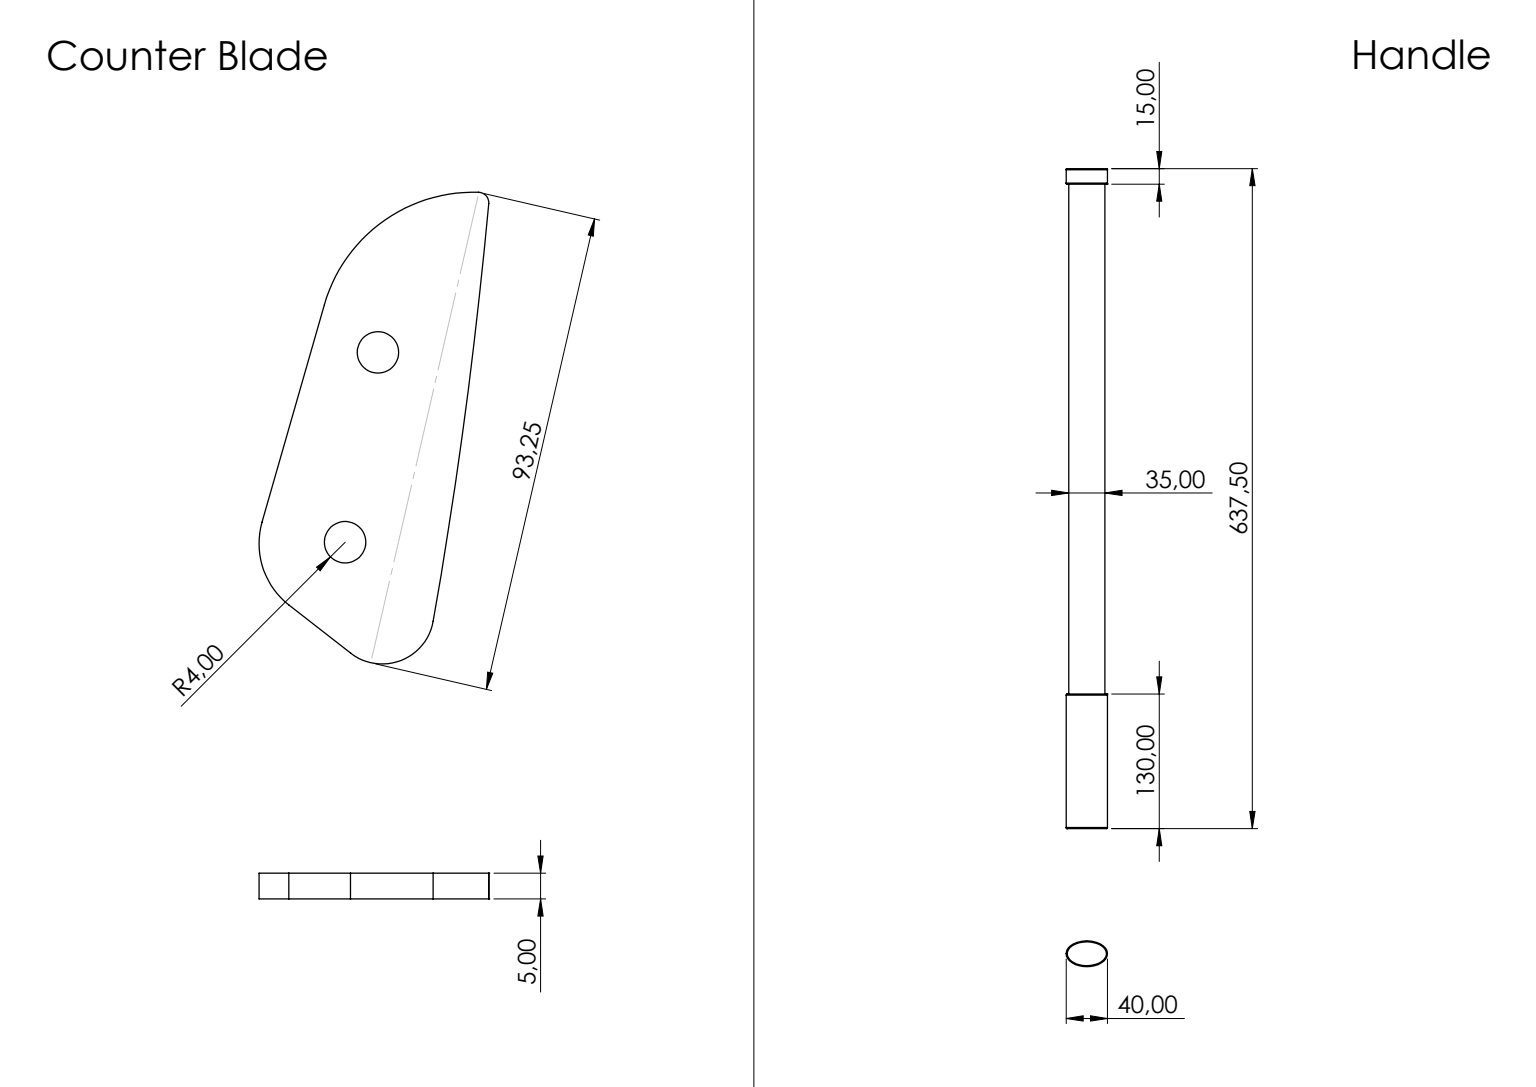
ISO-10303-21;
HEADER;
FILE_DESCRIPTION (('STEP AP214'),
    '1' );
FILE_NAME ('Handle.step',
    '2026-10-06T08:24:18',
    ( '' ),
    ( '' ),
    'SwSTEP 2.0',
    'SolidWorks 2020',
    '' );
FILE_SCHEMA (( 'AUTOMOTIVE_DESIGN' ));
ENDSEC;

DATA;
#4=CARTESIAN_POINT ( 'NONE',  ( 15.24035984457677628, 4.192874667847209302, 315.0000000000000000 ) ) ;
#5=CARTESIAN_POINT ( 'NONE',  ( 9.254661647337838914, -11.09380704494734360, -303.4999999999996589 ) ) ;
#6=CARTESIAN_POINT ( 'NONE',  ( 16.58659719219999928, 2.947707964209000053, -314.6383426456000052 ) ) ;
#11=CARTESIAN_POINT ( 'NONE',  ( 14.97796429264999141, 8.396158284077998246, -317.0792622552969533 ) ) ;
#15=CARTESIAN_POINT ( 'NONE',  ( 4.345375235838000449, -11.20786428128000090, 320.0000000000000000 ) ) ;
#19=CARTESIAN_POINT ( 'NONE',  ( 12.11078853722071180, -6.646648371397081867, -315.0000000000000000 ) ) ;
#22=VERTEX_POINT ( 'NONE', #5856 ) ;
#23=CARTESIAN_POINT ( 'NONE',  ( -16.90341843474000072, 5.241942252742000541, -317.4999999999989768 ) ) ;
#26=CARTESIAN_POINT ( 'NONE',  ( -6.686361683900003072, -11.78513185998999546, -303.6197174156509391 ) ) ;
#28=CARTESIAN_POINT ( 'NONE',  ( 9.022589772749004311, -9.990182113135000819, -317.4928077629770087 ) ) ;
#29=CARTESIAN_POINT ( 'NONE',  ( 10.00000000000000000, 2.500000000000000000, -317.5000000000000000 ) ) ;
#30=EDGE_CURVE ( 'NONE', #1105, #135, #3775, .T. ) ;
#31=CARTESIAN_POINT ( 'NONE',  ( -18.56223039349998771, 4.700611568415998143, -303.6197174156520759 ) ) ;
#32=CARTESIAN_POINT ( 'NONE',  ( -17.50000003227012613, 5.857864393370423528, 314.9999999999999432 ) ) ;
#40=CARTESIAN_POINT ( 'NONE',  ( 16.39637408479998726, -7.274214857915000998, 190.4207385301700128 ) ) ;
#42=CARTESIAN_POINT ( 'NONE',  ( 16.31080841943641602, 2.657385524587721370, -314.9999999999999432 ) ) ;
#45=CARTESIAN_POINT ( 'NONE',  ( 17.36938240862999905, -0.02134527931159000205, 314.6383426456000052 ) ) ;
#50=CARTESIAN_POINT ( 'NONE',  ( 15.30440697208000600, -7.531500302410004011, 320.0770942683900557 ) ) ;
#52=CARTESIAN_POINT ( 'NONE',  ( -19.86889125890001395, 1.746333262808030584, -303.4999999999990905 ) ) ;
#53=CARTESIAN_POINT ( 'NONE',  ( 15.71297435277999810, 3.490404421959999670, 315.0848619657999734 ) ) ;
#55=CARTESIAN_POINT ( 'NONE',  ( 12.16184652991773163, -9.933083713569276441, 190.9999999999995737 ) ) ;
#61=CARTESIAN_POINT ( 'NONE',  ( 15.00000000000000000, 0.000000000000000000, -285.0000000000000000 ) ) ;
#67=ORIENTED_EDGE ( 'NONE', *, *, #7702, .T. ) ;
#68=CARTESIAN_POINT ( 'NONE',  ( -16.87780931964001141, 6.722286650069999148, -316.3802825947000201 ) ) ;
#70=CARTESIAN_POINT ( 'NONE',  ( -13.47907531561000027, -8.083075672345000129, 320.0000000000000000 ) ) ;
#72=DIRECTION ( 'NONE',  ( 2.134661487851416834E-05, 5.799867324353239268E-11, -0.9999999997721611411 ) ) ;
#73=CARTESIAN_POINT ( 'NONE',  ( 2.450863364448387038, -9.399909383054028567, -315.0000000000000000 ) ) ;
#76=CARTESIAN_POINT ( 'NONE',  ( 4.551150791544315233, -9.653623619670588241, -314.5171481538503144 ) ) ;
#79=CARTESIAN_POINT ( 'NONE',  ( 14.32993508528999982, 7.533629911342000440, -317.5000000000000000 ) ) ;
#80=EDGE_LOOP ( 'NONE', ( #2760, #368 ) ) ;
#82=CARTESIAN_POINT ( 'NONE',  ( -17.70828763765000247, -5.833668797872996414, -303.6197174156520759 ) ) ;
#83=CLOSED_SHELL ( 'NONE', ( #10215, #9940, #6869, #5277, #4807 ) ) ;
#84=CARTESIAN_POINT ( 'NONE',  ( 3.630810623869999976, -11.17897874952999793, -317.4928077629770087 ) ) ;
#92=CARTESIAN_POINT ( 'NONE',  ( -10.00000000000000000, 2.500000000000000000, -315.0000000000000000 ) ) ;
#95=CARTESIAN_POINT ( 'NONE',  ( 18.68134283559999531, -4.475435185431997809, 191.1197171614399792 ) ) ;
#99=CARTESIAN_POINT ( 'NONE',  ( -7.781240562249999826, 11.51887802030999985, 191.1197171614399792 ) ) ;
#100=ORIENTED_CLOSED_SHELL ( 'NONE', *, #3850, .F. );
#105=CARTESIAN_POINT ( 'NONE',  ( 18.85102544288001170, -0.8044398135754999846, 319.9928079742500131 ) ) ;
#106=CARTESIAN_POINT ( 'NONE',  ( -9.994972990543319113, 8.217268623422803842, 314.4999428952269227 ) ) ;
#107=CARTESIAN_POINT ( 'NONE',  ( 8.519003879469000395, 8.390442916014999142, 314.8616023057000461 ) ) ;
#109=CARTESIAN_POINT ( 'NONE',  ( 7.783073706837757122, -11.52583533951409756, 190.9999999999995737 ) ) ;
#116=CARTESIAN_POINT ( 'NONE',  ( -3.309867371927075919, 9.320876041153052682, 315.0000000000000568 ) ) ;
#118=EDGE_LOOP ( 'NONE', ( #3514, #10461 ) ) ;
#123=CARTESIAN_POINT ( 'NONE',  ( 0.000000000000000000, 7.937240849781000307, 315.0000000000001705 ) ) ;
#125=CARTESIAN_POINT ( 'NONE',  ( 1.606003227921999343, 12.55439432250999587, -317.0792622552969533 ) ) ;
#130=CARTESIAN_POINT ( 'NONE',  ( 16.45380452100018331, -2.370995337294541372, -315.0000000000000000 ) ) ;
#133=ORIENTED_EDGE ( 'NONE', *, *, #10090, .F. ) ;
#135=VERTEX_POINT ( 'NONE', #4262 ) ;
#136=CARTESIAN_POINT ( 'NONE',  ( 3.426853146664001759, -12.32346385046998627, -303.6197174156509391 ) ) ;
#137=CARTESIAN_POINT ( 'NONE',  ( -10.06352840551000050, -9.619263554820991047, -317.4928077629770087 ) ) ;
#139=CARTESIAN_POINT ( 'NONE',  ( -16.90798586812000082, -0.2930809059028999797, -315.0848619657999734 ) ) ;
#141=CARTESIAN_POINT ( 'NONE',  ( -5.044863629634003921, 12.10215170741999557, -303.6197174156520759 ) ) ;
#142=CARTESIAN_POINT ( 'NONE',  ( -15.42236150774597903, -4.758481132285194981, 314.4999482133869719 ) ) ;
#143=EDGE_LOOP ( 'NONE', ( #5687, #4056 ) ) ;
#145=CARTESIAN_POINT ( 'NONE',  ( -12.36246450207000080, 8.718211867489999989, -302.5000000000000000 ) ) ;
#147=CARTESIAN_POINT ( 'NONE',  ( 17.61637523988000353, -5.923742513492005202, 191.1197171614399792 ) ) ;
#148=CARTESIAN_POINT ( 'NONE',  ( -12.98706127646999953, -6.788989183774999603, -315.0000000000001137 ) ) ;
#149=CARTESIAN_POINT ( 'NONE',  ( 15.88699210612483803, 3.373196549223925533, -315.0000000000000000 ) ) ;
#151=CARTESIAN_POINT ( 'NONE',  ( 13.05089818882000507, 9.570190452814999915, 190.4207385301700128 ) ) ;
#153=CARTESIAN_POINT ( 'NONE',  ( 17.12432750374000179, 0.4000877216259000058, 314.8616023057000461 ) ) ;
#155=CARTESIAN_POINT ( 'NONE',  ( -18.77022956583000735, -3.456581952569002247, 320.0770942683900557 ) ) ;
#156=CARTESIAN_POINT ( 'NONE',  ( -17.50000000000000000, 1.896400240175167841E-08, 314.4999014931028682 ) ) ;
#157=CARTESIAN_POINT ( 'NONE',  ( -19.99979308783253273, 0.5741528085765136291, -303.4999999999998863 ) ) ;
#159=CARTESIAN_POINT ( 'NONE',  ( 14.38384290288000145, 5.252906928686999599, 314.8616023057000461 ) ) ;
#161=CARTESIAN_POINT ( 'NONE',  ( 10.13048420337591615, -10.78707197045944355, 190.9999999999995737 ) ) ;
#163=CARTESIAN_POINT ( 'NONE',  ( -0.6354225718825003977, 12.59144946217000260, 319.5792614743400009 ) ) ;
#166=CARTESIAN_POINT ( 'NONE',  ( -12.75139817577315604, 6.274227700150676768, 315.0000000000000568 ) ) ;
#175=CARTESIAN_POINT ( 'NONE',  ( 11.05300996161902560, -7.762248705067454679, 314.4999426419801694 ) ) ;
#183=CARTESIAN_POINT ( 'NONE',  ( 17.50000000000000000, 0.000000000000000000, -315.0000000000000000 ) ) ;
#185=CARTESIAN_POINT ( 'NONE',  ( 4.714169693051698751, -9.123832451407690058, -315.0000000000000000 ) ) ;
#188=CARTESIAN_POINT ( 'NONE',  ( 13.93637444108895096, -8.981144148067276234, -316.5000000000004547 ) ) ;
#189=VERTEX_POINT ( 'NONE', #1946 ) ;
#190=CARTESIAN_POINT ( 'NONE',  ( -5.180828043054999554, 11.07085478567999992, -317.5000000000000000 ) ) ;
#192=CARTESIAN_POINT ( 'NONE',  ( -5.254364691879999327, -12.06635523715000424, -303.6197174156520759 ) ) ;
#193=CARTESIAN_POINT ( 'NONE',  ( 10.19016500772999656, -9.569509725303996461, -317.4928077629770087 ) ) ;
#196=CARTESIAN_POINT ( 'NONE',  ( -3.426853146664001759, 12.32346385046998627, -303.6197174156509391 ) ) ;
#197=ADVANCED_FACE ( 'NONE', ( #5213 ), #3671, .T. ) ;
#200=CARTESIAN_POINT ( 'NONE',  ( -17.12450099635000100, 0.4005340032738999856, -314.8616023057000461 ) ) ;
#201=CARTESIAN_POINT ( 'NONE',  ( -19.00000000000000000, 0.000000000000000000, -302.5000000001010108 ) ) ;
#203=CARTESIAN_POINT ( 'NONE',  ( -20.05695074155000768, 0.5616361869863997214, 190.4207385301700128 ) ) ;
#205=CARTESIAN_POINT ( 'NONE',  ( 13.92525118639320425, 5.424153755683056133, -315.0000000000000000 ) ) ;
#206=CARTESIAN_POINT ( 'NONE',  ( 18.77789454208001985, 4.479159834667000517, 190.4207385301700128 ) ) ;
#207=CARTESIAN_POINT ( 'NONE',  ( 15.60185585328000002, -4.689707898928999974, 314.4150829855000211 ) ) ;
#210=CARTESIAN_POINT ( 'NONE',  ( 4.335116381453002710, -11.79481621787999757, 320.0770942683900557 ) ) ;
#212=CARTESIAN_POINT ( 'NONE',  ( -5.453155018295565704, 9.512440914238338152, 314.4999437815906731 ) ) ;
#213=CARTESIAN_POINT ( 'NONE',  ( -19.32402384659099326, 3.348155292981251030, -303.4999999999990905 ) ) ;
#214=CARTESIAN_POINT ( 'NONE',  ( 12.10743226551000085, 7.094093637544000686, 314.6383426456000052 ) ) ;
#217=CARTESIAN_POINT ( 'NONE',  ( 4.941041030666997180, 12.20591504665998350, 319.5792614743400009 ) ) ;
#220=CARTESIAN_POINT ( 'NONE',  ( -7.529172669043764365, 8.513076715957524243, 315.0000000000000000 ) ) ;
#227=CARTESIAN_POINT ( 'NONE',  ( -6.280550016735999996, 10.85821747223999978, 190.0000000000000000 ) ) ;
#228=CARTESIAN_POINT ( 'NONE',  ( 17.49966312145292591, -0.4461383165315541688, 314.4999388432775049 ) ) ;
#231=CARTESIAN_POINT ( 'NONE',  ( 10.60393767981000757, 9.400660304482000740, 190.0071920248299477 ) ) ;
#239=CARTESIAN_POINT ( 'NONE',  ( -8.616488358140818704, -8.177789738293625987, -315.0000000000000000 ) ) ;
#242=CARTESIAN_POINT ( 'NONE',  ( -13.89291764776418603, -9.007512922136868383, -316.5000000000004547 ) ) ;
#245=VERTEX_POINT ( 'NONE', #4539 ) ;
#246=CARTESIAN_POINT ( 'NONE',  ( -17.62591998684001027, 4.093640041088997705, -317.4928077629770087 ) ) ;
#247=CARTESIAN_POINT ( 'NONE',  ( 19.46922894822000316, -1.611824300579999925, -317.5770954168139610 ) ) ;
#249=CARTESIAN_POINT ( 'NONE',  ( -16.41165915566000066, 2.800979832323999830, -314.8616023057000461 ) ) ;
#258=CARTESIAN_POINT ( 'NONE',  ( -7.580171359958006505, -11.65906041016999062, 190.4207385301700128 ) ) ;
#260=CARTESIAN_POINT ( 'NONE',  ( 16.10169247195999631, -5.923112460043001626, -302.5071922382879279 ) ) ;
#261=CARTESIAN_POINT ( 'NONE',  ( -15.61478958302000208, 7.813810907915007320, 191.1197171614399792 ) ) ;
#263=CARTESIAN_POINT ( 'NONE',  ( 13.50042001888999899, -6.225262767767000049, 314.6383426456000052 ) ) ;
#264=DIRECTION ( 'NONE',  ( -1.023612789531999991E-09, -6.047396539087999167E-11, 1.000000000000000000 ) ) ;
#265=CARTESIAN_POINT ( 'NONE',  ( 2.578726422179000721, -12.49238522902999726, 319.5792614743400009 ) ) ;
#267=CARTESIAN_POINT ( 'NONE',  ( -16.88587703871184686, 6.724495681871323960, -303.4999999999990905 ) ) ;
#268=CARTESIAN_POINT ( 'NONE',  ( 16.95904175860000151, 2.156867278632000229, 314.6383426456000052 ) ) ;
#270=CARTESIAN_POINT ( 'NONE',  ( 13.10504385913262482, -9.452822371482909602, 190.9999999999995737 ) ) ;
#271=CARTESIAN_POINT ( 'NONE',  ( 6.490016473005998598, 11.91548699335000272, 319.5792614743400009 ) ) ;
#272=DIRECTION ( 'NONE',  ( 5.580921735165581358E-06, -2.007400791704409772E-12, 0.9999999999844266796 ) ) ;
#273=CARTESIAN_POINT ( 'NONE',  ( 4.934712326437797003, 9.087261561615623151, 315.0000000000000000 ) ) ;
#277=CARTESIAN_POINT ( 'NONE',  ( 2.585384220735000405, 11.41066401029999966, 190.0000000000000000 ) ) ;
#278=CARTESIAN_POINT ( 'NONE',  ( -14.02804746531204749, 5.341076607092833051, -315.0000000000000000 ) ) ;
#284=LINE ( 'NONE', #8342, #7202 ) ;
#288=CARTESIAN_POINT ( 'NONE',  ( 5.323201728285183343, -12.06184864676790447, -316.5000000000004547 ) ) ;
#291=ORIENTED_EDGE ( 'NONE', *, *, #4224, .T. ) ;
#292=DIRECTION ( 'NONE',  ( -2.558226603731915840E-07, 0.9999999999999674705, 3.930810334569221757E-22 ) ) ;
#294=CARTESIAN_POINT ( 'NONE',  ( -19.60172830838999047, -0.3498260303709999630, -317.5770954168139610 ) ) ;
#296=CARTESIAN_POINT ( 'NONE',  ( -17.56758064089999749, 0.6313722887073000001, -314.4150829855000211 ) ) ;
#297=( BOUNDED_CURVE ( )  B_SPLINE_CURVE ( 3, ( #701, #648, #8167, #4939 ),
 .UNSPECIFIED., .F., .F. ) 
 B_SPLINE_CURVE_WITH_KNOTS ( ( 4, 4 ),
 ( 0.000000000000000000, 0.9999999989866708017 ),
 .UNSPECIFIED. ) 
 CURVE ( )  GEOMETRIC_REPRESENTATION_ITEM ( )  RATIONAL_B_SPLINE_CURVE ( ( 1.000000000000000000, 0.8029010327867776020, 0.8003084355100938962, 0.9922222081699485496 ) ) 
 REPRESENTATION_ITEM ( '' )  );
#299=CARTESIAN_POINT ( 'NONE',  ( 17.59656075795390606, 5.807225057570236437, 315.0000000000000000 ) ) ;
#300=ORIENTED_EDGE ( 'NONE', *, *, #1909, .T. ) ;
#301=CARTESIAN_POINT ( 'NONE',  ( -17.35547125580999861, -4.661453509011000307, 190.0000000000000000 ) ) ;
#307=CARTESIAN_POINT ( 'NONE',  ( -10.00000000000000000, 2.500000000000000000, -285.0000000000000000 ) ) ;
#310=CARTESIAN_POINT ( 'NONE',  ( 7.580171359958006505, 11.65906041016999062, 190.4207385301700128 ) ) ;
#314=CARTESIAN_POINT ( 'NONE',  ( -18.87180507196998747, -0.3567823988189002815, -302.5071922382879279 ) ) ;
#315=CARTESIAN_POINT ( 'NONE',  ( -19.98292278601002181, 0.4165571180016003350, 318.8802828394900644 ) ) ;
#317=CARTESIAN_POINT ( 'NONE',  ( 17.13090252310000139, 0.3058267005333999977, -314.8616023057000461 ) ) ;
#319=CARTESIAN_POINT ( 'NONE',  ( -14.57772014836000096, 5.380605385836000565, 314.6383426456000052 ) ) ;
#321=CARTESIAN_POINT ( 'NONE',  ( 14.19899178590998190, -7.472503199908998361, 190.0071920248299477 ) ) ;
#323=CARTESIAN_POINT ( 'NONE',  ( 1.330908921489000418, 12.56946842516999041, 319.5792614743400009 ) ) ;
#325=CARTESIAN_POINT ( 'NONE',  ( 9.142607798242581296, 7.997258514545670494, 315.0000000000000000 ) ) ;
#330=CARTESIAN_POINT ( 'NONE',  ( 13.37693598625000213, 8.145668871592000926, 190.0000000000000000 ) ) ;
#331=CARTESIAN_POINT ( 'NONE',  ( 13.64750606492133045, -6.290789845814279246, 314.4999418822395114 ) ) ;
#332=CARTESIAN_POINT ( 'NONE',  ( -15.60334176867001688, 6.376785739494004623, 190.0071920248299477 ) ) ;
#337=CARTESIAN_POINT ( 'NONE',  ( 14.25090727152774228, -5.161646102170217354, 315.0000000000000568 ) ) ;
#340=CARTESIAN_POINT ( 'NONE',  ( 3.092734256763002065, 11.24153629139000188, 319.9928079742500131 ) ) ;
#341=CARTESIAN_POINT ( 'NONE',  ( -16.85039254115126539, -6.759165854037040511, -316.5000000000004547 ) ) ;
#347=CARTESIAN_POINT ( 'NONE',  ( -14.69255688194000520, -7.987735679832996816, -317.5770954168139610 ) ) ;
#348=CARTESIAN_POINT ( 'NONE',  ( -15.92197846796999983, 3.582977715798000062, -314.8616023057000461 ) ) ;
#349=CARTESIAN_POINT ( 'NONE',  ( 17.27223423031419358, 1.573973318776797026, -314.5135302205612220 ) ) ;
#350=ORIENTED_EDGE ( 'NONE', *, *, #8269, .F. ) ;
#361=ADVANCED_FACE ( 'NONE', ( #10562 ), #4708, .F. ) ;
#364=FACE_OUTER_BOUND ( 'NONE', #2969, .T. ) ;
#365=CARTESIAN_POINT ( 'NONE',  ( 19.56939737065003015, -2.860667089442002986, 319.5792614743400009 ) ) ;
#367=CARTESIAN_POINT ( 'NONE',  ( -14.43094748301999886, 5.211771040651000497, 314.8616023057000461 ) ) ;
#368=ORIENTED_EDGE ( 'NONE', *, *, #5471, .T. ) ;
#370=ORIENTED_EDGE ( 'NONE', *, *, #7787, .T. ) ;
#371=CARTESIAN_POINT ( 'NONE',  ( -17.61140045117998554, 5.929979699424000827, 318.8802828394900644 ) ) ;
#374=CARTESIAN_POINT ( 'NONE',  ( -17.13182678275000370, 0.2945984483948000388, 314.8616023057000461 ) ) ;
#375=CARTESIAN_POINT ( 'NONE',  ( -15.88661950543927404, 3.373766516133892335, 315.0000000000000000 ) ) ;
#383=CARTESIAN_POINT ( 'NONE',  ( -8.676965067697993916, 10.10010313590999509, 190.0071920248299477 ) ) ;
#387=CARTESIAN_POINT ( 'NONE',  ( 8.517242506840645433, -8.210459489885888473, 315.0000000000000568 ) ) ;
#388=CARTESIAN_POINT ( 'NONE',  ( 11.99990625867999938, 6.898016740823000426, -314.8616023057000461 ) ) ;
#391=CARTESIAN_POINT ( 'NONE',  ( 10.79243608611000305, 9.321647281761997306, 319.9928079742500131 ) ) ;
#395=CARTESIAN_POINT ( 'NONE',  ( -15.97383562432999149, -7.643564190274003245, -317.0792622552969533 ) ) ;
#399=CARTESIAN_POINT ( 'NONE',  ( 12.62255196312000116, -8.576358104672999971, 190.0000000000000000 ) ) ;
#402=CARTESIAN_POINT ( 'NONE',  ( -15.59929043073998578, -7.826471063572999931, 191.1197171614399792 ) ) ;
#405=CARTESIAN_POINT ( 'NONE',  ( -1.914578617915998704, -11.33709939001001032, -302.5071922382879279 ) ) ;
#411=CARTESIAN_POINT ( 'NONE',  ( -13.35956122709998795, 8.020600178289003068, -302.5071922382879279 ) ) ;
#412=CARTESIAN_POINT ( 'NONE',  ( -19.58476356052999279, -2.818858455686998887, 319.5792614743400009 ) ) ;
#413=CARTESIAN_POINT ( 'NONE',  ( 16.99702983282000091, -1.298346578676000007, -314.8616023057000461 ) ) ;
#414=AXIS2_PLACEMENT_3D ( 'NONE', #9424, #292, #2763 ) ;
#415=CARTESIAN_POINT ( 'NONE',  ( -12.17979804859000126, 7.053762231097000068, 314.6383426456000052 ) ) ;
#417=CARTESIAN_POINT ( 'NONE',  ( -9.595833218033995138, -9.789665514059997520, 190.0071920248299477 ) ) ;
#423=CARTESIAN_POINT ( 'NONE',  ( -17.35477687787999912, 0.3068793820639000303, 314.6383426456000052 ) ) ;
#424=CARTESIAN_POINT ( 'NONE',  ( -16.34899991413091414, 2.583752171356570759, 315.0000000000000000 ) ) ;
#427=AXIS2_PLACEMENT_3D ( 'NONE', #92, #1648, #838 ) ;
#428=CARTESIAN_POINT ( 'NONE',  ( -16.31080841943642312, -2.657385524587722703, -315.0000000000001137 ) ) ;
#431=CARTESIAN_POINT ( 'NONE',  ( 11.71572875054933327, 12.50000000135959688, -303.5000000000000000 ) ) ;
#433=CARTESIAN_POINT ( 'NONE',  ( 8.586696445213114259, 8.187646113561793726, -314.9999999999999432 ) ) ;
#434=CARTESIAN_POINT ( 'NONE',  ( 17.75414941409001557, 3.856242593410000197, 190.0071920248299477 ) ) ;
#436=CARTESIAN_POINT ( 'NONE',  ( 17.50000000000000711, -8.653864165198663120E-10, -302.4999999999999432 ) ) ;
#439=CARTESIAN_POINT ( 'NONE',  ( -11.26076953950000004, -9.251451169536998975, -317.5000000000000000 ) ) ;
#442=CARTESIAN_POINT ( 'NONE',  ( 2.737672117484407863, -9.377292971636139285, 315.0000000000000568 ) ) ;
#443=CARTESIAN_POINT ( 'NONE',  ( 13.18712987686000027, 5.898505050745000311, -315.0848619657999734 ) ) ;
#445=CARTESIAN_POINT ( 'NONE',  ( 18.45919443845001950, 2.405475664342000996, 319.9928079742500131 ) ) ;
#448=ORIENTED_EDGE ( 'NONE', *, *, #9438, .T. ) ;
#450=CARTESIAN_POINT ( 'NONE',  ( 19.39427072114999717, -3.381181012882998882, -317.0792622552969533 ) ) ;
#452=B_SPLINE_CURVE_WITH_KNOTS ( 'NONE', 3,
 ( #9871, #3367, #5940, #9919, #5772, #2557, #9228, #142, #5825, #942, #10323, #1912, #8408, #5184, #1349, #10377, #4385, #5129, #7659, #8654, #4578, #3528 ),
 .UNSPECIFIED., .F., .F.,
 ( 4, 2, 2, 2, 2, 2, 2, 2, 2, 2, 4 ),
 ( 0.000000000000000000, 0.06249979490446620767, 0.1249995898089324153, 0.1874993847133986091, 0.2499991796178648307, 0.3124989745223310522, 0.3437488719745641630, 0.3749987694267972183, 0.4062486668790303290, 0.4374985643312634398, 0.4999983592357296613 ),
 .UNSPECIFIED. ) ;
#453=ADVANCED_BREP_SHAPE_REPRESENTATION ( '', ( #5170, #2817 ), #8168 ) ;
#455=ORIENTED_EDGE ( 'NONE', *, *, #1550, .F. ) ;
#456=CARTESIAN_POINT ( 'NONE',  ( -14.18540515794000001, -7.627402598852000004, 190.0000000000000000 ) ) ;
#458=ORIENTED_EDGE ( 'NONE', *, *, #4238, .T. ) ;
#459=CARTESIAN_POINT ( 'NONE',  ( 10.12800840543000724, -10.78031690431999756, 191.1197171614399792 ) ) ;
#461=CARTESIAN_POINT ( 'NONE',  ( -16.68818136459866253, -1.819152193222137281, 315.0000000000000000 ) ) ;
#462=CARTESIAN_POINT ( 'NONE',  ( 13.35956122709998795, -8.020600178289003068, -302.5071922382879279 ) ) ;
#466=CARTESIAN_POINT ( 'NONE',  ( 6.445894847559003438, 10.69844988487999693, -302.5071922382879279 ) ) ;
#468=CARTESIAN_POINT ( 'NONE',  ( -16.43550475785002263, -7.239471399781003846, 319.5792614743400009 ) ) ;
#469=CARTESIAN_POINT ( 'NONE',  ( 15.92197846796999983, -3.582977715798000062, -314.8616023057000461 ) ) ;
#470=CARTESIAN_POINT ( 'NONE',  ( -13.62823431091000081, 6.408810695481999886, 314.4150829855000211 ) ) ;
#472=CARTESIAN_POINT ( 'NONE',  ( 17.73236801841998300, -3.892024484092002634, 190.0071920248299477 ) ) ;
#482=CARTESIAN_POINT ( 'NONE',  ( -16.61594764501906596, 2.013242305049250280, 315.0000000000001137 ) ) ;
#484=CARTESIAN_POINT ( 'NONE',  ( -10.90988923471838667, -7.272053090123304031, -315.0000000000000568 ) ) ;
#487=CARTESIAN_POINT ( 'NONE',  ( 17.50000000088855501, 5.867334121986936601, -302.4999999999996589 ) ) ;
#488=CARTESIAN_POINT ( 'NONE',  ( 0.9838506439437809670, 9.488399989288442526, -314.9999999999998863 ) ) ;
#489=CARTESIAN_POINT ( 'NONE',  ( -19.54676335584001023, 0.8901129224502002391, 189.9229057364800042 ) ) ;
#490=CARTESIAN_POINT ( 'NONE',  ( 11.54127216423516877, 7.525448809341461320, 314.4999468205385824 ) ) ;
#496=CARTESIAN_POINT ( 'NONE',  ( 9.217211940708146756, -7.977736869146946574, 315.0000000000000000 ) ) ;
#497=CARTESIAN_POINT ( 'NONE',  ( -8.551447359560999217, 8.144527334518999240, -315.0848619657999734 ) ) ;
#499=CARTESIAN_POINT ( 'NONE',  ( -18.12318599310000167, 3.186119256560000945, 319.9928079742500131 ) ) ;
#503=CARTESIAN_POINT ( 'NONE',  ( -18.21319838702001448, 4.476589323548002319, -317.5770954168139610 ) ) ;
#504=CARTESIAN_POINT ( 'NONE',  ( -11.69962851017000283, -10.23591410519999201, -317.0792622552969533 ) ) ;
#508=CARTESIAN_POINT ( 'NONE',  ( -17.50000000000000000, 0.000000000000000000, -315.0000000000000000 ) ) ;
#510=CARTESIAN_POINT ( 'NONE',  ( -12.62255196312000116, 8.576358104672999971, 190.0000000000000000 ) ) ;
#513=DIRECTION ( 'NONE',  ( 0.000000000000000000, 0.000000000000000000, 1.000000000000000000 ) ) ;
#515=CARTESIAN_POINT ( 'NONE',  ( -19.78498824058000594, -1.878712957033002340, 191.1197171614399792 ) ) ;
#518=CARTESIAN_POINT ( 'NONE',  ( 10.36918760129999484, -10.25095399663999451, -302.4229045757450081 ) ) ;
#523=CARTESIAN_POINT ( 'NONE',  ( -6.297776810737998332, 10.73166643879000404, -302.5071922382879279 ) ) ;
#525=CARTESIAN_POINT ( 'NONE',  ( -17.14577796628000073, 0.02050488658304999712, 314.8616023057000461 ) ) ;
#528=CARTESIAN_POINT ( 'NONE',  ( -16.98888588455999127, 6.600739700975996271, 318.8802828394900644 ) ) ;
#530=DIRECTION ( 'NONE',  ( 0.000000000000000000, 0.000000000000000000, 1.000000000000000000 ) ) ;
#534=CARTESIAN_POINT ( 'NONE',  ( 11.28781796570999951, -4.951468039558000633, 315.0000000000001705 ) ) ;
#535=CARTESIAN_POINT ( 'NONE',  ( -13.94567317170587017, -5.407789506212602682, -314.9999999999999432 ) ) ;
#538=CARTESIAN_POINT ( 'NONE',  ( -10.23467949692583190, 10.00000000050611959, -302.5000000000002842 ) ) ;
#539=CARTESIAN_POINT ( 'NONE',  ( 8.377487131979357571, 8.255758461348163380, -315.0000000000000000 ) ) ;
#540=CARTESIAN_POINT ( 'NONE',  ( -20.05687582562997662, -0.5621360437329007143, 190.4207385301700128 ) ) ;
#542=CARTESIAN_POINT ( 'NONE',  ( 9.038557733644999814, -10.11114377999000169, -317.5000000000000000 ) ) ;
#545=CARTESIAN_POINT ( 'NONE',  ( 13.92506561308973545, -5.424300063451886089, 315.0000000000000568 ) ) ;
#546=CARTESIAN_POINT ( 'NONE',  ( -6.488017178959999853, 9.182784307579000327, -314.6383426456000052 ) ) ;
#547=FACE_OUTER_BOUND ( 'NONE', #6635, .T. ) ;
#548=CARTESIAN_POINT ( 'NONE',  ( 17.87038977196999312, 4.940238929760003117, 320.0770942683900557 ) ) ;
#552=CARTESIAN_POINT ( 'NONE',  ( -20.10152810630999554, 0.3450717431897997733, -317.0792622552969533 ) ) ;
#553=CARTESIAN_POINT ( 'NONE',  ( -7.863726017345004315, -11.49810175465000661, -316.3802825947000201 ) ) ;
#558=CARTESIAN_POINT ( 'NONE',  ( -4.551150791544325003, 9.653623619670586464, -314.5171481538502576 ) ) ;
#561=CARTESIAN_POINT ( 'NONE',  ( -17.80781204382000027, 3.997739559166000323, 190.0000000000000000 ) ) ;
#562=CARTESIAN_POINT ( 'NONE',  ( 15.56166711177641204, -7.864757419948091410, 319.0000000000003979 ) ) ;
#563=VERTEX_POINT ( 'NONE', #7338 ) ;
#566=CARTESIAN_POINT ( 'NONE',  ( -4.780298404687055580, -9.113031460416761931, 315.0000000000000000 ) ) ;
#567=CARTESIAN_POINT ( 'NONE',  ( -16.90094380520001849, -6.817658119454999444, -302.9207377450070453 ) ) ;
#572=CARTESIAN_POINT ( 'NONE',  ( -9.124390749379998056, 10.69353917616999539, -302.4229045757450081 ) ) ;
#573=CARTESIAN_POINT ( 'NONE',  ( 17.61140045117998554, -5.929979699424000827, 318.8802828394900644 ) ) ;
#575=CARTESIAN_POINT ( 'NONE',  ( -13.56771446467999986, -6.451120369226999607, -314.4150829855000211 ) ) ;
#576=LINE ( 'NONE', #10569, #3520 ) ;
#577=ORIENTED_EDGE ( 'NONE', *, *, #8567, .T. ) ;
#578=CARTESIAN_POINT ( 'NONE',  ( -0.7033324871772000941, -12.09174782753000166, 189.9229057364800042 ) ) ;
#579=CARTESIAN_POINT ( 'NONE',  ( -19.77468550638000266, 1.920668048511998904, 318.8802828394900644 ) ) ;
#584=CARTESIAN_POINT ( 'NONE',  ( -13.31399140613000043, -6.082710156904999721, 314.8616023057000461 ) ) ;
#586=CARTESIAN_POINT ( 'NONE',  ( -13.82226565756009684, 5.505830577453552088, 315.0000000000000568 ) ) ;
#587=FACE_OUTER_BOUND ( 'NONE', #4840, .T. ) ;
#589=CARTESIAN_POINT ( 'NONE',  ( -3.970004819630974957, -9.235895690467337715, -315.0000000000000568 ) ) ;
#590=CARTESIAN_POINT ( 'NONE',  ( 19.99999035944999903, -7.277437094418000096E-10, -303.5000000000000000 ) ) ;
#591=CARTESIAN_POINT ( 'NONE',  ( -11.28781796570999951, 4.951468039558000633, 315.0000000000000000 ) ) ;
#596=CARTESIAN_POINT ( 'NONE',  ( -4.780493465650554441, 9.113006550021843566, -314.9999999999999432 ) ) ;
#598=CARTESIAN_POINT ( 'NONE',  ( 16.06942734036999454, 6.898991720969999797, 189.9229057364800042 ) ) ;
#599=CARTESIAN_POINT ( 'NONE',  ( 17.50000000088856567, 5.867334121986925055, 190.0000000000002558 ) ) ;
#600=CARTESIAN_POINT ( 'NONE',  ( -17.62191473184000046, -4.312542294520999242, -317.5000000000030127 ) ) ;
#604=FACE_BOUND ( 'NONE', #4756, .T. ) ;
#607=CARTESIAN_POINT ( 'NONE',  ( 17.57772697299999720, -0.3191603157329999663, -314.4150829855000211 ) ) ;
#609=CARTESIAN_POINT ( 'NONE',  ( -11.81011838702999484, 9.634252844421009598, 320.0770942683900557 ) ) ;
#613=CARTESIAN_POINT ( 'NONE',  ( -19.56985579239002959, -0.3946094453810997660, -317.5770954168139610 ) ) ;
#614=CARTESIAN_POINT ( 'NONE',  ( 11.75551710966999153, -10.11738730586000123, -316.3802825947000201 ) ) ;
#619=CARTESIAN_POINT ( 'NONE',  ( 19.99999721132999753, -3.518697978483000342E-10, 319.0000000000000000 ) ) ;
#623=CARTESIAN_POINT ( 'NONE',  ( -15.47214269673303200, -3.911151857093433382, 315.0000000000000568 ) ) ;
#624=CARTESIAN_POINT ( 'NONE',  ( -19.95002954278003315, -1.762942793154997911, -302.9207377450070453 ) ) ;
#625=CARTESIAN_POINT ( 'NONE',  ( 10.00000000000000000, 2.500000000000000000, -315.0000000000000000 ) ) ;
#627=ADVANCED_FACE ( 'NONE', ( #9915 ), #6187, .T. ) ;
#628=CARTESIAN_POINT ( 'NONE',  ( 5.268482393219001025, 12.14948647186998976, -302.9207377450070453 ) ) ;
#631=CARTESIAN_POINT ( 'NONE',  ( 10.58688533405000065, -7.844683714540999553, -314.6383426456000052 ) ) ;
#632=CARTESIAN_POINT ( 'NONE',  ( -17.13090252310000139, -0.3058267005333999977, 314.8616023057000461 ) ) ;
#633=ORIENTED_EDGE ( 'NONE', *, *, #4237, .T. ) ;
#634=CARTESIAN_POINT ( 'NONE',  ( 1.232798796115999851, -12.07489154382001040, 189.9229057364800042 ) ) ;
#635=CARTESIAN_POINT ( 'NONE',  ( 9.974269275089660880, 10.84391064191637000, 190.9999999999996589 ) ) ;
#639=CARTESIAN_POINT ( 'NONE',  ( -12.21495827233999876, -7.290170534263999969, 314.4150829855000211 ) ) ;
#642=CARTESIAN_POINT ( 'NONE',  ( 11.73784133842000088, 9.026952533543999735, 320.0000000000000000 ) ) ;
#643=CARTESIAN_POINT ( 'NONE',  ( -1.281333103385001726, -11.37293729856000368, 319.9928079742500131 ) ) ;
#644=CARTESIAN_POINT ( 'NONE',  ( 12.21612826667444729, 9.907025583609536667, 319.0000000000005116 ) ) ;
#645=CARTESIAN_POINT ( 'NONE',  ( -17.50000000000000711, 8.653861160270983887E-10, 190.0000000000000568 ) ) ;
#648=CARTESIAN_POINT ( 'NONE',  ( 10.23467948564923091, 9.999999999493891067, 190.0000000000002558 ) ) ;
#649=CARTESIAN_POINT ( 'NONE',  ( -17.84297720825001221, 4.977647671642006166, 189.9229057364800042 ) ) ;
#651=B_SPLINE_CURVE_WITH_KNOTS ( 'NONE', 3,
 ( #7741, #9568, #4623, #10319, #2960, #6230, #7896, #8699, #10222, #6077, #2857, #6178, #9366, #542, #3819, #7103, #2907, #8589, #9413, #4463, #5316, #9516, #1237, #2157, #10370, #2207, #9462, #439, #8754, #1397, #2102, #1293, #4680, #4513, #600, #6895, #2001, #7793, #5265 ),
 .UNSPECIFIED., .F., .F.,
 ( 4, 1, 1, 1, 1, 1, 1, 1, 1, 1, 1, 1, 1, 1, 1, 1, 1, 1, 1, 1, 1, 1, 1, 1, 1, 1, 1, 1, 1, 1, 1, 1, 1, 1, 1, 1, 4 ),
 ( 0.000000000000000000, 0.02777777777778000015, 0.05555555555556000030, 0.08333333333333001192, 0.1111111111111000027, 0.1388888888888999973, 0.1666666666667000196, 0.1944444444444000109, 0.2222222222222000054, 0.2500000000000000000, 0.2777777777777999946, 0.3055555555555999891, 0.3333333333333000081, 0.3611111111111000027, 0.3888888888888999973, 0.4166666666666999919, 0.4444444444444000109, 0.4722222222222000054, 0.5000000000000000000, 0.5277777777777999946, 0.5555555555555999891, 0.5833333333333000637, 0.6111111111111000582, 0.6388888888888999418, 0.6666666666667000474, 0.6944444444444000109, 0.7222222222222000054, 0.7500000000000000000, 0.7777777777777999946, 0.8055555555555999891, 0.8333333333333000637, 0.8611111111111000582, 0.8888888888888999418, 0.9166666666667000474, 0.9444444444444000109, 0.9722222222222000054, 1.000000000000000000 ),
 .UNSPECIFIED. ) ;
#653=FACE_OUTER_BOUND ( 'NONE', #7217, .T. ) ;
#654=CARTESIAN_POINT ( 'NONE',  ( 11.77008734995756178, 6.834641529527616832, 315.0000000000000568 ) ) ;
#659=CARTESIAN_POINT ( 'NONE',  ( -18.86319819242002183, -0.4765179085981003926, 319.9928079742500131 ) ) ;
#662=CARTESIAN_POINT ( 'NONE',  ( -6.769722431736004076, 11.85293133419998846, -317.0792622552969533 ) ) ;
#663=CARTESIAN_POINT ( 'NONE',  ( 3.762811461229003562, -12.28417267642999278, -316.3802825947000201 ) ) ;
#666=B_SPLINE_CURVE_WITH_KNOTS ( 'NONE', 3,
 ( #4430, #5384, #5329, #349, #4384, #10335, #8456, #2766, #4475, #7755, #9429, #3676, #8664, #1097, #6963, #10237, #6038, #9328, #1964, #6909, #2873, #8605, #1251, #3728, #10285, #2924, #558, #4860, #7225, #8886, #8939, #7169, #3079, #8832, #8715, #9530, #2388, #2224, #7331, #10439, #4055, #7912, #5493, #3890, #2170, #9748 ),
 .UNSPECIFIED., .F., .F.,
 ( 4, 2, 2, 2, 2, 2, 2, 2, 2, 2, 2, 2, 2, 2, 2, 2, 2, 2, 2, 2, 2, 2, 4 ),
 ( 0.000000000000000000, 0.001362852592701295929, 0.002044278889051944111, 0.002725705185402593159, 0.004088557778103887354, 0.005451410370805182849, 0.006814262963506478345, 0.008177115556207774708, 0.01090282074161036743, 0.01635423111241555982, 0.01907993629781816122, 0.02180564148322075915, 0.02453134666862336055, 0.02725705185402596195, 0.02998275703942856335, 0.03270846222483116128, 0.03543416741023376615, 0.03815987259563636408, 0.03952272518833765264, 0.04088557778103895507, 0.04224843037374024363, 0.04292985667009089484, 0.04361128296644153912 ),
 .UNSPECIFIED. ) ;
#669=CARTESIAN_POINT ( 'NONE',  ( 16.99996037728000076, -1.352915083302999933E-09, -314.9999801883000146 ) ) ;
#672=CARTESIAN_POINT ( 'NONE',  ( 10.97430844189483423, -10.45950866754415820, 319.0000000000003979 ) ) ;
#674=CARTESIAN_POINT ( 'NONE',  ( 13.89291764776418603, 9.007512922137015821, -316.5000000000004547 ) ) ;
#675=ORIENTED_EDGE ( 'NONE', *, *, #9162, .F. ) ;
#676=CARTESIAN_POINT ( 'NONE',  ( -5.241997271368903810, -9.033710068163633977, 315.0000000000000000 ) ) ;
#677=CARTESIAN_POINT ( 'NONE',  ( -20.06799914428001941, 0.4075895895062001673, -302.9207377450070453 ) ) ;
#683=CARTESIAN_POINT ( 'NONE',  ( -5.058393412147005108, 12.18538300202998315, -302.9207377450070453 ) ) ;
#684=CARTESIAN_POINT ( 'NONE',  ( -12.21300849950000433, -9.900542285453001412, 318.8802828394900644 ) ) ;
#686=CARTESIAN_POINT ( 'NONE',  ( 13.62823431091000081, -6.408810695481999886, -314.4150829855000211 ) ) ;
#689=CARTESIAN_POINT ( 'NONE',  ( 16.06649953495000105, -6.900914778667005756, 189.9229057364800042 ) ) ;
#690=CARTESIAN_POINT ( 'NONE',  ( -13.10504385913262837, 9.452822371482907826, 190.9999999999996589 ) ) ;
#695=CARTESIAN_POINT ( 'NONE',  ( 1.388768300183999882, -9.421618921053999784, 315.0848619657999734 ) ) ;
#701=CARTESIAN_POINT ( 'NONE',  ( 1.279515965483999906E-07, 10.00000000755999885, 190.0000000000000000 ) ) ;
#702=CARTESIAN_POINT ( 'NONE',  ( -4.791123986588002204, 11.72534684832999119, 189.9229057364800042 ) ) ;
#706=( BOUNDED_SURFACE ( )  B_SPLINE_SURFACE ( 3, 1, ( 
 ( #9973, #6695 ),
 ( #7344, #9011 ),
 ( #5876, #1646 ),
 ( #9168, #7446 ),
 ( #32, #10026 ),
 ( #2508, #6588 ),
 ( #4922, #8198 ) ),
 .UNSPECIFIED., .F., .F., .F. ) 
 B_SPLINE_SURFACE_WITH_KNOTS ( ( 4, 3, 4 ),
 ( 2, 2 ),
 ( 0.000000000000000000, 0.5000000000000000000, 1.000000000000000000 ),
 ( 0.000000000000000000, 1.000000000000000000 ),
 .UNSPECIFIED. ) 
 GEOMETRIC_REPRESENTATION_ITEM ( )  RATIONAL_B_SPLINE_SURFACE ( (
 ( 1.000000000000000000, 1.000000000000000000),
 ( 0.8047378516590519837, 0.8047378516590519837),
 ( 0.8047378516590519837, 0.8047378516590519837),
 ( 1.000000000000000000, 1.000000000000000000),
 ( 0.8047378516590519837, 0.8047378516590519837),
 ( 0.8047378516590519837, 0.8047378516590519837),
 ( 1.000000000000000000, 1.000000000000000000) ) ) 
 REPRESENTATION_ITEM ( '' )  SURFACE ( )  );
#707=CARTESIAN_POINT ( 'NONE',  ( 17.49999999954662044, -9.625715914672042649E-06, 190.0000000000000000 ) ) ;
#710=CARTESIAN_POINT ( 'NONE',  ( 16.98808798087999961, 1.334629195702000004, -314.8616023057000461 ) ) ;
#712=CARTESIAN_POINT ( 'NONE',  ( -19.37251270682998694, 1.820313540576997680, 320.0770942683900557 ) ) ;
#716=CARTESIAN_POINT ( 'NONE',  ( 18.19038122738000141, 4.511441183124001775, -317.5770954168139610 ) ) ;
#717=CARTESIAN_POINT ( 'NONE',  ( 18.56065892533998962, -4.703159488203003669, -316.3802825947000201 ) ) ;
#718=CARTESIAN_POINT ( 'NONE',  ( -18.53598399141000286, -2.541378258162000137, 320.0000000000000000 ) ) ;
#719=AXIS2_PLACEMENT_3D ( 'NONE', #5470, #4675, #10264 ) ;
#721=CARTESIAN_POINT ( 'NONE',  ( 16.53772850381890791, -2.187491735906823997, -314.9999999999998863 ) ) ;
#725=CARTESIAN_POINT ( 'NONE',  ( 15.92495094281444601, 7.583842622554345603, -316.5000000000004547 ) ) ;
#727=( BOUNDED_CURVE ( )  B_SPLINE_CURVE ( 3, ( #4537, #2178, #9337, #3788, #7716, #7022, #2073 ),
 .UNSPECIFIED., .F., .T. ) 
 B_SPLINE_CURVE_WITH_KNOTS ( ( 4, 3, 4 ),
 ( 0.006576891565977574343, 0.5000000000000000000, 0.9934231084340225948 ),
 .UNSPECIFIED. ) 
 CURVE ( )  GEOMETRIC_REPRESENTATION_ITEM ( )  RATIONAL_B_SPLINE_CURVE ( ( 0.9922222087809801083, 0.8003084355045907428, 0.8029010325775972623, 1.000000000000000000, 0.8029010325775971513, 0.8003084355045906317, 0.9922222087809804414 ) ) 
 REPRESENTATION_ITEM ( '' )  );
#728=CARTESIAN_POINT ( 'NONE',  ( -14.89844356947526727, -4.564575774521109963, 315.0000000000000000 ) ) ;
#729=CARTESIAN_POINT ( 'NONE',  ( 4.978480136836995307, -11.69377972944999478, -302.4229045757450081 ) ) ;
#734=CARTESIAN_POINT ( 'NONE',  ( -1.652129430310999236, 12.05325387113999014, -302.4229045757450081 ) ) ;
#735=CARTESIAN_POINT ( 'NONE',  ( 19.98389199037000452, 0.4027620370101000491, 318.8802828394900644 ) ) ;
#736=ORIENTED_EDGE ( 'NONE', *, *, #7510, .T. ) ;
#737=CARTESIAN_POINT ( 'NONE',  ( 10.49789511286000021, -7.639556387670999982, -314.8616023057000461 ) ) ;
#738=CARTESIAN_POINT ( 'NONE',  ( -17.57673583306999632, -0.3313182897943000582, 314.4150829855000211 ) ) ;
#740=CARTESIAN_POINT ( 'NONE',  ( 4.791123986588002204, -11.72534684832999119, 189.9229057364800042 ) ) ;
#741=CARTESIAN_POINT ( 'NONE',  ( -19.78120799650142558, 1.924098540961039605, 190.9999999999996589 ) ) ;
#743=CARTESIAN_POINT ( 'NONE',  ( 1.399029207469000058, -9.644928263551999947, 314.8616023057000461 ) ) ;
#744=CARTESIAN_POINT ( 'NONE',  ( -18.95675155274000190, 0.9190877154199000865, 320.0000000000000000 ) ) ;
#746=CARTESIAN_POINT ( 'NONE',  ( 18.71196753105320099, 4.439097376277246099, 319.0000000000005116 ) ) ;
#747=DIRECTION ( 'NONE',  ( 0.000000000000000000, 0.000000000000000000, 1.000000000000000000 ) ) ;
#749=CARTESIAN_POINT ( 'NONE',  ( -11.71572875797656188, 12.49999999864037825, -303.5000000000000000 ) ) ;
#753=CARTESIAN_POINT ( 'NONE',  ( 14.08994485310920730, 5.290256584484003710, 314.9999999999999432 ) ) ;
#755=CARTESIAN_POINT ( 'NONE',  ( -11.70471109486296690, -10.14826236475114740, -303.4999999999996589 ) ) ;
#756=CARTESIAN_POINT ( 'NONE',  ( 16.19514236092000203, 2.730451569713999938, -315.0848619657999734 ) ) ;
#760=CARTESIAN_POINT ( 'NONE',  ( 17.64852322130001738, 5.886271888320000478, 318.8802828394900644 ) ) ;
#761=CARTESIAN_POINT ( 'NONE',  ( 10.00000000000000000, 2.500000000000000000, -285.0000000000000000 ) ) ;
#763=CARTESIAN_POINT ( 'NONE',  ( 7.006889269069000115, 6.844138725329000472, -284.9999999999999432 ) ) ;
#765=CARTESIAN_POINT ( 'NONE',  ( 19.86719273998999213, 1.743644188460999667, -316.3802825947000201 ) ) ;
#766=CARTESIAN_POINT ( 'NONE',  ( -19.98383894087000812, 0.4026063077914996402, -316.3802825947000201 ) ) ;
#769=CARTESIAN_POINT ( 'NONE',  ( -18.78897325516000194, -1.756194273835000041, 320.0000000000000000 ) ) ;
#777=FACE_OUTER_BOUND ( 'NONE', #6314, .T. ) ;
#779=CARTESIAN_POINT ( 'NONE',  ( -5.323201728285183343, 12.06184864676790269, -316.5000000000004547 ) ) ;
#781=CARTESIAN_POINT ( 'NONE',  ( 19.97270637197000909, 0.5553832019671997022, -303.6197174156509391 ) ) ;
#785=CARTESIAN_POINT ( 'NONE',  ( 5.185096592093999313, 11.65847420015999170, -302.4229045757450081 ) ) ;
#792=CARTESIAN_POINT ( 'NONE',  ( -16.79769345205001585, -5.168336178625003718, 190.0071920248299477 ) ) ;
#793=CARTESIAN_POINT ( 'NONE',  ( 11.03108320835583633, 10.43614982842405858, 190.9999999999996589 ) ) ;
#794=CARTESIAN_POINT ( 'NONE',  ( 8.096765587028130540, 8.344222180821057933, -315.0000000000000000 ) ) ;
#796=VECTOR ( 'NONE', #10114, 1000.000000000000000 ) ;
#797=CARTESIAN_POINT ( 'NONE',  ( -16.89608781496000134, -0.5923740909019999945, 315.0848619657999734 ) ) ;
#798=CARTESIAN_POINT ( 'NONE',  ( 17.81405818021000087, 3.987619665940000502, 320.0000000000000000 ) ) ;
#799=CARTESIAN_POINT ( 'NONE',  ( -18.89057790499001754, -0.06397434778252995835, 319.9928079742500131 ) ) ;
#800=CARTESIAN_POINT ( 'NONE',  ( 14.88027513490714249, 8.363422937417032799, 319.0000000000005116 ) ) ;
#802=CARTESIAN_POINT ( 'NONE',  ( -14.79012398733999945, 1.483731117707000058, 315.0000000000000000 ) ) ;
#806=CARTESIAN_POINT ( 'NONE',  ( 14.89844356947526727, 4.564575774521109963, 315.0000000000000000 ) ) ;
#808=CARTESIAN_POINT ( 'NONE',  ( 17.34710322845000263, -0.4172063223308000168, -314.6383426456000052 ) ) ;
#810=EDGE_CURVE ( 'NONE', #8301, #3853, #10500, .T. ) ;
#811=B_SPLINE_CURVE_WITH_KNOTS ( 'NONE', 3,
 ( #7075, #6916, #7815, #461, #3585, #10343, #6865, #2832, #1158, #6101, #10294, #2931, #6199, #4704, #6306, #8085, #623, #9590, #9644, #6363, #728, #2286, #4004, #3144, #2394, #8723, #5551, #6417, #5610, #4649, #8778, #2232, #5660, #7231, #7983, #8839, #7126, #10445, #1483, #3842, #7919, #4761, #7284, #8031, #3897, #1421, #8945, #9701, #3086, #7176, #676, #5499, #566, #3951, #2341, #4814, #10498, #10393, #8892, #1531, #10560, #3033, #3200, #6472, #9754, #1589, #1366, #6130, #7796, #2105, #442, #7003, #8702, #6951, #1241, #1186, #1346, #5480, #6080, #7744, #8759, #7057, #7694, #387, #10321, #2963, #9571, #10275, #496, #1400, #2004, #4628, #3661, #6234, #5371, #3615, #2860, #2807, #9370, #10225, #5318, #9417, #7900, #545, #5268, #6897, #337, #2053, #3821, #9464, #7106, #9521, #8543, #8592, #4465, #10375, #4517, #3717, #10164, #2912, #3015, #6180, #8652, #6289, #1295, #2211, #4575, #7849, #3764, #2160, #5426, #4558, #6437 ),
 .UNSPECIFIED., .F., .F.,
 ( 4, 1, 1, 1, 1, 1, 2, 2, 1, 1, 1, 1, 1, 2, 2, 1, 1, 1, 1, 1, 2, 2, 1, 1, 1, 1, 1, 2, 2, 1, 1, 1, 1, 1, 1, 2, 2, 1, 1, 1, 1, 1, 2, 2, 1, 1, 2, 2, 2, 1, 1, 2, 2, 1, 1, 1, 1, 2, 2, 1, 1, 1, 1, 1, 1, 2, 2, 1, 1, 1, 1, 1, 2, 2, 1, 1, 1, 1, 1, 2, 2, 1, 1, 1, 1, 1, 2, 2, 1, 1, 1, 1, 2, 2, 1, 1, 1, 2, 2, 4 ),
 ( 0.000000000000000000, 0.06250000000000791034, 0.09375000000001181000, 0.1093750000000137529, 0.1171875000000147105, 0.1210937500000152794, 0.1230468750000155709, 0.1250000000000158484, 0.1562500000000223432, 0.1718750000000255906, 0.1796875000000270617, 0.1835937500000277833, 0.1855468750000281719, 0.1865234375000283107, 0.1875000000000284217, 0.2187500000000311418, 0.2343750000000323908, 0.2421875000000330014, 0.2460937500000334177, 0.2480468750000336398, 0.2490234375000336953, 0.2500000000000337508, 0.2812500000000370259, 0.2968750000000386358, 0.3046875000000394684, 0.3085937500000398570, 0.3105468750000400235, 0.3115234375000401346, 0.3125000000000403011, 0.3437500000000445199, 0.3593750000000465739, 0.3671875000000476286, 0.3710937500000481282, 0.3730468750000484057, 0.3740234375000484612, 0.3745117187500484612, 0.3750000000000484612, 0.4062500000000490163, 0.4218750000000493494, 0.4296875000000495159, 0.4335937500000495715, 0.4355468750000495715, 0.4365234375000495715, 0.4375000000000495715, 0.4531250000000494604, 0.4609375000000494049, 0.4648437500000494049, 0.4687500000000494049, 0.5000000000000491829, 0.5156250000000491829, 0.5234375000000491829, 0.5273437500000490719, 0.5312500000000490719, 0.5468750000000488498, 0.5546875000000488498, 0.5585937500000488498, 0.5605468750000488498, 0.5615234375000488498, 0.5625000000000488498, 0.5937500000000481837, 0.6093750000000478506, 0.6171875000000476286, 0.6210937500000475175, 0.6230468750000474065, 0.6240234375000474065, 0.6245117187500474065, 0.6250000000000472955, 0.6562500000000430767, 0.6718750000000409672, 0.6796875000000398570, 0.6835937500000393019, 0.6855468750000390799, 0.6865234375000389688, 0.6875000000000388578, 0.7187500000000363043, 0.7343750000000350830, 0.7421875000000345279, 0.7460937500000343059, 0.7480468750000340838, 0.7490234375000340838, 0.7500000000000340838, 0.7812500000000317524, 0.7968750000000304201, 0.8046875000000298650, 0.8085937500000295319, 0.8105468750000293099, 0.8115234375000293099, 0.8125000000000293099, 0.8437500000000242029, 0.8593750000000216493, 0.8671875000000203171, 0.8710937500000196509, 0.8730468750000193179, 0.8750000000000189848, 0.9062500000000143219, 0.9218750000000121014, 0.9296875000000109912, 0.9335937500000103251, 0.9375000000000097700, 1.000000000000000000 ),
 .UNSPECIFIED. ) ;
#817=CARTESIAN_POINT ( 'NONE',  ( 13.93268562690000678, 9.073621533052996568, -317.0792622552969533 ) ) ;
#820=CARTESIAN_POINT ( 'NONE',  ( -14.99960151356000004, -7.033824075090999273, 320.0000000000000000 ) ) ;
#825=CARTESIAN_POINT ( 'NONE',  ( 8.900723324022980165, -8.081813809772741664, -315.0000000000000000 ) ) ;
#827=CARTESIAN_POINT ( 'NONE',  ( 12.98706127646999953, 6.788989183774999603, -314.4963898845653603 ) ) ;
#829=CARTESIAN_POINT ( 'NONE',  ( -13.36995595564000006, 8.154012700520999246, -317.5000000000000000 ) ) ;
#833=EDGE_CURVE ( 'NONE', #245, #7676, #3711, .T. ) ;
#834=CARTESIAN_POINT ( 'NONE',  ( -15.00000000000000000, -0.4945770392355999800, 315.0000000000000000 ) ) ;
#835=CARTESIAN_POINT ( 'NONE',  ( -16.93986923087000562, 6.779672025222003739, -302.9207377450070453 ) ) ;
#836=DIRECTION ( 'NONE',  ( 0.000000000000000000, 1.000000000000000000, 0.000000000000000000 ) ) ;
#838=DIRECTION ( 'NONE',  ( 1.000000000000000000, 0.000000000000000000, 0.000000000000000000 ) ) ;
#841=CARTESIAN_POINT ( 'NONE',  ( -19.56991616969001058, 0.3941640562313002416, 189.9229057364800042 ) ) ;
#842=CARTESIAN_POINT ( 'NONE',  ( -13.99679147458261319, 8.939383429014137405, 190.9999999999996589 ) ) ;
#843=CARTESIAN_POINT ( 'NONE',  ( 11.72583169940718584, 6.858410958448125427, -315.0000000000000000 ) ) ;
#845=AXIS2_PLACEMENT_3D ( 'NONE', #2139, #530, #7882 ) ;
#846=CARTESIAN_POINT ( 'NONE',  ( 13.37260572687999982, -6.041714840053000302, 314.8616023057000461 ) ) ;
#847=CARTESIAN_POINT ( 'NONE',  ( 6.294482982547999761, 10.85527983184999989, 320.0000000000000000 ) ) ;
#848=CARTESIAN_POINT ( 'NONE',  ( 16.03176714517000079, -6.932210726315004123, 320.0770942683900557 ) ) ;
#849=CARTESIAN_POINT ( 'NONE',  ( -19.95988936745280995, 0.9706423173584770581, 319.0000000000005116 ) ) ;
#850=CARTESIAN_POINT ( 'NONE',  ( 16.84717009645851604, 6.762270094121639374, -303.4999999999990905 ) ) ;
#851=CARTESIAN_POINT ( 'NONE',  ( 11.99990625867999938, 6.898016740823000426, 314.8616023057000461 ) ) ;
#852=ORIENTED_EDGE ( 'NONE', *, *, #3700, .T. ) ;
#858=CARTESIAN_POINT ( 'NONE',  ( 13.64105609808563457, 5.653588212731087026, 315.0000000000000000 ) ) ;
#864=CARTESIAN_POINT ( 'NONE',  ( 10.49155472272000011, 10.73755170802999714, -317.0792622552969533 ) ) ;
#868=CARTESIAN_POINT ( 'NONE',  ( 16.83239583074999857, -5.311267823799999732, 320.0000000000000000 ) ) ;
#870=PRODUCT_DEFINITION_CONTEXT ( 'detailed design', #5238, 'design' ) ;
#871=DIRECTION ( 'NONE',  ( 0.000000000000000000, 0.000000000000000000, -1.000000000000000000 ) ) ;
#872=CARTESIAN_POINT ( 'NONE',  ( 14.00145308865741711, -5.362717611231083481, -315.0000000000000000 ) ) ;
#874=CARTESIAN_POINT ( 'NONE',  ( -8.037373804805000077, 9.179324345868998591, -314.4963898845653603 ) ) ;
#876=CARTESIAN_POINT ( 'NONE',  ( 18.99987372849000167, 0.5562009942294000586, -317.4999999998989892 ) ) ;
#879=CARTESIAN_POINT ( 'NONE',  ( -20.01660392705000646, -0.3690847706228002623, -303.6197174156509391 ) ) ;
#884=CARTESIAN_POINT ( 'NONE',  ( 5.254364691879999327, 12.06635523715000424, -303.6197174156520759 ) ) ;
#892=CARTESIAN_POINT ( 'NONE',  ( 6.420662313211997763, -11.93024803506000531, 190.4207385301700128 ) ) ;
#894=CARTESIAN_POINT ( 'NONE',  ( 15.06645494800450891, 4.378519400638148262, -315.0000000000000568 ) ) ;
#896=CARTESIAN_POINT ( 'NONE',  ( -11.20196042648000123, 10.44833032063000111, 190.4207385301700128 ) ) ;
#897=CARTESIAN_POINT ( 'NONE',  ( 13.24479143485999977, -5.858166912337999577, 315.0848619657999734 ) ) ;
#900=LINE ( 'NONE', #1923, #3134 ) ;
#901=CARTESIAN_POINT ( 'NONE',  ( 19.57081977481000834, 0.3814303831828999014, 320.0770942683900557 ) ) ;
#903=( NAMED_UNIT ( * ) SI_UNIT ( $, .STERADIAN. ) SOLID_ANGLE_UNIT ( ) );
#904=CARTESIAN_POINT ( 'NONE',  ( 6.273744347102000241, 8.772995918477999311, 315.0848619657999734 ) ) ;
#909=CARTESIAN_POINT ( 'NONE',  ( -11.54746845216141082, 6.952771041492575854, 315.0000000000000000 ) ) ;
#915=CARTESIAN_POINT ( 'NONE',  ( 14.18540515794000001, 7.627402598852000004, 190.0000000000000000 ) ) ;
#917=CARTESIAN_POINT ( 'NONE',  ( 0.000000000000000000, 7.937240849781000307, -284.9999999999999432 ) ) ;
#919=CARTESIAN_POINT ( 'NONE',  ( 7.863726017345004315, 11.49810175465000661, -316.3802825947000201 ) ) ;
#923=DIRECTION ( 'NONE',  ( 0.000000000000000000, 0.000000000000000000, 1.000000000000000000 ) ) ;
#925=CARTESIAN_POINT ( 'NONE',  ( 13.64075175739776924, -5.653800323622448332, -315.0000000000000000 ) ) ;
#928=CARTESIAN_POINT ( 'NONE',  ( 0.000000000000000000, 10.54711710274999881, -314.4963898845653603 ) ) ;
#929=AXIS2_PLACEMENT_3D ( 'NONE', #6785, #1073, #8433 ) ;
#934=CARTESIAN_POINT ( 'NONE',  ( 6.550050338814993545, -11.90210887660999184, -302.9207377450070453 ) ) ;
#935=CARTESIAN_POINT ( 'NONE',  ( -3.239095488904002007, -11.22417384501999038, -317.4928077629770087 ) ) ;
#936=FACE_OUTER_BOUND ( 'NONE', #3393, .T. ) ;
#938=VECTOR ( 'NONE', #1431, 1000.000000000000000 ) ;
#941=CARTESIAN_POINT ( 'NONE',  ( 11.70175841024000185, 10.14170047206000014, -303.6197174156520759 ) ) ;
#942=CARTESIAN_POINT ( 'NONE',  ( -13.64771691246352781, -6.290639962997291335, 314.4999474536514299 ) ) ;
#944=PLANE ( 'NONE',  #427 ) ;
#947=CARTESIAN_POINT ( 'NONE',  ( 19.77421425755001039, -1.922351829117000976, 191.1197171614399792 ) ) ;
#949=CARTESIAN_POINT ( 'NONE',  ( 11.65180110541762737, 6.897852064324585974, -315.0000000000000000 ) ) ;
#951=CARTESIAN_POINT ( 'NONE',  ( 2.648868200019002472, 12.40196232477001459, 191.1197171614399792 ) ) ;
#952=CARTESIAN_POINT ( 'NONE',  ( 16.92217352393999974, -0.01966449385450000364, 315.0848619657999734 ) ) ;
#954=CARTESIAN_POINT ( 'NONE',  ( -7.740399053647997185, -11.10168159160000201, 320.0770942683900557 ) ) ;
#955=CARTESIAN_POINT ( 'NONE',  ( -9.425149215659013535, 8.435515111409248590, 314.4999430218502425 ) ) ;
#956=CARTESIAN_POINT ( 'NONE',  ( -14.97723399828063506, 8.302382553459795034, -303.5000000000000000 ) ) ;
#957=CARTESIAN_POINT ( 'NONE',  ( 17.59334121105999671, 0.04733121045982999903, 314.4150829855000211 ) ) ;
#959=CARTESIAN_POINT ( 'NONE',  ( 3.129133257132350465, -12.36387889853562960, 190.9999999999995737 ) ) ;
#960=CARTESIAN_POINT ( 'NONE',  ( -20.04253597850999569, 0.9484392003694999129, 319.5792614743400009 ) ) ;
#967=CARTESIAN_POINT ( 'NONE',  ( -11.72570362167166635, 6.858483604278664103, 315.0000000000000000 ) ) ;
#970=CARTESIAN_POINT ( 'NONE',  ( -0.1867348994714999877, -11.51775814840000045, -302.5000000000000000 ) ) ;
#973=CARTESIAN_POINT ( 'NONE',  ( -15.48916725177958220, 3.890278845006961195, -314.9999999999999432 ) ) ;
#976=CARTESIAN_POINT ( 'NONE',  ( 19.95007997204999839, 1.762487863542002486, -317.0792622552969533 ) ) ;
#981=CARTESIAN_POINT ( 'NONE',  ( -0.3940538687071432067, -9.499927474253880177, -315.0000000000000568 ) ) ;
#983=CARTESIAN_POINT ( 'NONE',  ( 17.50000000000125766, -0.2304358844820579011, -314.4997350343306266 ) ) ;
#984=CARTESIAN_POINT ( 'NONE',  ( 9.374494192145222726, -11.05367988180385197, -316.5000000000004547 ) ) ;
#986=CARTESIAN_POINT ( 'NONE',  ( 15.26883884775999967, 6.827716174106000402, -317.5000000000000000 ) ) ;
#988=CARTESIAN_POINT ( 'NONE',  ( 7.947966332010000023, -11.56278913298000077, -302.9207377450070453 ) ) ;
#989=CARTESIAN_POINT ( 'NONE',  ( 9.242264416715993747, -10.65406548831999878, -317.5770954168139610 ) ) ;
#990=CARTESIAN_POINT ( 'NONE',  ( -15.74033075358999945, 3.452242816619000010, -315.0848619657999734 ) ) ;
#992=CARTESIAN_POINT ( 'NONE',  ( 1.983590419337998734, 12.44807596301999908, -303.6197174156509391 ) ) ;
#996=CARTESIAN_POINT ( 'NONE',  ( -13.37992741786000117, 8.147955808703001068, -302.5000000000000000 ) ) ;
#998=CARTESIAN_POINT ( 'NONE',  ( -4.478082317681002955, -12.27758592791000147, 190.4207385301700128 ) ) ;
#1001=CARTESIAN_POINT ( 'NONE',  ( -1.252197968602001943, 12.57265714642999477, 190.4207385301700128 ) ) ;
#1004=CARTESIAN_POINT ( 'NONE',  ( 17.57673583306999632, 0.3313182897943000582, 314.4150829855000211 ) ) ;
#1006=CARTESIAN_POINT ( 'NONE',  ( -19.56990143371999125, 0.3944980022354002136, 320.0770942683900557 ) ) ;
#1007=CARTESIAN_POINT ( 'NONE',  ( -11.05300986228076354, 7.762248751444681183, 314.4999426419797715 ) ) ;
#1008=CARTESIAN_POINT ( 'NONE',  ( 18.54125634398932121, 4.746072667744948959, -303.4999999999990905 ) ) ;
#1009=CARTESIAN_POINT ( 'NONE',  ( 15.39920013370999996, 4.579805981517999669, 314.6383426456000052 ) ) ;
#1010=VERTEX_POINT ( 'NONE', #2776 ) ;
#1012=CARTESIAN_POINT ( 'NONE',  ( -20.06808111288002294, -0.4071096865243000185, 319.5792614743400009 ) ) ;
#1015=CARTESIAN_POINT ( 'NONE',  ( -4.578954556310520729, 9.145511589803685837, 315.0000000000000000 ) ) ;
#1020=LINE ( 'NONE', #9142, #9353 ) ;
#1025=CARTESIAN_POINT ( 'NONE',  ( 16.56500304494299058, -3.264221034209901617, 314.4999403627581387 ) ) ;
#1032=CARTESIAN_POINT ( 'NONE',  ( 7.042363285622346147, -8.656086706473070436, -314.9999999999999432 ) ) ;
#1036=CARTESIAN_POINT ( 'NONE',  ( -12.80773887004084877, -9.614708322195335555, -316.5000000000004547 ) ) ;
#1041=CARTESIAN_POINT ( 'NONE',  ( -19.99999721801999897, -7.771324026006999692E-11, 191.0000000000000000 ) ) ;
#1042=CARTESIAN_POINT ( 'NONE',  ( 16.58827648083000028, -6.426222433883002516, -317.5770954168139610 ) ) ;
#1043=CARTESIAN_POINT ( 'NONE',  ( -17.13090252310000139, -0.3058267005333000221, -314.8616023057000461 ) ) ;
#1046=CARTESIAN_POINT ( 'NONE',  ( -19.87644374459000929, 1.701742232560001788, -303.6197174156509391 ) ) ;
#1050=CARTESIAN_POINT ( 'NONE',  ( 9.006891093149000938, 10.12158591819999920, -302.5000000000000000 ) ) ;
#1051=APPLICATION_CONTEXT ( 'automotive_design' ) ;
#1053=CARTESIAN_POINT ( 'NONE',  ( 9.036610176479998202, -11.24204914511999398, 190.4207385301700128 ) ) ;
#1055=CARTESIAN_POINT ( 'NONE',  ( -6.445894847559003438, -10.69844988487999693, -302.5071922382879279 ) ) ;
#1056=CARTESIAN_POINT ( 'NONE',  ( -17.61637523988000353, 5.923742513492005202, 191.1197171614399792 ) ) ;
#1057=CARTESIAN_POINT ( 'NONE',  ( 4.061138133959000029, -9.851562218542998295, 314.4150829855000211 ) ) ;
#1059=CARTESIAN_POINT ( 'NONE',  ( 5.958765323235996725, -11.51784730653000643, 320.0770942683900557 ) ) ;
#1062=CARTESIAN_POINT ( 'NONE',  ( -1.674130924758677530, 12.47364919270561856, -303.5000000000000000 ) ) ;
#1063=CARTESIAN_POINT ( 'NONE',  ( 3.874983216044999956, 9.425407904674999671, 314.8616023057000461 ) ) ;
#1066=CARTESIAN_POINT ( 'NONE',  ( -18.75338617474996994, 4.519296150162002590, 319.5792614743400009 ) ) ;
#1070=CARTESIAN_POINT ( 'NONE',  ( -3.970161185191127817, 9.235879793686278205, 315.0000000000000000 ) ) ;
#1073=DIRECTION ( 'NONE',  ( 0.000000000000000000, 0.000000000000000000, 1.000000000000000000 ) ) ;
#1075=CARTESIAN_POINT ( 'NONE',  ( -14.21145943247442922, 5.188748475648758074, -315.0000000000000000 ) ) ;
#1080=ADVANCED_FACE ( 'NONE', ( #10245 ), #3998, .T. ) ;
#1085=VERTEX_POINT ( 'NONE', #1041 ) ;
#1086=CARTESIAN_POINT ( 'NONE',  ( 11.73041118561999951, 8.897639792529000502, 319.9928079742500131 ) ) ;
#1087=CARTESIAN_POINT ( 'NONE',  ( -10.46398288055045889, -10.66551579990979626, -316.5000000000004547 ) ) ;
#1092=CARTESIAN_POINT ( 'NONE',  ( -11.21026319665000948, -9.143022107836994650, -317.4928077629770087 ) ) ;
#1095=CARTESIAN_POINT ( 'NONE',  ( -15.10708484062000068, 4.236041382665999500, -315.0848619657999734 ) ) ;
#1097=CARTESIAN_POINT ( 'NONE',  ( 13.84663869404834102, 6.024484023773909236, -314.5809261257323897 ) ) ;
#1099=CARTESIAN_POINT ( 'NONE',  ( -3.214697847761800006E-15, 10.00000000000000000, 314.4999507458385892 ) ) ;
#1101=CARTESIAN_POINT ( 'NONE',  ( -18.53584076651999979, -2.541936159385000060, 190.0000000000000000 ) ) ;
#1102=FACE_OUTER_BOUND ( 'NONE', #1741, .T. ) ;
#1104=CARTESIAN_POINT ( 'NONE',  ( -19.96348645057001647, -0.8966426439394996617, 191.1197171614399792 ) ) ;
#1105=VERTEX_POINT ( 'NONE', #6138 ) ;
#1107=CARTESIAN_POINT ( 'NONE',  ( 18.90089112233000179, -0.2930644900430999789, -302.5071922382879279 ) ) ;
#1108=CARTESIAN_POINT ( 'NONE',  ( -19.12235363464000670, 3.679291565416002108, 191.1197171614399792 ) ) ;
#1113=EDGE_CURVE ( 'NONE', #2720, #1085, #9682, .T. ) ;
#1116=CARTESIAN_POINT ( 'NONE',  ( 20.08948270067001829, -0.1023867585008999687, 319.5792614743400009 ) ) ;
#1117=CARTESIAN_POINT ( 'NONE',  ( -17.50000000000000711, 8.653878165429867666E-10, 190.0000000000001137 ) ) ;
#1118=CARTESIAN_POINT ( 'NONE',  ( 1.276003512426000075, 9.874146089817999794, 314.6383426456000052 ) ) ;
#1120=CARTESIAN_POINT ( 'NONE',  ( 16.77317840633001467, -5.196478383294000025, 190.0071920248299477 ) ) ;
#1122=CARTESIAN_POINT ( 'NONE',  ( 13.19336277821000536, 9.492603533888004819, 319.5792614743400009 ) ) ;
#1124=CARTESIAN_POINT ( 'NONE',  ( 5.241997271368903810, 9.033710068163633977, 315.0000000000000000 ) ) ;
#1130=CARTESIAN_POINT ( 'NONE',  ( -3.134365345935000047, 11.35765845234000082, 190.0000000000000000 ) ) ;
#1131=( BOUNDED_SURFACE ( )  B_SPLINE_SURFACE ( 3, 3, ( 
 ( #4380, #2815, #5228, #2715, #3724, #246, #2867, #9377, #5981, #7010, #3522, #6801, #2011, #5178, #4425, #7651, #3570, #6852, #10121, #6032, #8505, #2663, #7701, #3624, #5276, #1193, #4472, #10233, #5324, #8600, #1248, #4524, #7804, #5930, #9221, #1854, #9581, #2918, #10486, #8878, #2220 ),
 ( #7858, #613, #1520, #6406, #1302, #503, #2113, #6186, #7114, #5379, #4800, #7163, #5596, #8072, #4636, #2970, #3074, #10434, #10281, #6241, #8660, #4582, #7064, #5433, #7218, #10329, #3128, #8767, #9527, #1408, #2167, #8711, #3886, #8822, #6348, #716, #3989, #9472, #1354, #9686, #2328 ),
 ( #9630, #7907, #552, #3829, #10382, #2272, #3771, #5488, #3022, #5538, #6296, #4691, #7967, #1468, #4749, #8019, #662, #3938, #4097, #7483, #8181, #125, #4902, #7375, #3238, #4853, #9149, #864, #2540, #2595, #817, #11, #3287, #6568, #10596, #9849, #6514, #976, #2487, #8338, #5756 ),
 ( #4152, #1575, #7430, #6626, #9954, #9044, #1679, #68, #3347, #4952, #8228, #9904, #8990, #5857, #3402, #5806, #9796, #9097, #1732, #5001, #1628, #1787, #4209, #8282, #6675, #919, #5057, #8128, #7271, #10542, #5646, #7325, #3186, #6459, #9740, #8931, #2382, #765, #4048, #2434, #5704 ) ),
 .UNSPECIFIED., .F., .F., .F. ) 
 B_SPLINE_SURFACE_WITH_KNOTS ( ( 4, 4 ),
 ( 4, 1, 1, 1, 1, 1, 1, 1, 1, 1, 1, 1, 1, 1, 1, 1, 1, 1, 1, 1, 1, 1, 1, 1, 1, 1, 1, 1, 1, 1, 1, 1, 1, 1, 1, 1, 1, 1, 4 ),
 ( 0.000000000000000000, 1.000000000000000000 ),
 ( -0.007738640450444999631, 0.000000000000000000, 0.03414709649185000001, 0.06696605908318999101, 0.09596079224771000837, 0.1211002772268999911, 0.1443783404606999998, 0.1680876537897000034, 0.1921286104184000143, 0.2160216200219000071, 0.2397245863996999848, 0.2634813019505999887, 0.2879188160025000220, 0.3133917475886000004, 0.3395543376315999784, 0.3663618195672999622, 0.3946229251345000355, 0.4252536485549999745, 0.4591139563344999730, 0.4956048897295999844, 0.5324779435423999674, 0.5674158629142000976, 0.5992726300609999557, 0.6287198090143000240, 0.6565915576515000129, 0.6836661054489000522, 0.7100337132233999204, 0.7353920520230999847, 0.7598724402797999433, 0.7838392479475999597, 0.8076909583479000565, 0.8317349054331000247, 0.8555088018188000687, 0.8788217029082999732, 0.9039691640437000908, 0.9329692239710999369, 0.9658153655582000230, 1.000000000000000000, 1.008464120473999914 ),
 .UNSPECIFIED. ) 
 GEOMETRIC_REPRESENTATION_ITEM ( )  RATIONAL_B_SPLINE_SURFACE ( (
 ( 1.236577356246000070, 1.236577356246000070, 1.236577356246000070, 1.236577356246000070, 1.236577356246000070, 1.236577356246000070, 1.236577356246000070, 1.236577356246000070, 1.236577356246000070, 1.236577356246000070, 1.236577356246000070, 1.236577356246000070, 1.236577356246000070, 1.236577356246000070, 1.236577356246000070, 1.236577356246000070, 1.236577356246000070, 1.236577356246000070, 1.236577356246000070, 1.236577356246000070, 1.236577356246000070, 1.236577356246000070, 1.236577356246000070, 1.236577356246000070, 1.236577356246000070, 1.236577356246000070, 1.236577356246000070, 1.236577356246000070, 1.236577356246000070, 1.236577356246000070, 1.236577356246000070, 1.236577356246000070, 1.236577356246000070, 1.236577356246000070, 1.236577356246000070, 1.236577356246000070, 1.236577356246000070, 1.236577356246000070, 1.236577356246000070, 1.236577356246000070, 1.236577356246000070),
 ( 0.9211408812511999722, 0.9211408812511999722, 0.9211408812511999722, 0.9211408812511999722, 0.9211408812511999722, 0.9211408812511999722, 0.9211408812511999722, 0.9211408812511999722, 0.9211408812511999722, 0.9211408812511999722, 0.9211408812511999722, 0.9211408812511999722, 0.9211408812511999722, 0.9211408812511999722, 0.9211408812511999722, 0.9211408812511999722, 0.9211408812511999722, 0.9211408812511999722, 0.9211408812511999722, 0.9211408812511999722, 0.9211408812511999722, 0.9211408812511999722, 0.9211408812511999722, 0.9211408812511999722, 0.9211408812511999722, 0.9211408812511999722, 0.9211408812511999722, 0.9211408812511999722, 0.9211408812511999722, 0.9211408812511999722, 0.9211408812511999722, 0.9211408812511999722, 0.9211408812511999722, 0.9211408812511999722, 0.9211408812511999722, 0.9211408812511999722, 0.9211408812511999722, 0.9211408812511999722, 0.9211408812511999722, 0.9211408812511999722, 0.9211408812511999722),
 ( 0.9211408812511999722, 0.9211408812511999722, 0.9211408812511999722, 0.9211408812511999722, 0.9211408812511999722, 0.9211408812511999722, 0.9211408812511999722, 0.9211408812511999722, 0.9211408812511999722, 0.9211408812511999722, 0.9211408812511999722, 0.9211408812511999722, 0.9211408812511999722, 0.9211408812511999722, 0.9211408812511999722, 0.9211408812511999722, 0.9211408812511999722, 0.9211408812511999722, 0.9211408812511999722, 0.9211408812511999722, 0.9211408812511999722, 0.9211408812511999722, 0.9211408812511999722, 0.9211408812511999722, 0.9211408812511999722, 0.9211408812511999722, 0.9211408812511999722, 0.9211408812511999722, 0.9211408812511999722, 0.9211408812511999722, 0.9211408812511999722, 0.9211408812511999722, 0.9211408812511999722, 0.9211408812511999722, 0.9211408812511999722, 0.9211408812511999722, 0.9211408812511999722, 0.9211408812511999722, 0.9211408812511999722, 0.9211408812511999722, 0.9211408812511999722),
 ( 1.236577356246000070, 1.236577356246000070, 1.236577356246000070, 1.236577356246000070, 1.236577356246000070, 1.236577356246000070, 1.236577356246000070, 1.236577356246000070, 1.236577356246000070, 1.236577356246000070, 1.236577356246000070, 1.236577356246000070, 1.236577356246000070, 1.236577356246000070, 1.236577356246000070, 1.236577356246000070, 1.236577356246000070, 1.236577356246000070, 1.236577356246000070, 1.236577356246000070, 1.236577356246000070, 1.236577356246000070, 1.236577356246000070, 1.236577356246000070, 1.236577356246000070, 1.236577356246000070, 1.236577356246000070, 1.236577356246000070, 1.236577356246000070, 1.236577356246000070, 1.236577356246000070, 1.236577356246000070, 1.236577356246000070, 1.236577356246000070, 1.236577356246000070, 1.236577356246000070, 1.236577356246000070, 1.236577356246000070, 1.236577356246000070, 1.236577356246000070, 1.236577356246000070) ) ) 
 REPRESENTATION_ITEM ( '' )  SURFACE ( )  );
#1132=CARTESIAN_POINT ( 'NONE',  ( 8.203579894969822206, -8.842447374029218210, 314.4999432750969390 ) ) ;
#1133=CARTESIAN_POINT ( 'NONE',  ( -17.27977314787002427, 4.562413721234999109, 190.0071920248299477 ) ) ;
#1141=CARTESIAN_POINT ( 'NONE',  ( 18.70127769336001222, 1.615776359209001312, 319.9928079742500131 ) ) ;
#1142=CARTESIAN_POINT ( 'NONE',  ( 19.86884641856056533, -1.746738893747486809, -316.5000000000004547 ) ) ;
#1144=ORIENTED_EDGE ( 'NONE', *, *, #2095, .F. ) ;
#1147=CARTESIAN_POINT ( 'NONE',  ( -10.31351018857999513, -10.27238149472999851, -317.5770954168139610 ) ) ;
#1148=ADVANCED_FACE ( 'NONE', ( #7751 ), #1131, .T. ) ;
#1153=CARTESIAN_POINT ( 'NONE',  ( -19.00000000000000000, 0.000000000000000000, 190.0000000000100044 ) ) ;
#1154=CARTESIAN_POINT ( 'NONE',  ( -14.88027513490713893, -8.363422937417031022, 319.0000000000003979 ) ) ;
#1156=CARTESIAN_POINT ( 'NONE',  ( -19.32351226214659690, 3.349534253028545461, -316.5000000000004547 ) ) ;
#1158=CARTESIAN_POINT ( 'NONE',  ( -16.37744599325981909, -2.527607301898085801, 314.9999999999999432 ) ) ;
#1161=CARTESIAN_POINT ( 'NONE',  ( 16.34352199340000311, 7.209047878930006092, 191.1197171614399792 ) ) ;
#1165=CARTESIAN_POINT ( 'NONE',  ( 17.60320223513998172, 4.128492944088002048, -302.5071922382879279 ) ) ;
#1166=CARTESIAN_POINT ( 'NONE',  ( -20.00482943604999164, -0.07455149923640995435, 318.8802828394900644 ) ) ;
#1168=CARTESIAN_POINT ( 'NONE',  ( 1.279515965483999906E-07, 10.00000000755999885, 190.0000000000000000 ) ) ;
#1169=CARTESIAN_POINT ( 'NONE',  ( -13.50042001888999899, 6.225262767767000049, 314.6383426456000052 ) ) ;
#1172=CARTESIAN_POINT ( 'NONE',  ( -13.88394749849000043, 9.000054837070988967, 318.8802828394900644 ) ) ;
#1173=B_SPLINE_SURFACE_WITH_KNOTS ( 'NONE', 3, 1, ( 
 ( #3373, #8463 ),
 ( #4126, #7402 ),
 ( #6650, #6595 ),
 ( #1866, #2677 ),
 ( #148, #4232 ),
 ( #7559, #9877 ),
 ( #3422, #5778 ),
 ( #9070, #7506 ),
 ( #2621, #9979 ),
 ( #5883, #9176 ),
 ( #1816, #8414 ),
 ( #5081, #1705 ),
 ( #7611, #4978 ) ),
 .UNSPECIFIED., .F., .F., .F.,
 ( 4, 1, 1, 1, 1, 1, 1, 1, 1, 1, 4 ),
 ( 2, 2 ),
 ( 0.01923076854978371733, 0.09935897435896999530, 0.1794871794871999993, 0.2596153846154000133, 0.3397435897436000274, 0.5000000000000000000, 0.6602564102564000281, 0.7403846153845999867, 0.8205128205128000562, 0.9006410256410000148, 0.9807692307692000844 ),
 ( 0.000000000000000000, 1.000000000000000000 ),
 .UNSPECIFIED. ) ;
#1179=CARTESIAN_POINT ( 'NONE',  ( -15.47196055635296474, 3.911380178888624215, -315.0000000000000568 ) ) ;
#1180=CARTESIAN_POINT ( 'NONE',  ( -18.85089486759000010, 0.8058634873976002755, 190.0071920248299477 ) ) ;
#1186=CARTESIAN_POINT ( 'NONE',  ( 4.532266548732788003, -9.152838354191798587, 315.0000000000000568 ) ) ;
#1187=CARTESIAN_POINT ( 'NONE',  ( 6.370857846455999507, 9.209451711050000711, -314.6383426456000052 ) ) ;
#1189=CARTESIAN_POINT ( 'NONE',  ( -11.51418862744999139, 9.000691300089004088, 319.9928079742500131 ) ) ;
#1192=ORIENTED_EDGE ( 'NONE', *, *, #9891, .F. ) ;
#1193=CARTESIAN_POINT ( 'NONE',  ( 7.576881921353003868, 10.42269368856000611, -317.4928077629770087 ) ) ;
#1196=CARTESIAN_POINT ( 'NONE',  ( -9.218822326027003911, -11.18653774893999220, -317.0792622552969533 ) ) ;
#1202=CARTESIAN_POINT ( 'NONE',  ( -14.94331899262999919, -7.078020551493000134, 190.0000000000000000 ) ) ;
#1204=CARTESIAN_POINT ( 'NONE',  ( -11.22905947253953762, -10.35317575229728781, 319.0000000000003979 ) ) ;
#1206=CARTESIAN_POINT ( 'NONE',  ( -18.70579689905999032, -4.435290649195002821, 191.1197171614399792 ) ) ;
#1210=CARTESIAN_POINT ( 'NONE',  ( 17.64332610462000872, 5.892819363352002959, 191.1197171614399792 ) ) ;
#1213=CARTESIAN_POINT ( 'NONE',  ( -8.907970405212992659, 10.02857016715000604, -302.5071922382879279 ) ) ;
#1214=CARTESIAN_POINT ( 'NONE',  ( -14.87617152917998631, -8.357511890987989744, 318.8802828394900644 ) ) ;
#1216=CARTESIAN_POINT ( 'NONE',  ( -6.388932193737000276, 8.746770244069999478, 315.0848619657999734 ) ) ;
#1219=CARTESIAN_POINT ( 'NONE',  ( 7.497671121046002973, -10.44264915526000514, 190.0071920248299477 ) ) ;
#1224=CARTESIAN_POINT ( 'NONE',  ( -17.12450099635000100, 0.4005340032738999856, 314.8616023057000461 ) ) ;
#1226=FACE_OUTER_BOUND ( 'NONE', #9202, .T. ) ;
#1227=CARTESIAN_POINT ( 'NONE',  ( -8.636340573252621056, -8.171206817651018639, -315.0000000000000568 ) ) ;
#1230=CARTESIAN_POINT ( 'NONE',  ( 20.00000000000000000, 0.000000000000000000, -303.5000000000000000 ) ) ;
#1231=CARTESIAN_POINT ( 'NONE',  ( -3.689485142014396590, 9.275849510248953322, -315.0000000000000000 ) ) ;
#1232=PRODUCT ( 'Handle', 'Handle', '', ( #1399 ) ) ;
#1234=CARTESIAN_POINT ( 'NONE',  ( 17.30501060709000072, 4.528037784100006569, 190.0071920248299477 ) ) ;
#1235=CARTESIAN_POINT ( 'NONE',  ( -17.49999999911142723, 5.867334123717705907, 189.9999999999995453 ) ) ;
#1237=CARTESIAN_POINT ( 'NONE',  ( -4.878402812341999351, -11.12254092566999830, -317.5000000000000000 ) ) ;
#1241=CARTESIAN_POINT ( 'NONE',  ( 4.462202093987085227, -9.163742891420229242, 315.0000000000000000 ) ) ;
#1242=CARTESIAN_POINT ( 'NONE',  ( -4.001463906138999604, 9.408458373209999337, -314.8616023057000461 ) ) ;
#1244=CARTESIAN_POINT ( 'NONE',  ( -16.99996037728000076, 1.352916227065999958E-09, 314.9999801883000146 ) ) ;
#1246=DIRECTION ( 'NONE',  ( 0.000000000000000000, 0.000000000000000000, -1.000000000000000000 ) ) ;
#1248=CARTESIAN_POINT ( 'NONE',  ( 13.31532601970998897, 8.047348965112000485, -317.4928077629770087 ) ) ;
#1249=CARTESIAN_POINT ( 'NONE',  ( 0.2369326581469002602, -12.59441454048000608, -317.0792622552969533 ) ) ;
#1251=CARTESIAN_POINT ( 'NONE',  ( 0.9204674644685802987, 9.999779064329263889, -314.4999424967811024 ) ) ;
#1254=CARTESIAN_POINT ( 'NONE',  ( 11.72056399716000108, -9.035224326960999974, 190.0000000000000000 ) ) ;
#1255=CARTESIAN_POINT ( 'NONE',  ( -17.65399305443192191, -5.890951312620556379, 319.0000000000003979 ) ) ;
#1258=CARTESIAN_POINT ( 'NONE',  ( 9.011282031845993856, -11.16162715973000097, 191.1197171614399792 ) ) ;
#1261=CARTESIAN_POINT ( 'NONE',  ( 11.26120837094999594, -9.120087085473000954, -302.5071922382879279 ) ) ;
#1267=CARTESIAN_POINT ( 'NONE',  ( -18.70581557644998938, -4.435354026251000725, 318.8802828394900644 ) ) ;
#1268=CARTESIAN_POINT ( 'NONE',  ( 15.43693218238999876, -4.538485726840999490, -314.6383426456000052 ) ) ;
#1270=CARTESIAN_POINT ( 'NONE',  ( -12.28828818102000042, 7.249309191407999897, 314.4150829855000211 ) ) ;
#1272=CARTESIAN_POINT ( 'NONE',  ( 18.87263095182001749, 0.3456903499861000983, 190.0071920248299477 ) ) ;
#1280=CARTESIAN_POINT ( 'NONE',  ( -15.35630118782766651, 4.050343336346089451, 315.0000000000000000 ) ) ;
#1281=CARTESIAN_POINT ( 'NONE',  ( 11.28781796570999951, -4.951468039558000633, -284.9999999999999432 ) ) ;
#1284=CARTESIAN_POINT ( 'NONE',  ( -2.257099744627868443, -9.415190953705950605, -315.0000000000000568 ) ) ;
#1288=CARTESIAN_POINT ( 'NONE',  ( -11.93419529315104732, 6.745200168737855329, -315.0000000000000568 ) ) ;
#1289=CARTESIAN_POINT ( 'NONE',  ( -9.985646804708002477, 10.39189181891999780, 189.9229057364800042 ) ) ;
#1293=CARTESIAN_POINT ( 'NONE',  ( -15.26883884775999967, -6.827716174106000402, -317.5000000000000000 ) ) ;
#1295=CARTESIAN_POINT ( 'NONE',  ( 16.61594764501906596, -2.013242305049250280, 315.0000000000001137 ) ) ;
#1296=CARTESIAN_POINT ( 'NONE',  ( -14.28417481768999941, 5.042936695466000430, -315.0848619657999734 ) ) ;
#1297=DIRECTION ( 'NONE',  ( 0.000000000000000000, 0.000000000000000000, -1.000000000000000000 ) ) ;
#1298=CARTESIAN_POINT ( 'NONE',  ( 18.35207017878000357, 4.220106527025000887, 320.0770942683900557 ) ) ;
#1302=CARTESIAN_POINT ( 'NONE',  ( -18.93734960604998463, 3.176822791883000985, -317.5770954168139610 ) ) ;
#1304=CARTESIAN_POINT ( 'NONE',  ( 19.97263891460998764, 0.5563097477957001935, -316.3802825947000201 ) ) ;
#1307=PLANE ( 'NONE',  #8112 ) ;
#1312=CARTESIAN_POINT ( 'NONE',  ( -12.03935733796000562, -9.983683518723006856, 191.1197171614399792 ) ) ;
#1313=ORIENTED_EDGE ( 'NONE', *, *, #3388, .F. ) ;
#1315=CARTESIAN_POINT ( 'NONE',  ( 11.54867409098999964, -9.757628671089998207, -302.4229045757450081 ) ) ;
#1319=CARTESIAN_POINT ( 'NONE',  ( -19.21835421908001607, -3.675208614194998447, 319.5792614743400009 ) ) ;
#1321=CARTESIAN_POINT ( 'NONE',  ( -16.28527389671999970, 3.844447514156999812, 314.4150829855000211 ) ) ;
#1323=CARTESIAN_POINT ( 'NONE',  ( -18.21004088691051948, -5.189404274100755110, 190.9999999999995737 ) ) ;
#1325=CARTESIAN_POINT ( 'NONE',  ( -19.97284803234999018, -0.5555888903174002191, 318.8802828394900644 ) ) ;
#1329=CARTESIAN_POINT ( 'NONE',  ( -19.00000000000000000, 0.000000000000000000, 190.0000000000100044 ) ) ;
#1330=CARTESIAN_POINT ( 'NONE',  ( 0.000000000000000000, 10.00000000000000000, 315.0000000000000000 ) ) ;
#1331=VECTOR ( 'NONE', #7819, 1000.000000000000000 ) ;
#1333=CARTESIAN_POINT ( 'NONE',  ( -10.25126261553517537, 10.00000004282989785, 314.9999999999999432 ) ) ;
#1334=CARTESIAN_POINT ( 'NONE',  ( -16.78721195431734614, -1.718634075882268908, -314.9999999999999432 ) ) ;
#1337=CARTESIAN_POINT ( 'NONE',  ( 11.71572875054933327, 12.50000000135959688, -316.5000000000000000 ) ) ;
#1339=CARTESIAN_POINT ( 'NONE',  ( 2.257099744627868443, 9.415190953705950605, -315.0000000000000568 ) ) ;
#1340=CARTESIAN_POINT ( 'NONE',  ( 19.11670425725001010, 2.646693943201001264, 189.9229057364800042 ) ) ;
#1346=CARTESIAN_POINT ( 'NONE',  ( 4.578954556310520729, -9.145511589803685837, 315.0000000000000000 ) ) ;
#1347=CARTESIAN_POINT ( 'NONE',  ( -13.24479143485999977, 5.858166912337999577, -315.0848619657999734 ) ) ;
#1349=CARTESIAN_POINT ( 'NONE',  ( -9.425113983963564479, -8.435516021358374417, 314.4999463140480884 ) ) ;
#1350=CARTESIAN_POINT ( 'NONE',  ( 19.38188031595998595, 1.781951755297001450, 320.0770942683900557 ) ) ;
#1354=CARTESIAN_POINT ( 'NONE',  ( 19.60172830838999047, 0.3498260303710997721, -317.5770954168139610 ) ) ;
#1355=CARTESIAN_POINT ( 'NONE',  ( -4.990336260259995882, -12.19640393417999036, -317.0792622552969533 ) ) ;
#1357=CARTESIAN_POINT ( 'NONE',  ( 12.98706127646999953, -6.788989183774999603, -315.0000000000000000 ) ) ;
#1360=CARTESIAN_POINT ( 'NONE',  ( -10.77777196380999847, 9.457622649256999026, 190.0000000000000000 ) ) ;
#1366=CARTESIAN_POINT ( 'NONE',  ( 1.669669261120717341, -9.454727574740482865, 315.0000000000000568 ) ) ;
#1367=CARTESIAN_POINT ( 'NONE',  ( 1.652129430310999236, -12.05325387113999014, -302.4229045757450081 ) ) ;
#1371=CARTESIAN_POINT ( 'NONE',  ( -19.56025181625999920, -0.5259968871555997794, -302.4229045757450081 ) ) ;
#1372=CARTESIAN_POINT ( 'NONE',  ( 20.00506338957998409, -0.1012955751877999966, 318.8802828394900644 ) ) ;
#1374=CARTESIAN_POINT ( 'NONE',  ( 3.971626792229000280, -9.186906450543000702, -315.0848619657999734 ) ) ;
#1376=VERTEX_POINT ( 'NONE', #8009 ) ;
#1377=CARTESIAN_POINT ( 'NONE',  ( 19.37206517509000037, -1.821913627144001735, 189.9229057364800042 ) ) ;
#1378=CARTESIAN_POINT ( 'NONE',  ( 3.204766135845001696, 12.34903855201999079, 318.8802828394900644 ) ) ;
#1383=CARTESIAN_POINT ( 'NONE',  ( -1.257430124576000008, -9.427442400486999219, 315.0848619657999734 ) ) ;
#1386=CARTESIAN_POINT ( 'NONE',  ( -14.96969266857001557, -6.905075921034003805, 319.9928079742500131 ) ) ;
#1387=CARTESIAN_POINT ( 'NONE',  ( -9.217250738626699302, -7.977707550455783725, -315.0000000000001137 ) ) ;
#1388=( BOUNDED_CURVE ( )  B_SPLINE_CURVE ( 3, ( #590, #8321, #2631, #3325, #1008, #5955, #850, #7410, #1661, #2469, #6659, #4936, #4348, #6711, #5146, #8422, #4189, #9078, #2687, #5894, #1062, #9245, #6770, #9935, #5737, #8372, #9989, #1875, #7621, #8264, #956, #7568, #267, #1768, #8212, #213, #52, #157, #3544 ),
 .UNSPECIFIED., .F., .F. ) 
 B_SPLINE_CURVE_WITH_KNOTS ( ( 4, 1, 1, 1, 1, 1, 1, 1, 1, 1, 1, 1, 1, 1, 1, 1, 1, 1, 1, 1, 1, 1, 1, 1, 1, 1, 1, 1, 1, 1, 1, 1, 1, 1, 1, 1, 4 ),
 ( 0.000000000000000000, 0.03255837131920315264, 0.06556990764360211277, 0.09473136908033905068, 0.1200161462726948014, 0.1434330934855738426, 0.1672842806195496690, 0.1914679751100890059, 0.2155028411842019598, 0.2393474010340431446, 0.2632466635524260967, 0.2878286224669093785, 0.3134478398786056386, 0.3397600561265990970, 0.3667240395490956595, 0.3951494960372031184, 0.4259522906035831391, 0.4599907034545276385, 0.4966508108602696869, 0.5336723842619190972, 0.5687290606137788140, 0.6006810251919935117, 0.6302097713864018846, 0.6581574700887727891, 0.6853091452815192053, 0.7117521918490830046, 0.7371786555985279099, 0.7617219361653213561, 0.7857512081544899551, 0.8096666007474261351, 0.8337748265625606336, 0.8576111943424252759, 0.8809858201129860955, 0.9062047945899976975, 0.9352885204660792429, 0.9682251798361949380, 1.000000000000000000 ),
 .UNSPECIFIED. ) 
 CURVE ( )  GEOMETRIC_REPRESENTATION_ITEM ( )  RATIONAL_B_SPLINE_CURVE ( ( 1.171573374054913907, 1.171573374054913685, 1.171573374054913685, 1.171573374054913685, 1.171573374054913685, 1.171573374054913685, 1.171573374054913685, 1.171573374054913685, 1.171573374054913685, 1.171573374054913685, 1.171573374054913685, 1.171573374054913685, 1.171573374054913685, 1.171573374054913685, 1.171573374054913685, 1.171573374054913685, 1.171573374054913685, 1.171573374054913685, 1.171573374054913685, 1.171573374054913685, 1.171573374054913685, 1.171573374054913685, 1.171573374054913685, 1.171573374054913685, 1.171573374054913685, 1.171573374054913685, 1.171573374054913685, 1.171573374054913685, 1.171573374054913685, 1.171573374054913685, 1.171573374054913685, 1.171573374054913685, 1.171573374054913685, 1.171573374054913685, 1.171573374054913685, 1.171573374054913685, 1.171573374054913685, 1.171573374054913685, 1.171573374054913685 ) ) 
 REPRESENTATION_ITEM ( '' )  );
#1393=CARTESIAN_POINT ( 'NONE',  ( -8.691431531408321476, 8.152829611300951740, -315.0000000000000000 ) ) ;
#1394=CARTESIAN_POINT ( 'NONE',  ( -20.04238130943000940, 0.9501178419093005978, 190.4207385301700128 ) ) ;
#1395=CARTESIAN_POINT ( 'NONE',  ( 10.00000000000000000, -2.500000000000000000, -317.5000000000000000 ) ) ;
#1396=VERTEX_POINT ( 'NONE', #1395 ) ;
#1397=CARTESIAN_POINT ( 'NONE',  ( -13.35645252658000004, -8.162105094466999944, -317.5000000000000000 ) ) ;
#1398=FACE_OUTER_BOUND ( 'NONE', #118, .T. ) ;
#1399=PRODUCT_CONTEXT ( 'NONE', #1051, 'mechanical' ) ;
#1400=CARTESIAN_POINT ( 'NONE',  ( 10.02519493912904380, -7.672398658596809362, 315.0000000000000568 ) ) ;
#1401=CARTESIAN_POINT ( 'NONE',  ( -1.388768300183999882, 9.421618921053999784, -315.0848619657999734 ) ) ;
#1404=CARTESIAN_POINT ( 'NONE',  ( 20.05691220054001178, -0.5621708077868997622, 319.5792614743400009 ) ) ;
#1408=CARTESIAN_POINT ( 'NONE',  ( 12.61362476840000113, 9.241140244908006451, -317.5770954168139610 ) ) ;
#1409=CARTESIAN_POINT ( 'NONE',  ( 20.01697452336999561, -0.3413909698088000710, -316.3802825947000201 ) ) ;
#1412=CARTESIAN_POINT ( 'NONE',  ( -17.19853431800999743, -2.231396706187000145, -315.0000000000000000 ) ) ;
#1417=CARTESIAN_POINT ( 'NONE',  ( -15.54698342962807089, -4.499693933759679076, -314.5711572504542346 ) ) ;
#1420=ORIENTED_EDGE ( 'NONE', *, *, #7521, .T. ) ;
#1421=CARTESIAN_POINT ( 'NONE',  ( -8.673721998911229747, -8.158754989085133857, 315.0000000000000568 ) ) ;
#1422=CARTESIAN_POINT ( 'NONE',  ( -19.60176101890002442, -0.3495461351719001408, -302.4229045757450081 ) ) ;
#1423=EDGE_CURVE ( 'NONE', #3853, #189, #8964, .T. ) ;
#1427=CARTESIAN_POINT ( 'NONE',  ( 16.90094380520001849, 6.817658119454999444, -302.9207377450070453 ) ) ;
#1430=CARTESIAN_POINT ( 'NONE',  ( -10.32396869588999877, -7.471487098147999717, -315.0848619657999734 ) ) ;
#1431=DIRECTION ( 'NONE',  ( -5.231093336277999443E-11, -3.356106971682999882E-12, 1.000000000000000000 ) ) ;
#1433=CARTESIAN_POINT ( 'NONE',  ( 6.317945743273003956, -11.44290306353000730, 189.9229057364800042 ) ) ;
#1434=CARTESIAN_POINT ( 'NONE',  ( -17.01113700077726776, 6.587853872568209646, 190.9999999999996589 ) ) ;
#1436=EDGE_CURVE ( 'NONE', #7676, #4804, #4600, .T. ) ;
#1438=CARTESIAN_POINT ( 'NONE',  ( -13.56771446467999986, -6.451120369226999607, 314.4150829855000211 ) ) ;
#1440=CARTESIAN_POINT ( 'NONE',  ( 14.26294315260000012, 7.573769859179999564, 320.0000000000000000 ) ) ;
#1441=CARTESIAN_POINT ( 'NONE',  ( -18.85507443398999428, -0.7700411122678003650, 319.9928079742500131 ) ) ;
#1443=CARTESIAN_POINT ( 'NONE',  ( 19.96236207922240879, 0.9438262771025343056, 319.0000000000005116 ) ) ;
#1445=CARTESIAN_POINT ( 'NONE',  ( 7.006889269069000115, 6.844138725329000472, 315.0000000000000000 ) ) ;
#1448=CARTESIAN_POINT ( 'NONE',  ( -20.00000000000000000, -4.642018570833219964E-09, -303.5000000000000000 ) ) ;
#1451=CARTESIAN_POINT ( 'NONE',  ( -19.56033241475001816, -0.5267183861394004740, 189.9229057364800042 ) ) ;
#1452=CARTESIAN_POINT ( 'NONE',  ( 16.24790196670450015, 3.755744802056943499, 314.4999487198771249 ) ) ;
#1455=CARTESIAN_POINT ( 'NONE',  ( -20.00000000068207129, -7.322330470855613171, -303.4999999999999432 ) ) ;
#1459=CARTESIAN_POINT ( 'NONE',  ( 11.84516230667378345, 6.793967159201454997, 315.0000000000000568 ) ) ;
#1461=CARTESIAN_POINT ( 'NONE',  ( -10.54003729909880605, -10.63540770771157717, -303.4999999999996589 ) ) ;
#1464=CARTESIAN_POINT ( 'NONE',  ( 12.03361782604000219, 9.527744202155000508, 320.0770942683900557 ) ) ;
#1468=CARTESIAN_POINT ( 'NONE',  ( -10.62478234909000285, 10.68521885564000051, -317.0792622552969533 ) ) ;
#1469=CARTESIAN_POINT ( 'NONE',  ( 17.73927626374001676, -5.796814996629003680, -316.3802825947000201 ) ) ;
#1470=ADVANCED_FACE ( 'NONE', ( #3926 ), #5434, .T. ) ;
#1471=EDGE_LOOP ( 'NONE', ( #1192, #1313, #4177, #3745 ) ) ;
#1472=CARTESIAN_POINT ( 'NONE',  ( -17.35388116884000098, -4.663644590058999562, 320.0000000000000000 ) ) ;
#1478=CARTESIAN_POINT ( 'NONE',  ( 17.61684826078804278, -5.934684944789437644, 319.0000000000003979 ) ) ;
#1482=( BOUNDED_CURVE ( )  B_SPLINE_CURVE ( 3, ( #8611, #5240, #10132, #1156, #7813, #7714, #5658, #3895, #10443, #5549, #5443, #6255, #9752, #9588, #4059, #7174, #779, #4864, #3084, #10391, #1587, #8029, #3031, #9536, #6304, #9699, #8083, #2230, #2978, #674, #5497, #725, #2176, #6361, #4759, #7981, #2392, #8721, #9642 ),
 .UNSPECIFIED., .F., .F. ) 
 B_SPLINE_CURVE_WITH_KNOTS ( ( 4, 1, 1, 1, 1, 1, 1, 1, 1, 1, 1, 1, 1, 1, 1, 1, 1, 1, 1, 1, 1, 1, 1, 1, 1, 1, 1, 1, 1, 1, 1, 1, 1, 1, 1, 1, 4 ),
 ( 0.000000000000000000, 0.03177462182248489558, 0.06473445752888679072, 0.09385364856954797608, 0.1191010430400941816, 0.1424790257418306616, 0.1662901096498164977, 0.1904342604133075489, 0.2144298290992794898, 0.2382345388122185659, 0.2620932284128461021, 0.2866356387947041062, 0.3122179111685363662, 0.3384928023102437566, 0.3654153534982620410, 0.3937977678961499528, 0.4245599715672165320, 0.4585656223635951600, 0.4952131905531246825, 0.5322445193856788492, 0.5673324073471925910, 0.5993259174520088051, 0.6288994963735404786, 0.6568908825538778418, 0.6840816459652386827, 0.7105624348628037934, 0.7360296225686679961, 0.7606150911898691414, 0.7846847747132009721, 0.8086388669220148095, 0.8327860209783324308, 0.8566619651612987774, 0.8800749352578085549, 0.9053303401216608037, 0.9344548807899610843, 0.9674420121560727281, 1.000000000000000000 ),
 .UNSPECIFIED. ) 
 CURVE ( )  GEOMETRIC_REPRESENTATION_ITEM ( )  RATIONAL_B_SPLINE_CURVE ( ( 1.171573374019466041, 1.171573374019466263, 1.171573374019466041, 1.171573374019466263, 1.171573374019466263, 1.171573374019466263, 1.171573374019466263, 1.171573374019466263, 1.171573374019466263, 1.171573374019466263, 1.171573374019466263, 1.171573374019466263, 1.171573374019466263, 1.171573374019466263, 1.171573374019466263, 1.171573374019466263, 1.171573374019466263, 1.171573374019466263, 1.171573374019466263, 1.171573374019466263, 1.171573374019466263, 1.171573374019466263, 1.171573374019466263, 1.171573374019466263, 1.171573374019466263, 1.171573374019466263, 1.171573374019466263, 1.171573374019466263, 1.171573374019466263, 1.171573374019466263, 1.171573374019466263, 1.171573374019466263, 1.171573374019466263, 1.171573374019466263, 1.171573374019466263, 1.171573374019466263, 1.171573374019466263, 1.171573374019466263, 1.171573374019466263 ) ) 
 REPRESENTATION_ITEM ( '' )  );
#1483=CARTESIAN_POINT ( 'NONE',  ( -10.54280934634114786, -7.451587612377529091, 315.0000000000000000 ) ) ;
#1484=CARTESIAN_POINT ( 'NONE',  ( -11.53197558896999020, -9.764383963115998100, -302.4229045757450081 ) ) ;
#1487=CARTESIAN_POINT ( 'NONE',  ( -1.678162365823997915, 12.55068027652000140, -302.9207377450070453 ) ) ;
#1488=CARTESIAN_POINT ( 'NONE',  ( 4.392607225559004291, -12.20457772578000366, 318.8802828394900644 ) ) ;
#1490=CARTESIAN_POINT ( 'NONE',  ( -12.21495827233999876, -7.290170534263999969, -314.4150829855000211 ) ) ;
#1494=CARTESIAN_POINT ( 'NONE',  ( -13.35558048726000635, -8.018799577237007981, 190.0071920248299477 ) ) ;
#1495=CARTESIAN_POINT ( 'NONE',  ( 18.71194885756699833, 4.439033925638975475, 190.9999999999996589 ) ) ;
#1497=CARTESIAN_POINT ( 'NONE',  ( -6.322301096779000318, -8.991223814764000011, 314.8616023057000461 ) ) ;
#1499=CARTESIAN_POINT ( 'NONE',  ( -4.345375235838000449, 11.20786428128000090, 320.0000000000000000 ) ) ;
#1500=CARTESIAN_POINT ( 'NONE',  ( 10.54985698513999637, -9.422913819601998142, 319.9928079742500131 ) ) ;
#1501=CARTESIAN_POINT ( 'NONE',  ( -16.30951479290585837, 7.248637510199256617, 319.0000000000005116 ) ) ;
#1503=CARTESIAN_POINT ( 'NONE',  ( 16.90189876424999937, -0.3838616842170000099, 315.0848619657999734 ) ) ;
#1507=CARTESIAN_POINT ( 'NONE',  ( 18.35205128653998230, 4.220047386950002810, 189.9229057364800042 ) ) ;
#1512=CARTESIAN_POINT ( 'NONE',  ( 14.02825138570089081, 5.340904894142199488, 315.0000000000000568 ) ) ;
#1515=CARTESIAN_POINT ( 'NONE',  ( -17.62021515802999971, -4.315182425209999728, -302.4999999999969873 ) ) ;
#1516=CARTESIAN_POINT ( 'NONE',  ( -18.75085780967000559, 3.496151560526002289, 320.0770942683900557 ) ) ;
#1520=CARTESIAN_POINT ( 'NONE',  ( -19.60211473220001110, 0.3233313581039002904, -317.5770954168139610 ) ) ;
#1522=CARTESIAN_POINT ( 'NONE',  ( 7.333949653644999955, -10.60950709473999964, 320.0000000000000000 ) ) ;
#1524=CARTESIAN_POINT ( 'NONE',  ( 16.99964540243389521, -0.4333634660859933541, -315.0000000000000000 ) ) ;
#1526=CARTESIAN_POINT ( 'NONE',  ( 13.88765719697804180, -9.006220412848989554, 319.0000000000003979 ) ) ;
#1531=CARTESIAN_POINT ( 'NONE',  ( -2.737043330023148258, -9.374968016864249520, 315.0000000000000568 ) ) ;
#1532=CARTESIAN_POINT ( 'NONE',  ( -8.052748353536003378, -11.53355103076000532, -302.9207377450070453 ) ) ;
#1536=SURFACE_STYLE_FILL_AREA ( #6642 ) ;
#1540=CARTESIAN_POINT ( 'NONE',  ( 11.53197558896999020, 9.764383963115998100, -302.4229045757450081 ) ) ;
#1541=CARTESIAN_POINT ( 'NONE',  ( 6.038923639677001631, -11.92375595181999870, 318.8802828394900644 ) ) ;
#1543=CARTESIAN_POINT ( 'NONE',  ( 6.388932193737000276, -8.746770244069999478, -315.0848619657999734 ) ) ;
#1546=CARTESIAN_POINT ( 'NONE',  ( 19.56033241475001816, 0.5267183861393005539, 189.9229057364800042 ) ) ;
#1548=CARTESIAN_POINT ( 'NONE',  ( 10.00000000000000000, 2.500000000000000000, -317.5000000000000000 ) ) ;
#1550=EDGE_CURVE ( 'NONE', #2509, #9430, #5096, .T. ) ;
#1551=CARTESIAN_POINT ( 'NONE',  ( -10.32396869588999877, -7.471487098147999717, 315.0848619657999734 ) ) ;
#1556=LINE ( 'NONE', #8003, #4345 ) ;
#1557=CARTESIAN_POINT ( 'NONE',  ( -1.514431797236434930E-09, -10.00000000000000000, -302.4999999999999432 ) ) ;
#1565=CARTESIAN_POINT ( 'NONE',  ( -17.16660215780892784, -1.253874176888070540E-08, -314.8332688233516024 ) ) ;
#1567=CARTESIAN_POINT ( 'NONE',  ( 18.56827417761491361, -4.704550062028092228, -303.4999999999996589 ) ) ;
#1568=CARTESIAN_POINT ( 'NONE',  ( -10.18931492271999950, -9.698324433322001781, -302.5000000000000000 ) ) ;
#1571=CARTESIAN_POINT ( 'NONE',  ( -17.67524584885999772, 5.985122643679996912, 319.5792614743400009 ) ) ;
#1573=CARTESIAN_POINT ( 'NONE',  ( 13.57573464316000056, 3.225916527208000151, 315.0000000000001705 ) ) ;
#1575=CARTESIAN_POINT ( 'NONE',  ( -19.98286815278001427, -0.4166756924005995955, -316.3802825947000201 ) ) ;
#1579=CARTESIAN_POINT ( 'NONE',  ( 17.34782881681000077, -4.671787541421999812, 320.0000000000000000 ) ) ;
#1585=CARTESIAN_POINT ( 'NONE',  ( 19.99997414083856739, -0.3194320646935533969, 319.0000000000003979 ) ) ;
#1587=CARTESIAN_POINT ( 'NONE',  ( 1.602145841528213932, 12.47735433440135644, -316.5000000000004547 ) ) ;
#1589=CARTESIAN_POINT ( 'NONE',  ( 0.9841565935054803482, -9.488387273935385835, 314.9999999999999432 ) ) ;
#1590=CARTESIAN_POINT ( 'NONE',  ( 19.31742247159998271, -3.345204157467998929, -303.6197174156509391 ) ) ;
#1596=( NAMED_UNIT ( * ) SI_UNIT ( $, .STERADIAN. ) SOLID_ANGLE_UNIT ( ) );
#1597=CARTESIAN_POINT ( 'NONE',  ( 3.644643686525998572, 11.88155656384000203, -302.4229045757450081 ) ) ;
#1598=CARTESIAN_POINT ( 'NONE',  ( 13.88394749849000043, -9.000054837070988967, 318.8802828394900644 ) ) ;
#1600=CARTESIAN_POINT ( 'NONE',  ( -1.276003512426000075, -9.874146089817999794, -314.6383426456000052 ) ) ;
#1601=CARTESIAN_POINT ( 'NONE',  ( 16.13341719193999779, 6.058597787994999706, -302.5000000000000000 ) ) ;
#1604=CARTESIAN_POINT ( 'NONE',  ( -17.75414941409001557, -3.856242593410000197, 190.0071920248299477 ) ) ;
#1606=CARTESIAN_POINT ( 'NONE',  ( -13.64075175739777102, 5.653800323622448332, -315.0000000000000568 ) ) ;
#1608=CARTESIAN_POINT ( 'NONE',  ( -14.52969073417999901, -5.422537850045999974, 314.6383426456000052 ) ) ;
#1610=CARTESIAN_POINT ( 'NONE',  ( -16.83239583074999857, 5.311267823799999732, 320.0000000000000000 ) ) ;
#1612=CARTESIAN_POINT ( 'NONE',  ( 17.65399305443192901, 5.890951312620557268, 319.0000000000005116 ) ) ;
#1614=CARTESIAN_POINT ( 'NONE',  ( 15.00000000000000000, 0.4945770392355999800, 315.0000000000000000 ) ) ;
#1616=CARTESIAN_POINT ( 'NONE',  ( 13.57573464316000056, 3.225916527208000151, -285.0000000000000000 ) ) ;
#1622=CARTESIAN_POINT ( 'NONE',  ( -1.984036549750167078, -12.45525792938212284, -303.4999999999996589 ) ) ;
#1623=CARTESIAN_POINT ( 'NONE',  ( 17.34089965840999881, 0.6440164457022999889, -314.6383426456000052 ) ) ;
#1628=CARTESIAN_POINT ( 'NONE',  ( -0.2363117521398999110, 12.51008298726001300, -316.3802825947000201 ) ) ;
#1632=CARTESIAN_POINT ( 'NONE',  ( -16.84305512206999822, -5.298470530761999697, 320.0000000000000000 ) ) ;
#1634=UNCERTAINTY_MEASURE_WITH_UNIT (LENGTH_MEASURE( 1.000000000000000082E-05 ), #4296, 'distance_accuracy_value', 'NONE');
#1636=CARTESIAN_POINT ( 'NONE',  ( 16.39029893813008343, -2.501810464458257943, -315.0000000000000568 ) ) ;
#1637=ORIENTED_EDGE ( 'NONE', *, *, #8378, .T. ) ;
#1638=CARTESIAN_POINT ( 'NONE',  ( 6.348506474365276375, -9.305625771097021826, -314.5281326612879411 ) ) ;
#1640=DIRECTION ( 'NONE',  ( 0.000000000000000000, 0.000000000000000000, 1.000000000000000000 ) ) ;
#1642=CARTESIAN_POINT ( 'NONE',  ( 20.01694242003000568, -0.3416920405409001327, -303.6197174156509391 ) ) ;
#1645=CARTESIAN_POINT ( 'NONE',  ( -12.89386942443999295, 9.656754267509002787, -302.9207377450070453 ) ) ;
#1646=CARTESIAN_POINT ( 'NONE',  ( -17.49999996772987743, -5.857864456328762515, 314.4997059534069308 ) ) ;
#1648=DIRECTION ( 'NONE',  ( -0.000000000000000000, 1.000000000000000000, 0.000000000000000000 ) ) ;
#1649=CARTESIAN_POINT ( 'NONE',  ( 7.774319915545000015, 10.49237824600999858, -302.5000000000000000 ) ) ;
#1651=CARTESIAN_POINT ( 'NONE',  ( -10.00032506892000406, -10.91649673191999526, 190.4207385301700128 ) ) ;
#1653=CARTESIAN_POINT ( 'NONE',  ( 13.95711901494857443, 5.398584340276486593, -315.0000000000000568 ) ) ;
#1656=CARTESIAN_POINT ( 'NONE',  ( 17.21448334449999962, -1.351716521078000222, 314.6383426456000052 ) ) ;
#1658=CARTESIAN_POINT ( 'NONE',  ( -17.34782881681000077, 4.671787541421999812, 320.0000000000000000 ) ) ;
#1659=CARTESIAN_POINT ( 'NONE',  ( 7.392698694382005442, -11.19283382348000622, 320.0770942683900557 ) ) ;
#1660=CARTESIAN_POINT ( 'NONE',  ( -9.914941699848355938, 10.86515064494810545, 319.0000000000005116 ) ) ;
#1661=CARTESIAN_POINT ( 'NONE',  ( 14.92864611359688531, 8.336576156742356858, -303.4999999999990905 ) ) ;
#1672=CARTESIAN_POINT ( 'NONE',  ( 16.90189876424999937, -0.3838616842170000099, -315.0848619657999734 ) ) ;
#1676=CARTESIAN_POINT ( 'NONE',  ( 11.28781796570999951, 4.951468039558000633, 315.0000000000001705 ) ) ;
#1679=CARTESIAN_POINT ( 'NONE',  ( -17.73927626374001676, 5.796814996629003680, -316.3802825947000201 ) ) ;
#1681=CARTESIAN_POINT ( 'NONE',  ( -18.20902923167000154, -3.282017551273999967, 320.0000000000000000 ) ) ;
#1686=CARTESIAN_POINT ( 'NONE',  ( 4.648899539349734766, -9.134382686408038410, -315.0000000000001137 ) ) ;
#1687=ORIENTED_EDGE ( 'NONE', *, *, #5354, .F. ) ;
#1688=CARTESIAN_POINT ( 'NONE',  ( -17.19853431801041665, 2.231396706186351775, -315.0000000000001137 ) ) ;
#1692=CARTESIAN_POINT ( 'NONE',  ( 19.39478698591998551, -3.379789856048000196, -302.9207377450070453 ) ) ;
#1693=CARTESIAN_POINT ( 'NONE',  ( 18.86306334786000605, 0.4771235332119000971, -317.4928077629770087 ) ) ;
#1698=CARTESIAN_POINT ( 'NONE',  ( 9.312701725069002734, 11.06649994634999246, -303.6197174156509391 ) ) ;
#1699=CARTESIAN_POINT ( 'NONE',  ( -10.00000000000000000, -2.500000000000000000, -317.5000000000000000 ) ) ;
#1700=ORIENTED_EDGE ( 'NONE', *, *, #9251, .F. ) ;
#1703=ORIENTED_EDGE ( 'NONE', *, *, #9636, .T. ) ;
#1704=CARTESIAN_POINT ( 'NONE',  ( -20.08919666923998903, -0.07462331497648995449, 190.4207385301700128 ) ) ;
#1705=CARTESIAN_POINT ( 'NONE',  ( 17.50000000000126832, -0.7437989020612977287, -314.4944826805096341 ) ) ;
#1706=CARTESIAN_POINT ( 'NONE',  ( 16.34919249956382714, 2.583378889817198765, -314.9999999999999432 ) ) ;
#1708=CARTESIAN_POINT ( 'NONE',  ( -6.420662313211997763, 11.93024803506000531, 190.4207385301700128 ) ) ;
#1712=CARTESIAN_POINT ( 'NONE',  ( 17.56758064089999749, -0.6313722887073999201, 314.4150829855000211 ) ) ;
#1714=CARTESIAN_POINT ( 'NONE',  ( 19.54690800120000205, -0.8885403386512999990, 320.0770942683900557 ) ) ;
#1716=CARTESIAN_POINT ( 'NONE',  ( 10.58801790939999954, 8.088125079530000150, 314.4150829855000211 ) ) ;
#1721=VECTOR ( 'NONE', #836, 1000.000000000000000 ) ;
#1724=CARTESIAN_POINT ( 'NONE',  ( 2.450606348566487735, 9.399923241459493539, 315.0000000000000568 ) ) ;
#1732=CARTESIAN_POINT ( 'NONE',  ( -3.762811461229003562, 12.28417267642999278, -316.3802825947000201 ) ) ;
#1737=CARTESIAN_POINT ( 'NONE',  ( 16.37727794820371940, -2.527950228764472396, -315.0000000000001137 ) ) ;
#1741=EDGE_LOOP ( 'NONE', ( #6927, #2531 ) ) ;
#1742=CARTESIAN_POINT ( 'NONE',  ( -12.36094278317000139, 8.718445687105001340, -317.5000000000000000 ) ) ;
#1745=CARTESIAN_POINT ( 'NONE',  ( -19.29864983862999850, -3.387441872937999143, -303.6197174156520759 ) ) ;
#1746=CARTESIAN_POINT ( 'NONE',  ( 18.21319838702001448, -4.476589323548002319, -317.5770954168139610 ) ) ;
#1756=CARTESIAN_POINT ( 'NONE',  ( -17.08426003144000305, -6.624354047749995367, 190.4207385301700128 ) ) ;
#1761=CARTESIAN_POINT ( 'NONE',  ( -6.403271823880001712, 11.84773780780999530, 191.1197171614399792 ) ) ;
#1762=CARTESIAN_POINT ( 'NONE',  ( 16.99702983282000091, -1.298346578676000007, 314.8616023057000461 ) ) ;
#1766=CARTESIAN_POINT ( 'NONE',  ( -17.87038977196999312, -4.940238929760003117, 320.0770942683900557 ) ) ;
#1768=CARTESIAN_POINT ( 'NONE',  ( -17.74743742734689178, 5.798256014711220097, -303.5000000000000000 ) ) ;
#1769=CARTESIAN_POINT ( 'NONE',  ( 17.34710322845000263, -0.4172063223308000168, 314.6383426456000052 ) ) ;
#1771=CARTESIAN_POINT ( 'NONE',  ( -9.974269275089660880, -10.84391064191636644, 190.9999999999995737 ) ) ;
#1772=CARTESIAN_POINT ( 'NONE',  ( -12.02088824526999211, 10.08549396686999522, 319.5792614743400009 ) ) ;
#1776=CARTESIAN_POINT ( 'NONE',  ( -11.33727843270404634, 7.061073773682574384, 315.0000000000000000 ) ) ;
#1778=CARTESIAN_POINT ( 'NONE',  ( -15.00000000000000000, 0.000000000000000000, -285.0000000000000000 ) ) ;
#1783=CARTESIAN_POINT ( 'NONE',  ( 9.616122863433998802, 9.909251266138999981, 190.0000000000000000 ) ) ;
#1787=CARTESIAN_POINT ( 'NONE',  ( 1.601785992426999705, 12.47016740323998718, -316.3802825947000201 ) ) ;
#1792=CARTESIAN_POINT ( 'NONE',  ( 15.47196055635296119, -3.911380178888624215, -315.0000000000000568 ) ) ;
#1794=CARTESIAN_POINT ( 'NONE',  ( 7.237892782308166240, -9.087442202657101120, -314.5335583295243964 ) ) ;
#1797=CARTESIAN_POINT ( 'NONE',  ( 4.878402812341999351, 11.12254092566999830, -317.5000000000000000 ) ) ;
#1800=CARTESIAN_POINT ( 'NONE',  ( 16.88084019735002173, -6.719348373024005561, -303.6197174156509391 ) ) ;
#1802=CARTESIAN_POINT ( 'NONE',  ( 15.69339834701000136, -7.228928788388996551, -317.5770954168139610 ) ) ;
#1806=SHAPE_REPRESENTATION ( 'Handle', ( #2817 ), #8168 ) ;
#1808=CARTESIAN_POINT ( 'NONE',  ( 17.70828763765000247, 5.833668797872996414, -303.6197174156520759 ) ) ;
#1811=CARTESIAN_POINT ( 'NONE',  ( -16.58659719219999928, -2.947707964209000053, -314.6383426456000052 ) ) ;
#1813=CARTESIAN_POINT ( 'NONE',  ( 2.001531325394999783, 11.45199047667999892, -302.5000000000000000 ) ) ;
#1815=CARTESIAN_POINT ( 'NONE',  ( 11.20196042648000123, -10.44833032063000111, 190.4207385301700128 ) ) ;
#1816=CARTESIAN_POINT ( 'NONE',  ( 17.19853431801041665, -2.231396706186351775, -315.0000000000001137 ) ) ;
#1819=CARTESIAN_POINT ( 'NONE',  ( 19.86706274963002983, 1.898735342979001484, 190.4207385301700128 ) ) ;
#1820=CARTESIAN_POINT ( 'NONE',  ( 17.14577796628000073, -0.02050488658304000164, 314.8616023057000461 ) ) ;
#1823=CARTESIAN_POINT ( 'NONE',  ( -19.59064078059999758, -0.07061976926606000626, 320.0770942683900557 ) ) ;
#1826=CARTESIAN_POINT ( 'NONE',  ( 16.77099092997999819, 1.279831385791999843, 315.0848619657999734 ) ) ;
#1829=ORIENTED_EDGE ( 'NONE', *, *, #9368, .T. ) ;
#1830=CARTESIAN_POINT ( 'NONE',  ( -7.514439085588995759, 11.67576679883001667, 319.5792614743400009 ) ) ;
#1831=CARTESIAN_POINT ( 'NONE',  ( -15.00000000000000000, 0.000000000000000000, -285.0000000000000000 ) ) ;
#1834=CARTESIAN_POINT ( 'NONE',  ( 7.042505780985288233, 8.656073623659681360, 315.0000000000000000 ) ) ;
#1837=CARTESIAN_POINT ( 'NONE',  ( 16.15280651819000113, -6.039793344733999980, -302.5000000000000000 ) ) ;
#1838=CARTESIAN_POINT ( 'NONE',  ( 7.347903365571999856, 10.60600056872999986, 190.0000000000000000 ) ) ;
#1839=CARTESIAN_POINT ( 'NONE',  ( 17.05540563375874541, -2.295823697340080738, 314.4999398562650867 ) ) ;
#1840=CARTESIAN_POINT ( 'NONE',  ( -15.00000000000072120, 0.4945770392355430256, -284.9999999999999432 ) ) ;
#1845=CARTESIAN_POINT ( 'NONE',  ( 15.67978886374999803, 4.575336738469999887, -315.0000000000000000 ) ) ;
#1846=CARTESIAN_POINT ( 'NONE',  ( 16.03969916442340704, -3.142024325209859636, -315.0000000000000568 ) ) ;
#1848=CIRCLE ( 'NONE', #2708, 1.000000000000008882 ) ;
#1849=CARTESIAN_POINT ( 'NONE',  ( 15.67978886374999803, 4.575336738469999887, -315.0000000000001137 ) ) ;
#1850=CARTESIAN_POINT ( 'NONE',  ( -19.99999036626000048, -4.642009783819999925E-09, -316.5000000000000000 ) ) ;
#1852=CARTESIAN_POINT ( 'NONE',  ( 18.32252861763999974, 3.123808493131999597, -317.4999999999870397 ) ) ;
#1854=CARTESIAN_POINT ( 'NONE',  ( 17.60469080286000931, 4.126100741655001514, -317.4928077629770087 ) ) ;
#1855=CARTESIAN_POINT ( 'NONE',  ( -18.86307259346999032, 0.4762574081846996932, -317.4928077629770087 ) ) ;
#1859=CARTESIAN_POINT ( 'NONE',  ( -9.252434838928003558, 11.08696499602999630, -303.6197174156509391 ) ) ;
#1860=CARTESIAN_POINT ( 'NONE',  ( 10.32803372116435270, 10.00000000000000178, 315.0000000000000000 ) ) ;
#1863=CARTESIAN_POINT ( 'NONE',  ( 0.1867348994714999877, 11.51775814840000045, -302.5000000000000000 ) ) ;
#1864=VERTEX_POINT ( 'NONE', #7267 ) ;
#1865=CARTESIAN_POINT ( 'NONE',  ( 3.136708848033998187, -12.44064353863999983, 190.4207385301700128 ) ) ;
#1866=CARTESIAN_POINT ( 'NONE',  ( -15.67978886374999803, -4.575336738469999887, -315.0000000000001137 ) ) ;
#1867=CARTESIAN_POINT ( 'NONE',  ( 11.74249363970098514, 6.849480045866885192, -315.0000000000000000 ) ) ;
#1868=CARTESIAN_POINT ( 'NONE',  ( 12.07524870805000639, 10.05998438363999981, 190.4207385301700128 ) ) ;
#1871=CARTESIAN_POINT ( 'NONE',  ( 11.96281778373999849, -6.662668310474999522, 315.0848619657999734 ) ) ;
#1873=CARTESIAN_POINT ( 'NONE',  ( -12.03361782604000219, -9.527744202155000508, 320.0770942683900557 ) ) ;
#1875=CARTESIAN_POINT ( 'NONE',  ( -11.72170966038013340, 10.14138702413947968, -303.4999999999990905 ) ) ;
#1876=CARTESIAN_POINT ( 'NONE',  ( 3.846123575835999731, 9.203727088275000412, 315.0848619657999734 ) ) ;
#1878=CARTESIAN_POINT ( 'NONE',  ( 13.99679147458261141, -8.939383429014133853, 190.9999999999995737 ) ) ;
#1879=CARTESIAN_POINT ( 'NONE',  ( 11.25912153621000300, 10.42419777155999938, 319.5792614743400009 ) ) ;
#1883=CARTESIAN_POINT ( 'NONE',  ( 4.669690493011572130, 9.131031402067035785, 315.0000000000001137 ) ) ;
#1884=CARTESIAN_POINT ( 'NONE',  ( 14.79012398733999945, -1.483731117707000058, -285.0000000000000000 ) ) ;
#1887=CARTESIAN_POINT ( 'NONE',  ( 11.28854116844999922, -9.238965579841000419, -302.5000000000000000 ) ) ;
#1890=CARTESIAN_POINT ( 'NONE',  ( 17.81342281586000098, 3.988456401492999959, 190.0000000000000000 ) ) ;
#1892=CARTESIAN_POINT ( 'NONE',  ( -15.75853520210212011, 3.543431633405213610, -314.9999999999999432 ) ) ;
#1893=CARTESIAN_POINT ( 'NONE',  ( -18.87263095182001749, -0.3456903499861000983, 190.0071920248299477 ) ) ;
#1900=CARTESIAN_POINT ( 'NONE',  ( 7.560581757588001217, 10.42594579828999990, 319.9928079742500131 ) ) ;
#1902=CARTESIAN_POINT ( 'NONE',  ( 14.97237716209997416, -8.305886502593784471, -316.5000000000004547 ) ) ;
#1908=CARTESIAN_POINT ( 'NONE',  ( 19.60211473220001110, -0.3233313581039002904, -317.5770954168139610 ) ) ;
#1909=EDGE_CURVE ( 'NONE', #1864, #4012, #8125, .T. ) ;
#1912=CARTESIAN_POINT ( 'NONE',  ( -11.54127207300577496, -7.525448855209205590, 314.4999468205385256 ) ) ;
#1914=CARTESIAN_POINT ( 'NONE',  ( 13.46369163363000077, -8.092480683229998917, 190.0000000000000000 ) ) ;
#1920=CARTESIAN_POINT ( 'NONE',  ( 13.97596040350999402, 9.042973024665997173, 190.4207385301700128 ) ) ;
#1923=CARTESIAN_POINT ( 'NONE',  ( 1.279515965483999906E-07, 10.00000000755999885, 190.0000000000000000 ) ) ;
#1925=CARTESIAN_POINT ( 'NONE',  ( 17.67524584885999772, -5.985122643678997711, 319.5792614743400009 ) ) ;
#1928=CARTESIAN_POINT ( 'NONE',  ( 14.72449281369000040, -5.549439731021000632, -314.4150829855000211 ) ) ;
#1929=CARTESIAN_POINT ( 'NONE',  ( 17.42228208267999889, 1.444224815522999972, 314.4150829855000211 ) ) ;
#1931=CARTESIAN_POINT ( 'NONE',  ( 19.99999721801999897, 7.771189452710000131E-11, 191.0000000000000000 ) ) ;
#1932=CARTESIAN_POINT ( 'NONE',  ( -20.05691607070997051, -0.5615793767616999999, 319.5792614743400009 ) ) ;
#1937=CARTESIAN_POINT ( 'NONE',  ( -9.217211940708146756, 7.977736869146946574, 315.0000000000000000 ) ) ;
#1938=CARTESIAN_POINT ( 'NONE',  ( 14.79012398734008293, -1.483731117706880154, -284.9999999999999432 ) ) ;
#1939=CARTESIAN_POINT ( 'NONE',  ( 17.63021146919999893, -4.299866645372000029, -302.4999999999969873 ) ) ;
#1944=CARTESIAN_POINT ( 'NONE',  ( -16.37160231057345783, 2.539265572400264848, -315.0000000000001137 ) ) ;
#1946=CARTESIAN_POINT ( 'NONE',  ( 5.118368704603114087E-10, 10.00000000003099210, 314.4999681336588537 ) ) ;
#1953=VERTEX_POINT ( 'NONE', #7117 ) ;
#1954=CARTESIAN_POINT ( 'NONE',  ( 6.240232637630001911, 10.74449313720999832, 319.9928079742500131 ) ) ;
#1955=CARTESIAN_POINT ( 'NONE',  ( -1.602145841528213932, -12.47735433440135644, -316.5000000000004547 ) ) ;
#1956=PLANE ( 'NONE',  #2955 ) ;
#1959=CARTESIAN_POINT ( 'NONE',  ( -18.19038122738000141, -4.511441183124001775, -317.5770954168139610 ) ) ;
#1961=CARTESIAN_POINT ( 'NONE',  ( -15.60185585328000002, 4.689707898928999974, -314.4150829855000211 ) ) ;
#1964=CARTESIAN_POINT ( 'NONE',  ( 7.251913689787688355, 9.130298775770077313, -314.5336966332660040 ) ) ;
#1969=EDGE_LOOP ( 'NONE', ( #10293, #852, #7468, #7336, #5645 ) ) ;
#1970=CARTESIAN_POINT ( 'NONE',  ( -18.20422786544000715, -5.185156308378004120, 191.1197171614399792 ) ) ;
#1980=CARTESIAN_POINT ( 'NONE',  ( -14.92426358056000701, -8.426786174986000688, 319.5792614743400009 ) ) ;
#1981=B_SPLINE_CURVE_WITH_KNOTS ( 'NONE', 3,
 ( #2403, #5671, #2186, #4660, #3856, #7186, #1601, #8955, #4874, #10455, #6313, #5509, #3096, #1050, #1649, #5725, #3370, #8411, #1813, #1863, #8358, #2560, #5828, #3476, #3531, #4284, #2674, #9816, #145, #996, #2456, #4334, #7607, #9173, #6698, #9976, #2617, #7556, #201 ),
 .UNSPECIFIED., .F., .F.,
 ( 4, 1, 1, 1, 1, 1, 1, 1, 1, 1, 1, 1, 1, 1, 1, 1, 1, 1, 1, 1, 1, 1, 1, 1, 1, 1, 1, 1, 1, 1, 1, 1, 1, 1, 1, 1, 4 ),
 ( 0.000000000000000000, 0.02777777777778000015, 0.05555555555556000030, 0.08333333333333001192, 0.1111111111111000027, 0.1388888888888999973, 0.1666666666667000196, 0.1944444444444000109, 0.2222222222222000054, 0.2500000000000000000, 0.2777777777777999946, 0.3055555555555999891, 0.3333333333333000081, 0.3611111111111000027, 0.3888888888888999973, 0.4166666666666999919, 0.4444444444444000109, 0.4722222222222000054, 0.5000000000000000000, 0.5277777777777999946, 0.5555555555555999891, 0.5833333333333000637, 0.6111111111111000582, 0.6388888888888999418, 0.6666666666667000474, 0.6944444444444000109, 0.7222222222222000054, 0.7500000000000000000, 0.7777777777777999946, 0.8055555555555999891, 0.8333333333333000637, 0.8611111111111000582, 0.8888888888888999418, 0.9166666666667000474, 0.9444444444444000109, 0.9722222222222000054, 1.000000000000000000 ),
 .UNSPECIFIED. ) ;
#1983=CARTESIAN_POINT ( 'NONE',  ( -16.60805916514000202, 2.908391789136000050, 314.6383426456000052 ) ) ;
#1991=CARTESIAN_POINT ( 'NONE',  ( 7.006889269069000115, -6.844138725329000472, 315.0000000000001705 ) ) ;
#1996=CARTESIAN_POINT ( 'NONE',  ( 1.514429654104534930E-09, 10.00000000000000000, -302.5000000000000000 ) ) ;
#1997=CARTESIAN_POINT ( 'NONE',  ( 9.526067998327799539E-10, -10.00000000005854339, 314.4999528359535361 ) ) ;
#1998=CARTESIAN_POINT ( 'NONE',  ( 7.284698641071005731, 10.49877923466000063, 190.0071920248299477 ) ) ;
#2000=STYLED_ITEM ( 'NONE', ( #6479 ), #453 ) ;
#2001=CARTESIAN_POINT ( 'NONE',  ( -18.86945318303000008, -1.615078380336999908, -317.5000000000470095 ) ) ;
#2004=CARTESIAN_POINT ( 'NONE',  ( 10.90962076852776796, -7.272180451173178461, 315.0000000000000000 ) ) ;
#2005=CARTESIAN_POINT ( 'NONE',  ( 3.874983216044999956, 9.425407904674999671, -314.8616023057000461 ) ) ;
#2006=ORIENTED_EDGE ( 'NONE', *, *, #3523, .T. ) ;
#2007=CARTESIAN_POINT ( 'NONE',  ( -2.482300462934001306, 11.29873291818999803, 319.9928079742500131 ) ) ;
#2008=CARTESIAN_POINT ( 'NONE',  ( 2.055855549839187280, -12.45069410617974626, -316.5000000000004547 ) ) ;
#2011=CARTESIAN_POINT ( 'NONE',  ( -11.29610983636999144, 9.103527074753996473, -317.4928077629770087 ) ) ;
#2012=CARTESIAN_POINT ( 'NONE',  ( 20.10152810630999554, -0.3450717431897997733, -317.0792622552969533 ) ) ;
#2014=CARTESIAN_POINT ( 'NONE',  ( -16.97404422732000029, 2.118410180888999683, -314.6383426456000052 ) ) ;
#2015=DIRECTION ( 'NONE',  ( 1.000000000000000000, 0.000000000000000000, 0.000000000000000000 ) ) ;
#2017=CARTESIAN_POINT ( 'NONE',  ( -5.950428891765999317, -10.92854977363000124, 190.0000000000000000 ) ) ;
#2020=CARTESIAN_POINT ( 'NONE',  ( -16.34352199340000311, -7.209047878930006092, 191.1197171614399792 ) ) ;
#2023=CARTESIAN_POINT ( 'NONE',  ( -8.965618380443995505, -10.00899073891999436, -302.5071922382879279 ) ) ;
#2024=EDGE_CURVE ( 'NONE', #22, #8305, #5870, .T. ) ;
#2028=CARTESIAN_POINT ( 'NONE',  ( 5.068019528653000982, 10.96907295785000080, -302.5071922382879279 ) ) ;
#2029=CARTESIAN_POINT ( 'NONE',  ( -19.50549492440999089, -2.789745814424999359, 318.8802828394900644 ) ) ;
#2030=CARTESIAN_POINT ( 'NONE',  ( 16.90798586812000082, 0.2930809059028999797, -315.0848619657999734 ) ) ;
#2031=CARTESIAN_POINT ( 'NONE',  ( -16.97404422732000029, 2.118410180888999683, 314.6383426456000052 ) ) ;
#2033=CARTESIAN_POINT ( 'NONE',  ( -0.6878067384152003472, -11.39249343872000075, 190.0071920248299477 ) ) ;
#2035=CARTESIAN_POINT ( 'NONE',  ( -19.95862339310001943, 0.9382979884530006087, 318.8802828394900644 ) ) ;
#2038=CARTESIAN_POINT ( 'NONE',  ( -17.57772697299999720, 0.3191603157329000462, 314.4150829855000211 ) ) ;
#2040=CARTESIAN_POINT ( 'NONE',  ( -10.00000000000000000, -2.500000000000000000, -285.0000000000000000 ) ) ;
#2041=CARTESIAN_POINT ( 'NONE',  ( -11.72583169940718406, -6.858410958448124539, -315.0000000000000000 ) ) ;
#2044=FACE_OUTER_BOUND ( 'NONE', #8934, .T. ) ;
#2045=CARTESIAN_POINT ( 'NONE',  ( -2.545630254023276251, 9.391959925330709780, -315.0000000000000000 ) ) ;
#2046=CARTESIAN_POINT ( 'NONE',  ( 14.16528011596000169, 7.496216825914998161, 190.0071920248299477 ) ) ;
#2053=CARTESIAN_POINT ( 'NONE',  ( 14.65007096172560708, -4.807726778454477490, 314.9999999999998863 ) ) ;
#2054=CARTESIAN_POINT ( 'NONE',  ( 12.10743226551000085, 7.094093637544000686, -314.6383426456000052 ) ) ;
#2056=CARTESIAN_POINT ( 'NONE',  ( -19.30579288353658640, -3.388955136080751718, -316.5000000000004547 ) ) ;
#2060=VECTOR ( 'NONE', #9651, 1000.000000000000000 ) ;
#2062=CARTESIAN_POINT ( 'NONE',  ( -4.911540754813998433, -11.70462039183999892, -317.5770954168139610 ) ) ;
#2067=CARTESIAN_POINT ( 'NONE',  ( 16.83327205402999738, -5.309787193942999473, 190.0000000000000000 ) ) ;
#2073=CARTESIAN_POINT ( 'NONE',  ( -17.50000000000000000, 0.000000000000000000, -302.5000000000000000 ) ) ;
#2074=CARTESIAN_POINT ( 'NONE',  ( 6.297776810737998332, -10.73166643879000404, -302.5071922382879279 ) ) ;
#2080=CARTESIAN_POINT ( 'NONE',  ( 18.75338617474996994, -4.519296150162002590, 319.5792614743400009 ) ) ;
#2081=CARTESIAN_POINT ( 'NONE',  ( 15.27200851150000105, -4.387263554753999983, -314.8616023057000461 ) ) ;
#2083=CARTESIAN_POINT ( 'NONE',  ( -17.34500932694999875, 0.6070218422356999932, 314.6383426456000052 ) ) ;
#2086=CARTESIAN_POINT ( 'NONE',  ( -19.12221666159999600, 3.679580603257996962, 318.8802828394900644 ) ) ;
#2090=CARTESIAN_POINT ( 'NONE',  ( 18.95677580539999951, 0.9180370088860999589, 320.0000000000000000 ) ) ;
#2091=CARTESIAN_POINT ( 'NONE',  ( 13.57573464316000056, -3.225916527208000151, -284.9999999999999432 ) ) ;
#2092=CARTESIAN_POINT ( 'NONE',  ( -15.26192592288499483, -4.160213195839838285, -314.9999999999998863 ) ) ;
#2094=CARTESIAN_POINT ( 'NONE',  ( -17.50000000000000711, 8.653878165429867666E-10, 190.0000000000001137 ) ) ;
#2095=EDGE_CURVE ( 'NONE', #6759, #2473, #7328, .T. ) ;
#2096=CARTESIAN_POINT ( 'NONE',  ( -11.71572875797656188, 12.49999999864037825, -316.5000000000000000 ) ) ;
#2097=CARTESIAN_POINT ( 'NONE',  ( -3.024115758602054171, 9.348088905657231606, -315.0000000000000000 ) ) ;
#2100=CARTESIAN_POINT ( 'NONE',  ( 11.05317456124874553, 7.762181834020175586, 314.4999466939158879 ) ) ;
#2102=CARTESIAN_POINT ( 'NONE',  ( -14.32993508528999982, -7.533629911342000440, -317.5000000000000000 ) ) ;
#2105=CARTESIAN_POINT ( 'NONE',  ( 2.257382111677873393, -9.415175415973715545, 315.0000000000000000 ) ) ;
#2106=CARTESIAN_POINT ( 'NONE',  ( 3.846123575835999731, 9.203727088275000412, -315.0848619657999734 ) ) ;
#2109=CARTESIAN_POINT ( 'NONE',  ( -17.16661504264607885, 5.088157322090969144E-08, 314.8332817084517501 ) ) ;
#2113=CARTESIAN_POINT ( 'NONE',  ( -17.42196264042997100, 5.530423875593995398, -317.5770954168139610 ) ) ;
#2114=CARTESIAN_POINT ( 'NONE',  ( -13.67588481992999228, -8.646726704586995993, -317.5770954168139610 ) ) ;
#2119=CARTESIAN_POINT ( 'NONE',  ( -19.99999721132999753, 3.518711422920000253E-10, 319.0000000000000000 ) ) ;
#2127=CARTESIAN_POINT ( 'NONE',  ( 7.559362580479000115, 11.57734716366000072, 191.1197171614399792 ) ) ;
#2128=ADVANCED_FACE ( 'NONE', ( #2384, #3942 ), #4100, .F. ) ;
#2132=CARTESIAN_POINT ( 'NONE',  ( 19.46046181435998079, 1.651614223715000884, -302.4229045757450081 ) ) ;
#2133=CARTESIAN_POINT ( 'NONE',  ( -18.27279225368999249, -5.234253896328004529, 319.5792614743400009 ) ) ;
#2135=CARTESIAN_POINT ( 'NONE',  ( -13.37260572687999982, 6.041714840053000302, 314.8616023057000461 ) ) ;
#2137=CARTESIAN_POINT ( 'NONE',  ( -19.99999721801999897, -7.771324026006999692E-11, 191.0000000000000000 ) ) ;
#2138=CARTESIAN_POINT ( 'NONE',  ( 6.472425350819999146, 11.83301930295000126, 318.8802828394900644 ) ) ;
#2139=CARTESIAN_POINT ( 'NONE',  ( 0.000000000000000000, 0.000000000000000000, -315.0000000000000000 ) ) ;
#2140=VECTOR ( 'NONE', #5990, 1000.000000000000000 ) ;
#2143=EDGE_CURVE ( 'NONE', #4786, #9383, #9882, .T. ) ;
#2147=CARTESIAN_POINT ( 'NONE',  ( -2.814980436929585108E-10, -12.50000000000000000, 191.0000000000000000 ) ) ;
#2149=CARTESIAN_POINT ( 'NONE',  ( -14.65054575295525296, -4.807282645526338882, -315.0000000000000000 ) ) ;
#2150=CARTESIAN_POINT ( 'NONE',  ( -20.00000000000000000, -7.771159141713679452E-11, 191.0000000000000000 ) ) ;
#2152=CARTESIAN_POINT ( 'NONE',  ( 2.157987297531679616, 9.422522223986293355, -314.9999999999999432 ) ) ;
#2154=CARTESIAN_POINT ( 'NONE',  ( 19.55151251130001100, 0.8490756357253000930, 189.9229057364800042 ) ) ;
#2155=CARTESIAN_POINT ( 'NONE',  ( 15.42236153691470690, 4.758481100888916515, 314.4999482133868582 ) ) ;
#2156=ORIENTED_EDGE ( 'NONE', *, *, #7840, .T. ) ;
#2157=CARTESIAN_POINT ( 'NONE',  ( -6.294344443169999970, -10.85463315985999877, -317.5000000000000000 ) ) ;
#2160=CARTESIAN_POINT ( 'NONE',  ( 16.84526280568076118, -1.268064982489031545, 315.0000000000000568 ) ) ;
#2161=CARTESIAN_POINT ( 'NONE',  ( -8.759386130138000937, 8.782224002452998946, -314.4150829855000211 ) ) ;
#2163=CARTESIAN_POINT ( 'NONE',  ( -14.51666864684999680, 8.103202762918000346, 320.0770942683900557 ) ) ;
#2167=CARTESIAN_POINT ( 'NONE',  ( 13.67588481992999228, 8.646726704586995993, -317.5770954168139610 ) ) ;
#2168=CARTESIAN_POINT ( 'NONE',  ( -6.484736462137004942, -11.91614536315999828, -317.0792622552969533 ) ) ;
#2170=CARTESIAN_POINT ( 'NONE',  ( -17.50000000000125056, 0.2304358844820636465, -314.4997350343305129 ) ) ;
#2171=ORIENTED_EDGE ( 'NONE', *, *, #4040, .F. ) ;
#2172=CARTESIAN_POINT ( 'NONE',  ( -8.751711036432999080, 10.20177972100999853, 190.0000000000000000 ) ) ;
#2175=ORIENTED_EDGE ( 'NONE', *, *, #7655, .T. ) ;
#2176=CARTESIAN_POINT ( 'NONE',  ( 16.85039254115126539, 6.759165854037039622, -316.5000000000004547 ) ) ;
#2178=CARTESIAN_POINT ( 'NONE',  ( 17.49999999911141302, -5.867334123717704131, -302.4999999999996021 ) ) ;
#2179=CARTESIAN_POINT ( 'NONE',  ( -5.185096592093999313, -11.65847420015999170, -302.4229045757450081 ) ) ;
#2180=CARTESIAN_POINT ( 'NONE',  ( 13.93226991011998450, 8.970845217077998868, 191.1197171614399792 ) ) ;
#2182=CARTESIAN_POINT ( 'NONE',  ( 15.21156667173000621, 6.719223644262998008, -302.5071922382879279 ) ) ;
#2184=CARTESIAN_POINT ( 'NONE',  ( -10.18759338605000409, -10.75836373329000217, 318.8802828394900644 ) ) ;
#2185=CARTESIAN_POINT ( 'NONE',  ( -1.266716818501000041, -9.650794245151999462, -314.8616023057000461 ) ) ;
#2186=CARTESIAN_POINT ( 'NONE',  ( 18.86954045039000150, 1.614942466016999978, -302.4999999999529905 ) ) ;
#2195=CARTESIAN_POINT ( 'NONE',  ( -16.80170962578117155, 1.436180489853609688, 315.0000000000000568 ) ) ;
#2196=CARTESIAN_POINT ( 'NONE',  ( -16.24851264371998738, -5.765366273007000331, 319.9928079742500131 ) ) ;
#2197=CARTESIAN_POINT ( 'NONE',  ( -6.369817261971415512, -8.818538635844451079, -315.0000000000000000 ) ) ;
#2198=CARTESIAN_POINT ( 'NONE',  ( -17.50000000088855501, -5.867334121986932161, 189.9999999999998010 ) ) ;
#2201=FACE_OUTER_BOUND ( 'NONE', #9913, .T. ) ;
#2203=CARTESIAN_POINT ( 'NONE',  ( 1.962614641415807215, 9.435987819058210491, -314.9999999999999432 ) ) ;
#2204=CARTESIAN_POINT ( 'NONE',  ( -19.59090808375999515, 0.09664295149309998223, 189.9229057364800042 ) ) ;
#2205=CARTESIAN_POINT ( 'NONE',  ( 1.514429654104534930E-09, 10.00000000000000000, -302.5000000000000568 ) ) ;
#2207=CARTESIAN_POINT ( 'NONE',  ( -8.891587890486999157, -10.15986303230000054, -317.5000000000000000 ) ) ;
#2211=CARTESIAN_POINT ( 'NONE',  ( 16.74588786138889063, -1.629246332199927538, 315.0000000000000000 ) ) ;
#2212=CARTESIAN_POINT ( 'NONE',  ( 1.266716818501000041, 9.650794245151999462, -314.8616023057000461 ) ) ;
#2216=CARTESIAN_POINT ( 'NONE',  ( 14.64020885817999584, 8.017619026918998415, 320.0770942683900557 ) ) ;
#2220=CARTESIAN_POINT ( 'NONE',  ( 18.86307259346999032, -0.4762574081846996932, -317.4928077629770087 ) ) ;
#2221=CARTESIAN_POINT ( 'NONE',  ( 10.59417419979999586, -10.60664446758999446, -316.3802825947000201 ) ) ;
#2224=CARTESIAN_POINT ( 'NONE',  ( -16.39269942312257200, 3.424609558409217325, -314.5540176726823347 ) ) ;
#2230=CARTESIAN_POINT ( 'NONE',  ( 11.66810544104021297, 10.16551412172561442, -316.5000000000004547 ) ) ;
#2232=CARTESIAN_POINT ( 'NONE',  ( -12.11102551177084941, -6.646503028198875285, 314.9999999999999432 ) ) ;
#2233=CARTESIAN_POINT ( 'NONE',  ( -16.55370135034999990, -6.459991253353003948, -302.4229045757450081 ) ) ;
#2236=CARTESIAN_POINT ( 'NONE',  ( 15.65461689722998706, 7.260828390490999595, -302.4229045757450081 ) ) ;
#2237=CARTESIAN_POINT ( 'NONE',  ( -19.00000000000000000, 0.000000000000000000, -302.5000000001010108 ) ) ;
#2239=CARTESIAN_POINT ( 'NONE',  ( 8.759386130138000937, -8.782224002452998946, -314.4150829855000211 ) ) ;
#2240=CARTESIAN_POINT ( 'NONE',  ( -17.50000000000000711, 8.653878165429867666E-10, 190.0000000000001137 ) ) ;
#2242=CARTESIAN_POINT ( 'NONE',  ( 19.10187173594998811, -2.686732971880998910, 189.9229057364800042 ) ) ;
#2248=CARTESIAN_POINT ( 'NONE',  ( -14.23799507159000122, -5.083276007328000112, 315.0848619657999734 ) ) ;
#2251=CARTESIAN_POINT ( 'NONE',  ( -3.309734165293447550, -9.320883339027414394, -315.0000000000000568 ) ) ;
#2252=CARTESIAN_POINT ( 'NONE',  ( -10.23467949917771591, -9.999999999493891067, 189.9999999999997726 ) ) ;
#2257=CARTESIAN_POINT ( 'NONE',  ( -15.66663193639001506, 7.880331994043005217, 190.4207385301700128 ) ) ;
#2263=CARTESIAN_POINT ( 'NONE',  ( 0.000000000000000000, 10.54711710274999881, -315.0000000000000000 ) ) ;
#2265=CARTESIAN_POINT ( 'NONE',  ( 16.07469914181999826, 3.754035329064000059, -314.6383426456000052 ) ) ;
#2268=CARTESIAN_POINT ( 'NONE',  ( -18.44593188493998426, 2.441603908132000011, 319.9928079742500131 ) ) ;
#2272=CARTESIAN_POINT ( 'NONE',  ( -18.63147570264002084, 4.749337304460001796, -317.0792622552969533 ) ) ;
#2273=CARTESIAN_POINT ( 'NONE',  ( 13.93264803488000858, -8.974986968055002734, -316.3802825947000201 ) ) ;
#2275=CARTESIAN_POINT ( 'NONE',  ( 2.579601697407999605, -11.41110358643000033, 320.0000000000000000 ) ) ;
#2279=DIRECTION ( 'NONE',  ( -2.716996281154024841E-06, 0.9999999999963090636, 1.474966429758616062E-22 ) ) ;
#2282=CARTESIAN_POINT ( 'NONE',  ( -11.52006393673609885, -7.476351274249519285, -314.5677505184611391 ) ) ;
#2283=ORIENTED_EDGE ( 'NONE', *, *, #1436, .F. ) ;
#2286=CARTESIAN_POINT ( 'NONE',  ( -14.44906369208900365, -4.983045831585199537, 315.0000000000000568 ) ) ;
#2287=CARTESIAN_POINT ( 'NONE',  ( 19.46926817186999514, -1.611439533454998241, -302.4229045757450081 ) ) ;
#2289=ORIENTED_EDGE ( 'NONE', *, *, #9983, .F. ) ;
#2290=CARTESIAN_POINT ( 'NONE',  ( 1.988818824435997890, 12.53224469152999099, -302.9207377450070453 ) ) ;
#2292=CARTESIAN_POINT ( 'NONE',  ( -13.15302580975001234, -9.418553998452996012, 318.8802828394900644 ) ) ;
#2294=CARTESIAN_POINT ( 'NONE',  ( -6.322301096779000318, -8.991223814764000011, -314.8616023057000461 ) ) ;
#2297=CARTESIAN_POINT ( 'NONE',  ( -16.23266328071998643, -5.782092517776998619, 190.0071920248299477 ) ) ;
#2298=CARTESIAN_POINT ( 'NONE',  ( -19.49681644515301215, 2.834072041603171499, 190.9999999999996589 ) ) ;
#2301=CARTESIAN_POINT ( 'NONE',  ( -8.655660348039997842, -8.816209662726999241, 314.4150829855000211 ) ) ;
#2306=CARTESIAN_POINT ( 'NONE',  ( 3.205490369836122788, 12.35619803902316960, 319.0000000000005116 ) ) ;
#2308=CARTESIAN_POINT ( 'NONE',  ( -15.00000000000000000, 0.000000000000000000, 315.0000000000000000 ) ) ;
#2313=CARTESIAN_POINT ( 'NONE',  ( 6.027267673561996553, 11.50416862954998365, 189.9229057364800042 ) ) ;
#2314=CARTESIAN_POINT ( 'NONE',  ( -10.23467949614885697, 10.00000000050611781, 189.9999999999995737 ) ) ;
#2320=CARTESIAN_POINT ( 'NONE',  ( -5.255569329967309855, -12.07344867603089256, -303.5000000000006253 ) ) ;
#2321=CARTESIAN_POINT ( 'NONE',  ( 16.54291557298000370, 1.991497705781999805, -315.0848619657999734 ) ) ;
#2323=CARTESIAN_POINT ( 'NONE',  ( 19.55138120870000407, 0.8505817651195003437, 320.0770942683900557 ) ) ;
#2328=CARTESIAN_POINT ( 'NONE',  ( 19.56018598331999314, -0.5259244641825996380, -317.5770954168139610 ) ) ;
#2332=DIRECTION ( 'NONE',  ( 0.000000000000000000, 0.000000000000000000, 1.000000000000000000 ) ) ;
#2334=CARTESIAN_POINT ( 'NONE',  ( 0.000000000000000000, 0.000000000000000000, 190.0000000000000000 ) ) ;
#2341=CARTESIAN_POINT ( 'NONE',  ( -4.669690493011572130, -9.131031402067035785, 315.0000000000001137 ) ) ;
#2342=CARTESIAN_POINT ( 'NONE',  ( -0.1642067852079997503, -12.59486910148998895, -302.9207377450070453 ) ) ;
#2343=EDGE_CURVE ( 'NONE', #3286, #7297, #651, .T. ) ;
#2347=CARTESIAN_POINT ( 'NONE',  ( 11.28781796570999951, -4.951468039558000633, 315.0000000000000000 ) ) ;
#2349=CARTESIAN_POINT ( 'NONE',  ( -11.75341581114999023, 10.21170493764999598, -302.9207377450070453 ) ) ;
#2352=CARTESIAN_POINT ( 'NONE',  ( -14.38384290288000145, -5.252906928686999599, -314.8616023057000461 ) ) ;
#2356=CARTESIAN_POINT ( 'NONE',  ( 9.985646804708002477, -10.39189181891999780, 189.9229057364800042 ) ) ;
#2357=CARTESIAN_POINT ( 'NONE',  ( -17.62182611535274290, 5.928443937941890063, 190.9999999999996589 ) ) ;
#2359=CARTESIAN_POINT ( 'NONE',  ( 1.409290114754000012, -9.868237606049000021, 314.6383426456000052 ) ) ;
#2360=CARTESIAN_POINT ( 'NONE',  ( 10.32803372116435270, 10.00000000000000178, 315.0000000000000000 ) ) ;
#2362=CARTESIAN_POINT ( 'NONE',  ( -16.80239380511999059, -5.162410948549997158, 319.9928079742500131 ) ) ;
#2366=ORIENTED_EDGE ( 'NONE', *, *, #8488, .T. ) ;
#2369=CARTESIAN_POINT ( 'NONE',  ( 4.407678726681998782, 11.78447947993998390, 189.9229057364800042 ) ) ;
#2371=AXIS2_PLACEMENT_3D ( 'NONE', #9691, #5542, #3132 ) ;
#2375=CARTESIAN_POINT ( 'NONE',  ( 19.99979308783253273, -0.5741528085765136291, -303.4999999999998295 ) ) ;
#2379=CARTESIAN_POINT ( 'NONE',  ( 16.43550475785002263, 7.239471399781003846, 319.5792614743400009 ) ) ;
#2381=EDGE_LOOP ( 'NONE', ( #7557, #8525, #10280, #4646, #1829 ) ) ;
#2382=CARTESIAN_POINT ( 'NONE',  ( 19.29920617650999404, 3.385971943253997640, -316.3802825947000201 ) ) ;
#2384=FACE_BOUND ( 'NONE', #9863, .T. ) ;
#2387=PRODUCT_DEFINITION ( 'UNKNOWN', '', #3704, #870 ) ;
#2388=CARTESIAN_POINT ( 'NONE',  ( -15.84610571802258150, 4.157530358492048883, -314.5664817403811639 ) ) ;
#2390=CARTESIAN_POINT ( 'NONE',  ( 7.495586483745385387, -11.60098025501653751, 319.0000000000003979 ) ) ;
#2391=ORIENTED_EDGE ( 'NONE', *, *, #4577, .F. ) ;
#2392=CARTESIAN_POINT ( 'NONE',  ( 19.86381236214655033, 1.775476277371076828, -316.5000000000004547 ) ) ;
#2394=CARTESIAN_POINT ( 'NONE',  ( -14.02825138570089081, -5.340904894142199488, 315.0000000000000568 ) ) ;
#2395=CARTESIAN_POINT ( 'NONE',  ( -1.957937398543000418, -12.03510449230999768, -302.4229045757450081 ) ) ;
#2398=EDGE_CURVE ( 'NONE', #4571, #10392, #1848, .T. ) ;
#2399=CARTESIAN_POINT ( 'NONE',  ( -16.59121592455001348, 6.423372090527998068, -302.4229045757450081 ) ) ;
#2400=CARTESIAN_POINT ( 'NONE',  ( 10.97158218462999457, -10.45285060525999121, 318.8802828394900644 ) ) ;
#2402=CARTESIAN_POINT ( 'NONE',  ( 4.031301020048999817, -9.630010295875997883, -314.6383426456000052 ) ) ;
#2403=CARTESIAN_POINT ( 'NONE',  ( 19.00000000000000000, 0.000000000000000000, -302.5000000001010108 ) ) ;
#2405=CARTESIAN_POINT ( 'NONE',  ( 18.32859070493001852, -4.258570244206002720, 189.9229057364800042 ) ) ;
#2406=CARTESIAN_POINT ( 'NONE',  ( 19.99999721801999897, 7.771189452710000131E-11, 191.0000000000000000 ) ) ;
#2407=CARTESIAN_POINT ( 'NONE',  ( -12.45686666771074513, 6.446195019498007994, -315.0000000000000568 ) ) ;
#2411=CARTESIAN_POINT ( 'NONE',  ( -8.587332113755000051, -8.603326289371000968, 314.6383426456000052 ) ) ;
#2414=CARTESIAN_POINT ( 'NONE',  ( -13.36276382026999876, 8.154196903800000840, 320.0000000000000000 ) ) ;
#2416=DIRECTION ( 'NONE',  ( -1.000000000000000000, 0.000000000000000000, 0.000000000000000000 ) ) ;
#2417=CARTESIAN_POINT ( 'NONE',  ( 17.50000000000001776, -8.653793959161173735E-10, -302.4999999999998863 ) ) ;
#2421=CARTESIAN_POINT ( 'NONE',  ( 15.00000000000000000, 0.4945770392355999800, -285.0000000000000000 ) ) ;
#2423=CARTESIAN_POINT ( 'NONE',  ( 20.00000000435078107, -7.322330466941333604, -303.4999999999999432 ) ) ;
#2424=CARTESIAN_POINT ( 'NONE',  ( 15.45559681510979466, 3.931366100772827998, 315.0000000000000000 ) ) ;
#2426=CARTESIAN_POINT ( 'NONE',  ( 19.99999035944999903, -7.277437094418000096E-10, -303.5000000000000000 ) ) ;
#2427=CARTESIAN_POINT ( 'NONE',  ( -12.33444409538000031, -8.732262621622000509, -302.5000000000000000 ) ) ;
#2430=CARTESIAN_POINT ( 'NONE',  ( -17.04863675780999088, 6.660280422001000566, 319.5792614743400009 ) ) ;
#2434=CARTESIAN_POINT ( 'NONE',  ( 19.98383894087000812, -0.4026063077914996402, -316.3802825947000201 ) ) ;
#2437=CARTESIAN_POINT ( 'NONE',  ( -12.63876572971000023, -8.567575428377999458, 320.0000000000000000 ) ) ;
#2441=CARTESIAN_POINT ( 'NONE',  ( 14.89798725392377143, -4.565017050278198596, -314.9999999999999432 ) ) ;
#2443=CARTESIAN_POINT ( 'NONE',  ( 16.39269942312257911, -3.424609558409206223, -314.5540176726823347 ) ) ;
#2452=CARTESIAN_POINT ( 'NONE',  ( 10.38823308980000704, 10.24279834975000192, -302.4229045757450081 ) ) ;
#2454=ORIENTED_EDGE ( 'NONE', *, *, #2095, .T. ) ;
#2455=CARTESIAN_POINT ( 'NONE',  ( -16.77099092997999819, -1.279831385791999843, -315.0848619657999734 ) ) ;
#2456=CARTESIAN_POINT ( 'NONE',  ( -14.35075321877000043, 7.519064610420000072, -302.5000000000000000 ) ) ;
#2458=EDGE_LOOP ( 'NONE', ( #2524, #2156, #10620, #10470 ) ) ;
#2459=CARTESIAN_POINT ( 'NONE',  ( -18.35205128653998230, -4.220047386950002810, 189.9229057364800042 ) ) ;
#2461=CARTESIAN_POINT ( 'NONE',  ( 14.25125116527599545, 5.161338287358923971, -315.0000000000000568 ) ) ;
#2462=CARTESIAN_POINT ( 'NONE',  ( -10.00000000000000000, 2.500000000000000000, -285.0000000000000000 ) ) ;
#2465=CARTESIAN_POINT ( 'NONE',  ( 6.537559671572000575, -9.400791339334000796, 314.4150829855000211 ) ) ;
#2467=CARTESIAN_POINT ( 'NONE',  ( -14.64020885817999584, -8.017619026918998415, 320.0770942683900557 ) ) ;
#2469=CARTESIAN_POINT ( 'NONE',  ( 13.88908508137762432, 9.009716997455479159, -303.5000000000000000 ) ) ;
#2473=VERTEX_POINT ( 'NONE', #4891 ) ;
#2476=DIRECTION ( 'NONE',  ( 2.558226600336915673E-07, -0.9999999999999674705, 3.955942811920841838E-22 ) ) ;
#2477=CARTESIAN_POINT ( 'NONE',  ( -17.50000000000000000, 0.000000000000000000, -314.4999343908002061 ) ) ;
#2480=CARTESIAN_POINT ( 'NONE',  ( 16.77099092997999819, 1.279831385791999843, -315.0848619657999734 ) ) ;
#2483=CARTESIAN_POINT ( 'NONE',  ( -17.34597251029000375, 4.674348096672999553, 190.0000000000000000 ) ) ;
#2485=FACE_OUTER_BOUND ( 'NONE', #5432, .T. ) ;
#2487=CARTESIAN_POINT ( 'NONE',  ( 20.10111883311001080, 0.3733660053931999734, -317.0792622552969533 ) ) ;
#2492=CARTESIAN_POINT ( 'NONE',  ( 8.531707904373998730, -10.27069628977000093, 320.0000000000000000 ) ) ;
#2496=CARTESIAN_POINT ( 'NONE',  ( 3.024115758602054171, -9.348088905657229830, -315.0000000000000568 ) ) ;
#2498=CARTESIAN_POINT ( 'NONE',  ( 17.19853431800999743, 2.231396706187000145, -315.0000000000001137 ) ) ;
#2500=CARTESIAN_POINT ( 'NONE',  ( 17.62191473184000046, 4.312542294520999242, -317.5000000000030127 ) ) ;
#2502=CARTESIAN_POINT ( 'NONE',  ( 11.75341581114999023, -10.21170493764999598, -302.9207377450070453 ) ) ;
#2503=CARTESIAN_POINT ( 'NONE',  ( 18.90091799877999179, -0.2928069713013998765, -317.4928077629770087 ) ) ;
#2507=CARTESIAN_POINT ( 'NONE',  ( 10.53744240725999681, 10.62869657088999986, -303.6197174156520759 ) ) ;
#2508=CARTESIAN_POINT ( 'NONE',  ( -10.25126261553517537, 10.00000004282989785, 314.9999999999999432 ) ) ;
#2509=VERTEX_POINT ( 'NONE', #10584 ) ;
#2510=CARTESIAN_POINT ( 'NONE',  ( -17.56330558013000243, -0.6698376231023999150, -314.4150829855000211 ) ) ;
#2513=CARTESIAN_POINT ( 'NONE',  ( -18.77789454208001985, -4.479159834667000517, 190.4207385301700128 ) ) ;
#2514=FACE_OUTER_BOUND ( 'NONE', #4926, .T. ) ;
#2515=CARTESIAN_POINT ( 'NONE',  ( 16.99996037728000076, -1.352915083302999933E-09, -314.9999801883000146 ) ) ;
#2518=CARTESIAN_POINT ( 'NONE',  ( 17.18263598829999950, -2.199757124398999952, 314.4150829855000211 ) ) ;
#2520=CARTESIAN_POINT ( 'NONE',  ( 18.44593188493998426, -2.441603908132000011, 319.9928079742500131 ) ) ;
#2521=CARTESIAN_POINT ( 'NONE',  ( -16.99398431597748171, 6.605820200493087491, 319.0000000000005116 ) ) ;
#2523=CARTESIAN_POINT ( 'NONE',  ( 17.11849373668000140, 0.6181952683021000317, 314.8616023057000461 ) ) ;
#2524=ORIENTED_EDGE ( 'NONE', *, *, #3365, .T. ) ;
#2525=CARTESIAN_POINT ( 'NONE',  ( 1.249193831065165128, -12.49557363514548314, 190.9999999999995737 ) ) ;
#2529=CARTESIAN_POINT ( 'NONE',  ( 14.21175436428723771, 5.188485551603381651, 315.0000000000000000 ) ) ;
#2530=CARTESIAN_POINT ( 'NONE',  ( -15.00000000000000000, -0.4945770392355999800, -285.0000000000000000 ) ) ;
#2531=ORIENTED_EDGE ( 'NONE', *, *, #4895, .T. ) ;
#2533=ADVANCED_FACE ( 'NONE', ( #653 ), #3598, .T. ) ;
#2535=CARTESIAN_POINT ( 'NONE',  ( 16.84157450053000105, 5.300668178571999789, 190.0000000000000000 ) ) ;
#2540=CARTESIAN_POINT ( 'NONE',  ( 11.69962851017000283, 10.23591410519999201, -317.0792622552969533 ) ) ;
#2546=CARTESIAN_POINT ( 'NONE',  ( -1.962614641415807659, -9.435987819058212267, -315.0000000000000000 ) ) ;
#2548=CARTESIAN_POINT ( 'NONE',  ( 13.85286411329786560, -6.044949306166734537, -314.5816605312646175 ) ) ;
#2552=CARTESIAN_POINT ( 'NONE',  ( 20.06707331603001521, 0.4205479510244998220, -302.9207377450070453 ) ) ;
#2553=CARTESIAN_POINT ( 'NONE',  ( -4.800908653447998553, -11.01413625319999845, -317.4928077629770087 ) ) ;
#2554=CARTESIAN_POINT ( 'NONE',  ( -19.99999035944999903, 7.277427703818000446E-10, -303.5000000000000000 ) ) ;
#2557=CARTESIAN_POINT ( 'NONE',  ( -16.56522182708686941, -3.263825229738949840, 314.4999489731223434 ) ) ;
#2560=CARTESIAN_POINT ( 'NONE',  ( -3.370560865743999823, 11.33032003377000052, -302.5000000000000000 ) ) ;
#2562=CARTESIAN_POINT ( 'NONE',  ( -2.655864369898997435, -12.48600887025999029, 190.4207385301700128 ) ) ;
#2566=CARTESIAN_POINT ( 'NONE',  ( -13.10162021654998732, 9.446493979990000511, 191.1197171614399792 ) ) ;
#2569=CARTESIAN_POINT ( 'NONE',  ( 15.43693218238999876, -4.538485726840999490, 314.6383426456000052 ) ) ;
#2571=CARTESIAN_POINT ( 'NONE',  ( -19.11656497511998154, -2.646905232783001605, 320.0770942683900557 ) ) ;
#2574=CARTESIAN_POINT ( 'NONE',  ( 6.419414596134000561, 9.427679607337001499, 314.4150829855000211 ) ) ;
#2577=CARTESIAN_POINT ( 'NONE',  ( -7.561138155138405814, -11.58431960382585402, 190.9999999999995737 ) ) ;
#2584=CARTESIAN_POINT ( 'NONE',  ( 3.689342025446077589, 9.275861061134104801, 315.0000000000001137 ) ) ;
#2591=CARTESIAN_POINT ( 'NONE',  ( 14.94331899262999919, 7.078020551493000134, 190.0000000000000000 ) ) ;
#2592=CARTESIAN_POINT ( 'NONE',  ( 9.994973107563785319, -8.217268576751703080, 314.4999428952268659 ) ) ;
#2593=CARTESIAN_POINT ( 'NONE',  ( -13.57573464316000056, 3.225916527208000151, -284.9999999999999432 ) ) ;
#2595=CARTESIAN_POINT ( 'NONE',  ( 12.84330733966000437, 9.683159015349998455, -317.0792622552969533 ) ) ;
#2602=CARTESIAN_POINT ( 'NONE',  ( 11.93419529315104732, -6.745200168737855329, -315.0000000000000568 ) ) ;
#2604=CARTESIAN_POINT ( 'NONE',  ( -17.50000000000126832, 0.7437989020612977287, -314.4963898845654171 ) ) ;
#2608=CARTESIAN_POINT ( 'NONE',  ( -3.692777996438003196, -12.29248881612998190, -303.6197174156509391 ) ) ;
#2609=CARTESIAN_POINT ( 'NONE',  ( -18.77313104639999253, -1.494918992088000831, -317.4928077629770087 ) ) ;
#2611=CARTESIAN_POINT ( 'NONE',  ( -16.21525914616999842, 2.693567875512000054, -315.0848619657999734 ) ) ;
#2613=CARTESIAN_POINT ( 'NONE',  ( -20.06707331603001521, -0.4205479510244998220, -302.9207377450070453 ) ) ;
#2616=CARTESIAN_POINT ( 'NONE',  ( -17.16710485141000220, -2.239552065056999997, -314.4150829855000211 ) ) ;
#2617=CARTESIAN_POINT ( 'NONE',  ( -18.86992372454000133, 1.611776198549999872, -302.4999999999529905 ) ) ;
#2620=CARTESIAN_POINT ( 'NONE',  ( 19.56918397773000962, -2.861069655901001152, 190.4207385301700128 ) ) ;
#2621=CARTESIAN_POINT ( 'NONE',  ( 12.98706127646999953, -6.788989183774999603, -315.0000000000001137 ) ) ;
#2622=CARTESIAN_POINT ( 'NONE',  ( 13.82248977823974734, 5.505663031471445201, -315.0000000000000000 ) ) ;
#2624=CARTESIAN_POINT ( 'NONE',  ( 0.7125182177438000863, 12.50545814267000644, 191.1197171614399792 ) ) ;
#2625=CARTESIAN_POINT ( 'NONE',  ( 10.40890489166000066, -7.434429060800999522, 315.0848619657999734 ) ) ;
#2629=CARTESIAN_POINT ( 'NONE',  ( 0.6255878334489998194, -12.09339422449000168, 320.0770942683900557 ) ) ;
#2630=CARTESIAN_POINT ( 'NONE',  ( -17.44869542604064705, 0.8969788624277408307, 314.4999390965243720 ) ) ;
#2631=CARTESIAN_POINT ( 'NONE',  ( 19.86375996897344720, 1.775925728142829341, -303.4999999999999432 ) ) ;
#2632=CARTESIAN_POINT ( 'NONE',  ( 10.50000150490000017, 7.882579085736000302, 314.6383426456000052 ) ) ;
#2635=CARTESIAN_POINT ( 'NONE',  ( 13.15302580975001234, 9.418553998452996012, 318.8802828394900644 ) ) ;
#2638=CARTESIAN_POINT ( 'NONE',  ( -0.9841565935054803482, 9.488387273935385835, 314.9999999999999432 ) ) ;
#2640=CARTESIAN_POINT ( 'NONE',  ( -15.00000000000325784, 8.632726818195413123E-17, -284.9999999999999432 ) ) ;
#2645=CARTESIAN_POINT ( 'NONE',  ( -1.290325097615000027, 11.49300988401000012, 190.0000000000000000 ) ) ;
#2647=CARTESIAN_POINT ( 'NONE',  ( 15.00000000000325784, -8.632726818195413123E-17, -284.9999999999999432 ) ) ;
#2653=CARTESIAN_POINT ( 'NONE',  ( 17.19853431800999743, 2.231396706187000145, -315.0000000000000000 ) ) ;
#2655=CARTESIAN_POINT ( 'NONE',  ( 9.619051408962835836, -7.822710805390641120, -315.0000000000000568 ) ) ;
#2658=CARTESIAN_POINT ( 'NONE',  ( -19.99984272814741715, -0.5882336804855470280, -316.5000000000004547 ) ) ;
#2663=CARTESIAN_POINT ( 'NONE',  ( 1.546121016139999638, 11.35842264293001591, -317.4928077629770087 ) ) ;
#2665=CARTESIAN_POINT ( 'NONE',  ( -16.86005112630999037, -5.110605191077000065, -317.4928077629770087 ) ) ;
#2670=CARTESIAN_POINT ( 'NONE',  ( 19.98381222165001248, -0.4032365313531999784, -303.6197174156509391 ) ) ;
#2673=EDGE_CURVE ( 'NONE', #9383, #563, #6489, .T. ) ;
#2674=CARTESIAN_POINT ( 'NONE',  ( -10.14429053679999981, 9.716529139337000132, -302.5000000000000000 ) ) ;
#2676=CARTESIAN_POINT ( 'NONE',  ( 16.34052447997000357, -7.211013068275999416, 191.1197171614399792 ) ) ;
#2677=CARTESIAN_POINT ( 'NONE',  ( -15.67978886374999803, -4.575336738469999887, -314.4944826805095772 ) ) ;
#2678=CARTESIAN_POINT ( 'NONE',  ( 15.43598538069025139, 3.955158390306824590, -315.0000000000000568 ) ) ;
#2680=CARTESIAN_POINT ( 'NONE',  ( -19.95847042008000827, 0.9399586737018998939, 191.1197171614399792 ) ) ;
#2681=CARTESIAN_POINT ( 'NONE',  ( 12.07130791616000032, -6.858215270785999351, 314.8616023057000461 ) ) ;
#2685=CARTESIAN_POINT ( 'NONE',  ( 18.12318599310000167, -3.186119256560000945, 319.9928079742500131 ) ) ;
#2687=CARTESIAN_POINT ( 'NONE',  ( 1.984036549750167300, 12.45525792938212639, -303.4999999999990905 ) ) ;
#2688=CARTESIAN_POINT ( 'NONE',  ( 12.21495827233999876, 7.290170534263999969, 314.4150829855000211 ) ) ;
#2690=CARTESIAN_POINT ( 'NONE',  ( 17.01113700077726776, -6.587853872568209646, 190.9999999999995737 ) ) ;
#2691=CARTESIAN_POINT ( 'NONE',  ( 9.099181536070998888, 11.22222323403999766, 319.5792614743400009 ) ) ;
#2692=CARTESIAN_POINT ( 'NONE',  ( 18.99999441908000009, 1.671652446847999990E-07, 319.0000000000000000 ) ) ;
#2693=CARTESIAN_POINT ( 'NONE',  ( 4.780298404687055580, 9.113031460416761931, 315.0000000000000000 ) ) ;
#2700=CARTESIAN_POINT ( 'NONE',  ( -15.24002748250033967, 4.193218933356376965, -315.0000000000000000 ) ) ;
#2708=AXIS2_PLACEMENT_3D ( 'NONE', #8060, #2476, #9030 ) ;
#2710=CARTESIAN_POINT ( 'NONE',  ( 16.88284456999480554, -6.727435487264400216, -316.5000000000004547 ) ) ;
#2711=ORIENTED_EDGE ( 'NONE', *, *, #6008, .F. ) ;
#2715=CARTESIAN_POINT ( 'NONE',  ( -18.78102408959999536, 1.459157757289999413, -317.4928077629770087 ) ) ;
#2716=CARTESIAN_POINT ( 'NONE',  ( -18.28030995243001655, -2.924502517761999876, -317.4928077629770087 ) ) ;
#2718=CARTESIAN_POINT ( 'NONE',  ( -10.51805095810000346, 10.63699911018001210, -303.6197174156520759 ) ) ;
#2719=PLANE ( 'NONE',  #9604 ) ;
#2720=VERTEX_POINT ( 'NONE', #1329 ) ;
#2721=CARTESIAN_POINT ( 'NONE',  ( 19.00000000000000000, 0.000000000000000000, 190.0000000000100044 ) ) ;
#2727=CARTESIAN_POINT ( 'NONE',  ( 18.78105930652002087, -1.458809753444000767, -302.5071922382879279 ) ) ;
#2728=CARTESIAN_POINT ( 'NONE',  ( 11.06049270995999123, 10.50744457173999713, 190.4207385301700128 ) ) ;
#2733=CARTESIAN_POINT ( 'NONE',  ( -10.21681110195000031, -10.83745499882999574, 319.5792614743400009 ) ) ;
#2734=CARTESIAN_POINT ( 'NONE',  ( -17.05540562798465842, 2.295823712133366445, 314.4999398562647457 ) ) ;
#2735=CARTESIAN_POINT ( 'NONE',  ( -17.49999998521812117, 5.867334131620513205, 189.9999999999998010 ) ) ;
#2736=CARTESIAN_POINT ( 'NONE',  ( 17.36972170382999892, 0.04551883977364000466, 314.6383426456000052 ) ) ;
#2738=CARTESIAN_POINT ( 'NONE',  ( 11.17208682466014302, -10.37722895585535454, 190.9999999999995737 ) ) ;
#2739=CARTESIAN_POINT ( 'NONE',  ( -8.796035389134001292, 11.31703133948999707, 319.5792614743400009 ) ) ;
#2743=CARTESIAN_POINT ( 'NONE',  ( -5.334308159457383347, 9.025045582129868293, 314.9999999999999432 ) ) ;
#2746=CARTESIAN_POINT ( 'NONE',  ( 15.28688047792000049, -6.812924772642000804, -302.5000000000000000 ) ) ;
#2748=CARTESIAN_POINT ( 'NONE',  ( 18.78940217795999956, 1.754852253524999961, 190.0000000000000000 ) ) ;
#2749=CARTESIAN_POINT ( 'NONE',  ( 5.453155204153861568, -9.512440879258083015, 314.4999437815906163 ) ) ;
#2750=CARTESIAN_POINT ( 'NONE',  ( 18.89053622393001675, 0.06335528492990002980, 190.0071920248299477 ) ) ;
#2756=CARTESIAN_POINT ( 'NONE',  ( 8.736690731312993563, 10.08117623986000133, 319.9928079742500131 ) ) ;
#2760=ORIENTED_EDGE ( 'NONE', *, *, #5354, .T. ) ;
#2763=DIRECTION ( 'NONE',  ( -3.267118270366935116E-06, -8.358028872200239840E-13, -0.9999999999946629359 ) ) ;
#2764=CARTESIAN_POINT ( 'NONE',  ( -19.56018598331999314, 0.5259244641825996380, -317.5770954168139610 ) ) ;
#2766=CARTESIAN_POINT ( 'NONE',  ( 16.63787452912263731, 3.035984518719835101, -314.5459997954137066 ) ) ;
#2773=CARTESIAN_POINT ( 'NONE',  ( 13.10162021654998732, -9.446493979990000511, 191.1197171614399792 ) ) ;
#2776=CARTESIAN_POINT ( 'NONE',  ( 0.000000000000000000, 10.00000000000000000, 315.0000000000000000 ) ) ;
#2777=CARTESIAN_POINT ( 'NONE',  ( -10.12800840543000724, 10.78031690431999756, 191.1197171614399792 ) ) ;
#2783=CARTESIAN_POINT ( 'NONE',  ( -20.06710154196001739, 0.4210530330733002757, 319.5792614743400009 ) ) ;
#2786=CARTESIAN_POINT ( 'NONE',  ( -14.72449281369000040, 5.549439731021000632, 314.4150829855000211 ) ) ;
#2788=CARTESIAN_POINT ( 'NONE',  ( -19.99996770037257221, -0.3054858693455834162, 190.9999999999995737 ) ) ;
#2790=CARTESIAN_POINT ( 'NONE',  ( -20.00506338957998409, 0.1012955751877999966, 318.8802828394900644 ) ) ;
#2796=CARTESIAN_POINT ( 'NONE',  ( 20.00000000000000000, 0.000000000000000000, 191.0000000000000000 ) ) ;
#2802=CARTESIAN_POINT ( 'NONE',  ( -1.205561540619000116, 11.37600766585000933, 190.0071920248299477 ) ) ;
#2804=B_SPLINE_SURFACE_WITH_KNOTS ( 'NONE', 3, 1, ( 
 ( #10604, #4106 ),
 ( #6743, #3296 ),
 ( #2498, #5812 ),
 ( #1849, #4913 ),
 ( #5010, #827 ),
 ( #4057, #4962 ),
 ( #8288, #928 ),
 ( #5764, #874 ),
 ( #3246, #6524 ),
 ( #7386, #9805 ),
 ( #1688, #3408 ),
 ( #9963, #2604 ),
 ( #5865, #6182 ) ),
 .UNSPECIFIED., .F., .F., .F.,
 ( 4, 1, 1, 1, 1, 1, 1, 1, 1, 1, 4 ),
 ( 2, 2 ),
 ( 0.01923076854978476163, 0.09935897435896999530, 0.1794871794871999993, 0.2596153846154000133, 0.3397435897436000274, 0.5000000000000000000, 0.6602564102564000281, 0.7403846153845999867, 0.8205128205128000562, 0.9006410256410000148, 0.9807692307692000844 ),
 ( 0.000000000000000000, 1.000000000000000000 ),
 .UNSPECIFIED. ) ;
#2807=CARTESIAN_POINT ( 'NONE',  ( 12.16656789651012005, -6.621481216618937182, 314.9999999999999432 ) ) ;
#2808=CARTESIAN_POINT ( 'NONE',  ( -12.17979804859000126, 7.053762231097000068, -314.6383426456000052 ) ) ;
#2811=CARTESIAN_POINT ( 'NONE',  ( -8.447271450478007537, 10.17170359172999738, 319.9928079742500131 ) ) ;
#2815=CARTESIAN_POINT ( 'NONE',  ( -18.87178158963000030, -0.3573130366704001526, -317.4928077629770087 ) ) ;
#2816=CARTESIAN_POINT ( 'NONE',  ( 12.90264537120001798, -9.651629027462002242, -317.0792622552969533 ) ) ;
#2817=AXIS2_PLACEMENT_3D ( 'NONE', #8634, #3966, #3161 ) ;
#2825=CARTESIAN_POINT ( 'NONE',  ( 15.66827725153000017, -6.479182156166999995, 190.0000000000000000 ) ) ;
#2829=ORIENTED_EDGE ( 'NONE', *, *, #4577, .T. ) ;
#2830=CARTESIAN_POINT ( 'NONE',  ( -13.01115177740000384, -9.495820311550003723, 191.1197171614399792 ) ) ;
#2832=CARTESIAN_POINT ( 'NONE',  ( -16.39045651208371979, -2.501479531468998818, 315.0000000000000000 ) ) ;
#2834=CARTESIAN_POINT ( 'NONE',  ( 19.14223954934999483, 3.638712114223002558, 191.1197171614399792 ) ) ;
#2839=CARTESIAN_POINT ( 'NONE',  ( -19.96334758606998605, -0.8982332345458986511, 318.8802828394900644 ) ) ;
#2840=CARTESIAN_POINT ( 'NONE',  ( 16.89986669904000394, -0.5583209492923999484, -315.0848619657999734 ) ) ;
#2841=CARTESIAN_POINT ( 'NONE',  ( -16.55686070535999832, 1.955716293870999767, 315.0848619657999734 ) ) ;
#2845=LINE ( 'NONE', #7139, #3275 ) ;
#2847=CARTESIAN_POINT ( 'NONE',  ( -16.83787941357387297, 1.297844089352232944, 315.0000000000000568 ) ) ;
#2848=CARTESIAN_POINT ( 'NONE',  ( 11.71572875238734213, -12.50000000010304113, 190.9999999999999432 ) ) ;
#2850=CARTESIAN_POINT ( 'NONE',  ( 19.79155829785256415, 1.881978406165077722, 319.0000000000005116 ) ) ;
#2854=CARTESIAN_POINT ( 'NONE',  ( -8.021995458420214220, 8.375882622524637000, -315.0000000000000568 ) ) ;
#2855=CARTESIAN_POINT ( 'NONE',  ( 2.556522775252001445, 11.29259618907000196, 190.0071920248299477 ) ) ;
#2857=CARTESIAN_POINT ( 'NONE',  ( 12.36094278317000139, -8.718445687105001340, -317.5000000000000000 ) ) ;
#2860=CARTESIAN_POINT ( 'NONE',  ( 11.74237836840727311, -6.849546447955716211, 315.0000000000000000 ) ) ;
#2861=CARTESIAN_POINT ( 'NONE',  ( -10.67587555525000020, 8.049811041411000900, -314.4150829855000211 ) ) ;
#2863=CARTESIAN_POINT ( 'NONE',  ( -17.33328289455318938, -2.867118240563160875E-08, 314.6666162271453118 ) ) ;
#2864=CARTESIAN_POINT ( 'NONE',  ( -3.357323174585255643, -12.33819210890098894, -316.5000000000004547 ) ) ;
#2867=CARTESIAN_POINT ( 'NONE',  ( -16.88563860788000781, 5.080169144092001154, -317.4928077629770087 ) ) ;
#2868=CARTESIAN_POINT ( 'NONE',  ( -20.10111883311001080, -0.3733660053931999734, -317.0792622552969533 ) ) ;
#2869=EDGE_CURVE ( 'NONE', #8301, #4592, #7779, .T. ) ;
#2870=B_SPLINE_CURVE_WITH_KNOTS ( 'NONE', 3,
 ( #6499, #1614, #4886, #8005, #3057, #1445, #8107, #8165, #591, #10521, #802, #6442, #2308 ),
 .UNSPECIFIED., .F., .F.,
 ( 4, 1, 1, 1, 1, 1, 1, 1, 1, 1, 4 ),
 ( 0.000000000000000000, 0.08333333333333001192, 0.1666666666667000196, 0.2500000000000000000, 0.3333333333333000081, 0.5000000000000000000, 0.6666666666667000474, 0.7500000000000000000, 0.8333333333333000637, 0.9166666666667000474, 1.000000000000000000 ),
 .UNSPECIFIED. ) ;
#2873=CARTESIAN_POINT ( 'NONE',  ( 3.650011388878862562, 9.782272988550909432, -314.5118284007356237 ) ) ;
#2875=CARTESIAN_POINT ( 'NONE',  ( 0.000000000000000000, 0.000000000000000000, -302.5000000000000000 ) ) ;
#2880=CARTESIAN_POINT ( 'NONE',  ( 1.615578127792000274, -11.35484692374000737, -302.5071922382879279 ) ) ;
#2883=ADVANCED_FACE ( 'NONE', ( #7680 ), #9329, .F. ) ;
#2885=CARTESIAN_POINT ( 'NONE',  ( 0.1580967862520001599, 11.39739484195000330, -302.5071922382879279 ) ) ;
#2886=CARTESIAN_POINT ( 'NONE',  ( 18.24388381812998361, -5.273776366776003144, 319.5792614743400009 ) ) ;
#2887=CARTESIAN_POINT ( 'NONE',  ( 16.10362618234000109, -3.713712614977999760, -314.6383426456000052 ) ) ;
#2888=CARTESIAN_POINT ( 'NONE',  ( -16.89986669904000394, 0.5583209492923999484, 315.0848619657999734 ) ) ;
#2890=CARTESIAN_POINT ( 'NONE',  ( -19.14871320452657244, -3.641870911972378444, 190.9999999999995737 ) ) ;
#2894=CARTESIAN_POINT ( 'NONE',  ( 2.381287040813000348E-07, -10.00000001404999850, 190.0000000000000000 ) ) ;
#2895=CARTESIAN_POINT ( 'NONE',  ( -16.99996037728000076, 1.352916227065999958E-09, 314.9999801883000146 ) ) ;
#2897=CARTESIAN_POINT ( 'NONE',  ( -7.006889269069000115, -6.844138725329000472, -284.9999999999999432 ) ) ;
#2898=CARTESIAN_POINT ( 'NONE',  ( -16.34919249956382714, -2.583378889817198765, -315.0000000000000568 ) ) ;
#2899=DIRECTION ( 'NONE',  ( 0.000000000000000000, 0.000000000000000000, 1.000000000000000000 ) ) ;
#2900=( BOUNDED_SURFACE ( )  B_SPLINE_SURFACE ( 3, 1, ( 
 ( #6169, #2150 ),
 ( #3753, #3706 ),
 ( #9455, #5414 ),
 ( #6991, #2796 ) ),
 .UNSPECIFIED., .F., .F., .T. ) 
 B_SPLINE_SURFACE_WITH_KNOTS ( ( 4, 4 ),
 ( 2, 2 ),
 ( 0.000000000000000000, 1.000000000000000000 ),
 ( 0.000000000000000000, 1.000000000000000000 ),
 .UNSPECIFIED. ) 
 GEOMETRIC_REPRESENTATION_ITEM ( )  RATIONAL_B_SPLINE_SURFACE ( (
 ( 1.000000000000000000, 1.000000000000000000),
 ( 0.3333333333312610280, 0.3333333333312610280),
 ( 0.3333333333312610280, 0.3333333333312610280),
 ( 1.000000000000000000, 1.000000000000000000) ) ) 
 REPRESENTATION_ITEM ( '' )  SURFACE ( )  );
#2903=CARTESIAN_POINT ( 'NONE',  ( -11.28358823633008079, 7.096269052248557863, -315.0000000000001137 ) ) ;
#2904=CARTESIAN_POINT ( 'NONE',  ( 18.14082875322000277, 3.150077164920001671, 190.0071920248299477 ) ) ;
#2907=CARTESIAN_POINT ( 'NONE',  ( 5.180828043054999554, -11.07085478567999992, -317.5000000000000000 ) ) ;
#2912=CARTESIAN_POINT ( 'NONE',  ( 16.31058353111865955, -2.657800654349994129, 315.0000000000000000 ) ) ;
#2913=CARTESIAN_POINT ( 'NONE',  ( -4.031301020048999817, 9.630010295875997883, -314.6383426456000052 ) ) ;
#2918=CARTESIAN_POINT ( 'NONE',  ( 18.77313104639999253, 1.494918992088000831, -317.4928077629770087 ) ) ;
#2920=CARTESIAN_POINT ( 'NONE',  ( -14.97796429264999141, -8.396158284077998246, -317.0792622552969533 ) ) ;
#2922=CARTESIAN_POINT ( 'NONE',  ( 17.50000000000000000, -0.7437989020623000380, -315.0000000000000000 ) ) ;
#2924=CARTESIAN_POINT ( 'NONE',  ( -3.644504295958682416, 9.783030308347003157, -314.5117835914683155 ) ) ;
#2926=CARTESIAN_POINT ( 'NONE',  ( -18.20814976352000158, -3.283820199526999772, 190.0000000000000000 ) ) ;
#2927=CARTESIAN_POINT ( 'NONE',  ( -19.51225877040621981, -2.792229942217316019, 319.0000000000003979 ) ) ;
#2929=CARTESIAN_POINT ( 'NONE',  ( 7.781240562249999826, -11.51887802030999985, 191.1197171614399792 ) ) ;
#2931=CARTESIAN_POINT ( 'NONE',  ( -16.04008061823806131, -3.141427272462999021, 315.0000000000000000 ) ) ;
#2934=CARTESIAN_POINT ( 'NONE',  ( 17.02428600387000301, 6.565037456673000982, 191.1197171614399792 ) ) ;
#2936=CARTESIAN_POINT ( 'NONE',  ( 19.57075148197997549, -0.3818783754278996523, -302.4229045757450081 ) ) ;
#2937=CARTESIAN_POINT ( 'NONE',  ( 20.05691607070997051, 0.5615793767616999999, 319.5792614743400009 ) ) ;
#2938=CARTESIAN_POINT ( 'NONE',  ( 14.28417481768999941, -5.042936695466000430, -315.0848619657999734 ) ) ;
#2939=CARTESIAN_POINT ( 'NONE',  ( -17.36938240862999905, 0.02134527931160000100, 314.6383426456000052 ) ) ;
#2941=CARTESIAN_POINT ( 'NONE',  ( -7.284698641071005731, -10.49877923466000063, 190.0071920248299477 ) ) ;
#2942=CARTESIAN_POINT ( 'NONE',  ( -0.6337574957234999307, 12.50712592802002021, 318.8802828394900644 ) ) ;
#2947=CARTESIAN_POINT ( 'NONE',  ( -13.89435758465052828, 5.448822883216570823, 315.0000000000000568 ) ) ;
#2948=CARTESIAN_POINT ( 'NONE',  ( -13.57573464316000056, -3.225916527208000151, 315.0000000000001705 ) ) ;
#2949=CARTESIAN_POINT ( 'NONE',  ( -14.25125116527600078, -5.161338287358921306, -315.0000000000000568 ) ) ;
#2953=CARTESIAN_POINT ( 'NONE',  ( -4.669917308725587191, 9.131001784561973977, -315.0000000000000000 ) ) ;
#2955=AXIS2_PLACEMENT_3D ( 'NONE', #4423, #1246, #8449 ) ;
#2956=CARTESIAN_POINT ( 'NONE',  ( 17.86997157320001151, 4.940892756443005851, 189.9229057364800042 ) ) ;
#2960=CARTESIAN_POINT ( 'NONE',  ( 17.62858316411999837, -4.302404616280000482, -317.5000000000030127 ) ) ;
#2963=CARTESIAN_POINT ( 'NONE',  ( 8.616673968646825443, -8.177724119443702477, 315.0000000000000000 ) ) ;
#2964=CARTESIAN_POINT ( 'NONE',  ( -1.419551022038999966, 10.09154694854999867, -314.4150829855000211 ) ) ;
#2965=DIRECTION ( 'NONE',  ( 0.000000000000000000, -1.000000000000000000, 0.000000000000000000 ) ) ;
#2967=CARTESIAN_POINT ( 'NONE',  ( 3.163121738623003054, 11.93735872977999968, 320.0770942683900557 ) ) ;
#2969=EDGE_LOOP ( 'NONE', ( #2366, #4306, #4136, #4911 ) ) ;
#2970=CARTESIAN_POINT ( 'NONE',  ( -7.982667963825995194, 11.03627960042998701, -317.5770954168139610 ) ) ;
#2971=CARTESIAN_POINT ( 'NONE',  ( 20.05670149355997722, 0.5623089763428997800, -317.0792622552969533 ) ) ;
#2975=CARTESIAN_POINT ( 'NONE',  ( 19.49702808861182746, -2.833672667318399618, 319.0000000000003979 ) ) ;
#2978=CARTESIAN_POINT ( 'NONE',  ( 12.80773887004084877, 9.614708322195337331, -316.5000000000004547 ) ) ;
#2979=ORIENTED_EDGE ( 'NONE', *, *, #10090, .T. ) ;
#2980=( BOUNDED_CURVE ( )  B_SPLINE_CURVE ( 3, ( #2119, #5187, #5237, #6195, #2927, #6966, #8512, #5285, #1255, #4533, #8460, #9332, #1154, #8558, #7712, #9481, #1204, #7758, #3947, #4757, #9534, #8137, #8888, #7280, #3784, #8026, #5606, #7071, #2390, #8941, #3140, #672, #7227, #10493, #1526, #4810, #562, #10339, #4645, #1478, #8081, #3196, #3029, #2975, #7978, #4862, #1585, #619 ),
 .UNSPECIFIED., .F., .F. ) 
 B_SPLINE_CURVE_WITH_KNOTS ( ( 4, 1, 1, 1, 1, 1, 1, 1, 1, 1, 1, 1, 1, 1, 1, 1, 1, 1, 1, 1, 1, 1, 1, 1, 1, 1, 1, 1, 1, 1, 1, 1, 1, 1, 1, 1, 1, 1, 1, 1, 1, 1, 1, 1, 1, 4 ),
 ( 0.000000000000000000, 0.01696016684112855444, 0.03526043942249579982, 0.05280277254187595859, 0.06993090526874458368, 0.08694163804313619071, 0.1040119350351715183, 0.1210139405588608608, 0.1379792171159070213, 0.1553986424958138379, 0.1736039501722520528, 0.1924119339504002102, 0.2116998327295473159, 0.2316504953696774671, 0.2523434511079291065, 0.2735071578860145403, 0.2951461022590910477, 0.3179819391660329009, 0.3428270683969382726, 0.3704763703089106741, 0.4013842106079443250, 0.4356267894623512271, 0.4731822280981954343, 0.5126799690798767850, 0.5516183454030080258, 0.5879427231221451278, 0.6209690717414463323, 0.6502633940987105898, 0.6759717312850139770, 0.6991685419836422000, 0.7210175260783882045, 0.7426211155567139510, 0.7640811388048153185, 0.7847659435495429880, 0.8046277674085308140, 0.8239473966552022244, 0.8426767883169219431, 0.8606205966378885908, 0.8779797588928679453, 0.8951189492511466561, 0.9121717320952801300, 0.9291919606104406260, 0.9463734364297033963, 0.9639783248497096890, 0.9823161612921426089, 1.000000000000000000 ),
 .UNSPECIFIED. ) 
 CURVE ( )  GEOMETRIC_REPRESENTATION_ITEM ( )  RATIONAL_B_SPLINE_CURVE ( ( 1.171573005652648991, 1.171573005652649213, 1.171573005652648991, 1.171573005652648991, 1.171573005652648991, 1.171573005652648991, 1.171573005652648991, 1.171573005652648991, 1.171573005652648991, 1.171573005652648991, 1.171573005652648991, 1.171573005652648991, 1.171573005652648991, 1.171573005652648991, 1.171573005652648991, 1.171573005652648991, 1.171573005652648991, 1.171573005652648991, 1.171573005652648991, 1.171573005652648991, 1.171573005652648991, 1.171573005652648991, 1.171573005652648991, 1.171573005652648991, 1.171573005652648991, 1.171573005652648991, 1.171573005652648991, 1.171573005652648991, 1.171573005652648991, 1.171573005652648991, 1.171573005652648991, 1.171573005652648991, 1.171573005652648991, 1.171573005652648991, 1.171573005652648991, 1.171573005652648991, 1.171573005652648991, 1.171573005652648991, 1.171573005652648991, 1.171573005652648991, 1.171573005652648991, 1.171573005652648991, 1.171573005652648991, 1.171573005652648991, 1.171573005652648991, 1.171573005652648991, 1.171573005652648991, 1.171573005652648991 ) ) 
 REPRESENTATION_ITEM ( '' )  );
#2982=CARTESIAN_POINT ( 'NONE',  ( 7.818484572095996121, -11.08186606788998674, -302.4229045757450081 ) ) ;
#2988=CARTESIAN_POINT ( 'NONE',  ( -16.88803284296001905, 5.077274453104001495, -302.5071922382879279 ) ) ;
#2989=CARTESIAN_POINT ( 'NONE',  ( 14.74960734804001916, -8.445183187697006488, 318.8802828394900644 ) ) ;
#2990=CARTESIAN_POINT ( 'NONE',  ( -8.519003879469000395, -8.390442916014999142, -314.8616023057000461 ) ) ;
#2991=CARTESIAN_POINT ( 'NONE',  ( -1.388768300183999882, 9.421618921053999784, 315.0848619657999734 ) ) ;
#2994=CARTESIAN_POINT ( 'NONE',  ( -19.79199150660973672, -1.880421430186972165, 190.9999999999995737 ) ) ;
#3001=EDGE_CURVE ( 'NONE', #1085, #6747, #6203, .T. ) ;
#3003=CARTESIAN_POINT ( 'NONE',  ( -20.00000000000000000, 3.518725546161979705E-10, 191.0000000000000000 ) ) ;
#3004=CARTESIAN_POINT ( 'NONE',  ( -16.99996037728000076, 1.352916535802999941E-09, -314.9999801883000146 ) ) ;
#3008=CARTESIAN_POINT ( 'NONE',  ( -2.450863364448387482, 9.399909383054032119, -315.0000000000000000 ) ) ;
#3009=CARTESIAN_POINT ( 'NONE',  ( -11.98038374875001111, 9.553300872651998787, 189.9229057364800042 ) ) ;
#3010=CARTESIAN_POINT ( 'NONE',  ( 1.604641703582619039, 9.999988110349836035, 314.4999449211996989 ) ) ;
#3015=CARTESIAN_POINT ( 'NONE',  ( 16.33370887135086491, -2.613387004688928261, 315.0000000000000568 ) ) ;
#3016=CARTESIAN_POINT ( 'NONE',  ( 10.41198510038999991, 7.677033091942000453, -314.8616023057000461 ) ) ;
#3018=CARTESIAN_POINT ( 'NONE',  ( 15.40147079910000372, 7.455286574312999903, 320.0770942683900557 ) ) ;
#3022=CARTESIAN_POINT ( 'NONE',  ( -16.01024372474999069, 7.613620273433004293, -317.0792622552969533 ) ) ;
#3029=CARTESIAN_POINT ( 'NONE',  ( 19.12867493021229137, -3.682770601350499717, 319.0000000000003979 ) ) ;
#3030=ORIENTED_EDGE ( 'NONE', *, *, #4040, .T. ) ;
#3031=CARTESIAN_POINT ( 'NONE',  ( 4.978134047761749947, 12.12024670600909282, -316.5000000000004547 ) ) ;
#3033=CARTESIAN_POINT ( 'NONE',  ( -2.450606348566487735, -9.399923241459493539, 315.0000000000000568 ) ) ;
#3034=CARTESIAN_POINT ( 'NONE',  ( -13.92883798546999508, -9.075834183867002025, -302.9207377450070453 ) ) ;
#3037=CARTESIAN_POINT ( 'NONE',  ( -15.69672544750998888, 7.226176219113002119, -302.4229045757450081 ) ) ;
#3041=CARTESIAN_POINT ( 'NONE',  ( -14.67553856548000013, -5.592168771406000438, -314.4150829855000211 ) ) ;
#3042=CARTESIAN_POINT ( 'NONE',  ( -19.99999036626000048, -4.642009783819999925E-09, -316.5000000000000000 ) ) ;
#3044=CARTESIAN_POINT ( 'NONE',  ( -8.712128322569002492, -10.82186910204999997, 189.9229057364800042 ) ) ;
#3046=CARTESIAN_POINT ( 'NONE',  ( -16.34529002343606052, 7.216405960070773951, 190.9999999999996589 ) ) ;
#3050=CARTESIAN_POINT ( 'NONE',  ( -14.67553856548000013, -5.592168771406000438, 314.4150829855000211 ) ) ;
#3052=VECTOR ( 'NONE', #8481, 1000.000000000000000 ) ;
#3054=CARTESIAN_POINT ( 'NONE',  ( -7.560581757588001217, -10.42594579828999990, 319.9928079742500131 ) ) ;
#3055=CARTESIAN_POINT ( 'NONE',  ( -5.334282155825492033, -9.025044196641820449, -314.9999999999999432 ) ) ;
#3057=CARTESIAN_POINT ( 'NONE',  ( 11.28781796570999951, 4.951468039558000633, 315.0000000000000000 ) ) ;
#3060=CARTESIAN_POINT ( 'NONE',  ( 4.461988713456979561, 9.163769885065249809, -314.9999999999999432 ) ) ;
#3061=CARTESIAN_POINT ( 'NONE',  ( -18.75323799499002675, 4.519634888734000100, 190.4207385301700128 ) ) ;
#3062=CARTESIAN_POINT ( 'NONE',  ( -10.23467949614885697, 10.00000000050611781, -302.5000000000003979 ) ) ;
#3064=CARTESIAN_POINT ( 'NONE',  ( 11.71572875766478639, -12.49999999885353041, -316.5000000000000000 ) ) ;
#3067=CARTESIAN_POINT ( 'NONE',  ( -9.314945463565893036, -11.07333627012143396, -303.4999999999996589 ) ) ;
#3068=CARTESIAN_POINT ( 'NONE',  ( 17.12450099635000100, -0.4005340032738999856, -314.8616023057000461 ) ) ;
#3069=CARTESIAN_POINT ( 'NONE',  ( 17.40348243411531826, -5.898854857574459487, 314.4999507458385892 ) ) ;
#3070=CARTESIAN_POINT ( 'NONE',  ( -19.59086175841999378, 0.09594170647769999227, 320.0770942683900557 ) ) ;
#3074=CARTESIAN_POINT ( 'NONE',  ( -6.660995095996002924, 11.36691212455000333, -317.5770954168139610 ) ) ;
#3079=CARTESIAN_POINT ( 'NONE',  ( -12.32405526929588291, 7.045528031251309997, -314.5741454722275421 ) ) ;
#3082=CARTESIAN_POINT ( 'NONE',  ( -13.47608353327723485, -6.291341891605536141, -314.5797986957608146 ) ) ;
#3084=CARTESIAN_POINT ( 'NONE',  ( -2.055855549839187280, 12.45069410617974448, -316.5000000000004547 ) ) ;
#3085=ORIENTED_EDGE ( 'NONE', *, *, #5584, .T. ) ;
#3086=CARTESIAN_POINT ( 'NONE',  ( -7.042505780985288233, -8.656073623659681360, 315.0000000000000000 ) ) ;
#3087=CARTESIAN_POINT ( 'NONE',  ( -10.38823308980000704, -10.24279834975000192, -302.4229045757450081 ) ) ;
#3092=CARTESIAN_POINT ( 'NONE',  ( 0.1616652313949000219, 12.09676013415999485, -302.4229045757450081 ) ) ;
#3093=CARTESIAN_POINT ( 'NONE',  ( -14.04143820182998503, -8.903536631273988533, 318.8802828394900644 ) ) ;
#3095=CARTESIAN_POINT ( 'NONE',  ( -3.932702496464000497, -9.868769537474999964, -314.4150829855000211 ) ) ;
#3096=CARTESIAN_POINT ( 'NONE',  ( 10.18931492271999950, 9.698324433322001781, -302.5000000000000000 ) ) ;
#3097=EDGE_LOOP ( 'NONE', ( #1420, #7294, #6137, #4139 ) ) ;
#3098=CARTESIAN_POINT ( 'NONE',  ( -12.81613682183999536, -9.130924732858002102, 189.9229057364800042 ) ) ;
#3099=CARTESIAN_POINT ( 'NONE',  ( -19.99999721801999897, -7.771324026006999692E-11, 191.0000000000000000 ) ) ;
#3103=CARTESIAN_POINT ( 'NONE',  ( -8.450675645183000739, -8.177559542660000957, 315.0848619657999734 ) ) ;
#3105=CARTESIAN_POINT ( 'NONE',  ( 16.29068328802999943, 5.892689959824000567, 320.0000000000000000 ) ) ;
#3106=CARTESIAN_POINT ( 'NONE',  ( -17.30539973653000629, -4.527429531397997309, 319.9928079742500131 ) ) ;
#3109=FACE_OUTER_BOUND ( 'NONE', #6004, .T. ) ;
#3114=CARTESIAN_POINT ( 'NONE',  ( 19.56991616969001058, -0.3941640562313002416, 189.9229057364800042 ) ) ;
#3115=CARTESIAN_POINT ( 'NONE',  ( 9.995120280747379127, 8.217201865419340834, 314.4999464406708967 ) ) ;
#3116=CARTESIAN_POINT ( 'NONE',  ( 20.00000000000000000, 4.642020101641720348E-09, -316.5000000000000000 ) ) ;
#3117=CARTESIAN_POINT ( 'NONE',  ( 17.50000000000000711, -8.653813013134384923E-10, -302.5000000000000568 ) ) ;
#3119=CARTESIAN_POINT ( 'NONE',  ( -13.88908508137762077, -9.009716997455477383, -303.4999999999996589 ) ) ;
#3120=CARTESIAN_POINT ( 'NONE',  ( -18.99987386368999864, -0.5560526133780999691, -302.5000000001010108 ) ) ;
#3124=CARTESIAN_POINT ( 'NONE',  ( -9.773738012405997821, 10.46865777734000424, 320.0770942683900557 ) ) ;
#3128=CARTESIAN_POINT ( 'NONE',  ( 9.065820074235004356, 10.71255845790999572, -317.5770954168139610 ) ) ;
#3129=CARTESIAN_POINT ( 'NONE',  ( -20.01656911870001920, -0.3693805509907998053, -316.3802825947000201 ) ) ;
#3132=DIRECTION ( 'NONE',  ( 1.000000000000000000, 0.000000000000000000, 0.000000000000000000 ) ) ;
#3134=VECTOR ( 'NONE', #264, 1000.000000000000000 ) ;
#3136=B_SPLINE_CURVE_WITH_KNOTS ( 'NONE', 3,
 ( #1244, #2109, #2863, #4520 ),
 .UNSPECIFIED., .F., .F.,
 ( 4, 4 ),
 ( 0.000000000000000000, 1.000000000000000000 ),
 .UNSPECIFIED. ) ;
#3140=CARTESIAN_POINT ( 'NONE',  ( 9.914941699848354162, -10.86515064494810545, 319.0000000000003979 ) ) ;
#3144=CARTESIAN_POINT ( 'NONE',  ( -14.08994485310920730, -5.290256584484003710, 314.9999999999999432 ) ) ;
#3145=CARTESIAN_POINT ( 'NONE',  ( -0.1616652313949000219, -12.09676013415999485, -302.4229045757450081 ) ) ;
#3148=CARTESIAN_POINT ( 'NONE',  ( -10.54839116401999988, 10.71567991178000057, -302.9207377450070453 ) ) ;
#3151=CARTESIAN_POINT ( 'NONE',  ( 18.68148959551998445, -4.475099553145003739, 318.8802828394900644 ) ) ;
#3153=CARTESIAN_POINT ( 'NONE',  ( -11.89238025184999792, -6.701939844102000166, -315.0848619657999734 ) ) ;
#3156=CARTESIAN_POINT ( 'NONE',  ( -19.59059457349998823, -0.06993619660353000977, 189.9229057364800042 ) ) ;
#3160=CARTESIAN_POINT ( 'NONE',  ( -6.273744347102000241, -8.772995918477999311, 315.0848619657999734 ) ) ;
#3161=DIRECTION ( 'NONE',  ( 1.000000000000000000, 0.000000000000000000, 0.000000000000000000 ) ) ;
#3163=CARTESIAN_POINT ( 'NONE',  ( -16.26474538691000049, 5.919460245093000061, 320.0000000000000000 ) ) ;
#3166=CARTESIAN_POINT ( 'NONE',  ( -17.50000000088855501, -5.867334121986932161, -302.5000000000001705 ) ) ;
#3172=CARTESIAN_POINT ( 'NONE',  ( 9.832070176257998284, 10.44777315889000313, 189.9229057364800042 ) ) ;
#3175=AXIS2_PLACEMENT_3D ( 'NONE', #2875, #513, #9384 ) ;
#3176=COLOUR_RGB ( '', 0.40784314, 0.44705882, 0.49803922) ;
#3177=CARTESIAN_POINT ( 'NONE',  ( -19.99998650234397957, 8.894530543673175064E-07, -302.9142199863263158 ) ) ;
#3178=CARTESIAN_POINT ( 'NONE',  ( 12.85811403544582099, -9.588400772462145838, -303.5000000000006253 ) ) ;
#3179=CARTESIAN_POINT ( 'NONE',  ( 16.89608781496000134, 0.5923740909019999945, -315.0848619657999734 ) ) ;
#3181=CARTESIAN_POINT ( 'NONE',  ( -18.99998114578000141, 0.3144692935366000253, 190.0000000000100044 ) ) ;
#3182=CARTESIAN_POINT ( 'NONE',  ( 19.56990143371999125, -0.3944980022354002136, 320.0770942683900557 ) ) ;
#3186=CARTESIAN_POINT ( 'NONE',  ( 15.92039057294001125, 7.578271297757998681, -316.3802825947000201 ) ) ;
#3187=CARTESIAN_POINT ( 'NONE',  ( -12.80442074722001067, -9.608322671940996429, -316.3802825947000201 ) ) ;
#3190=CARTESIAN_POINT ( 'NONE',  ( 13.36276382026999876, -8.154196903800000840, 320.0000000000000000 ) ) ;
#3192=PLANE ( 'NONE',  #5139 ) ;
#3196=CARTESIAN_POINT ( 'NONE',  ( 18.68762439754708637, -4.478870766961967398, 319.0000000000003979 ) ) ;
#3200=CARTESIAN_POINT ( 'NONE',  ( -1.573733331195987573, -9.469132543440894167, 315.0000000000001137 ) ) ;
#3201=CARTESIAN_POINT ( 'NONE',  ( -19.56012101500002132, 0.5268190066377996805, -302.4229045757450081 ) ) ;
#3207=CARTESIAN_POINT ( 'NONE',  ( 19.37583693248997108, 3.422417436021003123, -302.9207377450070453 ) ) ;
#3210=CARTESIAN_POINT ( 'NONE',  ( 8.620760283086999820, -8.357092890497000326, -314.8616023057000461 ) ) ;
#3211=DIRECTION ( 'NONE',  ( -5.235554895604999868E-10, -4.130579097307000442E-10, 1.000000000000000000 ) ) ;
#3213=CARTESIAN_POINT ( 'NONE',  ( -18.86321946521001180, 0.4765678057151996327, 190.0071920248299477 ) ) ;
#3214=CARTESIAN_POINT ( 'NONE',  ( 19.14871320452657599, 3.641870911972380220, 190.9999999999996589 ) ) ;
#3217=CARTESIAN_POINT ( 'NONE',  ( -17.20518503178000103, -1.389427005613000032, 314.6383426456000052 ) ) ;
#3218=CARTESIAN_POINT ( 'NONE',  ( -2.579601697407999605, 11.41110358643000033, 320.0000000000000000 ) ) ;
#3221=CARTESIAN_POINT ( 'NONE',  ( -6.040317665795909008, 11.93081507280031239, 319.0000000000005116 ) ) ;
#3227=CARTESIAN_POINT ( 'NONE',  ( -20.00000000068207129, -7.322330470855613171, -316.5000000000000000 ) ) ;
#3230=CARTESIAN_POINT ( 'NONE',  ( 11.72170966038013162, -10.14138702413947790, -303.4999999999996589 ) ) ;
#3234=CARTESIAN_POINT ( 'NONE',  ( 19.98292278601002181, -0.4165571180016003350, 318.8802828394900644 ) ) ;
#3238=CARTESIAN_POINT ( 'NONE',  ( 6.484736462136006629, 11.91614536315999828, -317.0792622552969533 ) ) ;
#3241=CARTESIAN_POINT ( 'NONE',  ( -4.804283134583999804, -11.13634285072000019, 320.0000000000000000 ) ) ;
#3243=DIRECTION ( 'NONE',  ( 1.000000000000000000, 0.000000000000000000, 0.000000000000000000 ) ) ;
#3244=CARTESIAN_POINT ( 'NONE',  ( -1.669371716897545710, -9.454742746653563401, -315.0000000000000000 ) ) ;
#3246=CARTESIAN_POINT ( 'NONE',  ( -12.98706127646999953, 6.788989183774999603, -315.0000000000001137 ) ) ;
#3248=CARTESIAN_POINT ( 'NONE',  ( -16.14934711101999909, 6.043101335943000585, -317.5000000000000000 ) ) ;
#3249=ORIENTED_EDGE ( 'NONE', *, *, #5471, .F. ) ;
#3250=CARTESIAN_POINT ( 'NONE',  ( 1.678162365823997915, -12.55068027652000140, -302.9207377450070453 ) ) ;
#3256=CARTESIAN_POINT ( 'NONE',  ( 7.921361508960999664, 11.05315760980000661, -302.4229045757450081 ) ) ;
#3259=CARTESIAN_POINT ( 'NONE',  ( -16.78232460783999969, -3.056336161456999712, -314.4150829855000211 ) ) ;
#3260=ADVANCED_FACE ( 'NONE', ( #1398, #604 ), #3877, .T. ) ;
#3261=CARTESIAN_POINT ( 'NONE',  ( -16.90171868104999930, -0.3834349726278000192, 315.0848619657999734 ) ) ;
#3263=CARTESIAN_POINT ( 'NONE',  ( -14.91611818836001824, -6.947523351336002406, 190.0071920248299477 ) ) ;
#3264=CARTESIAN_POINT ( 'NONE',  ( 19.99996770037257221, 0.3054858693455833052, 190.9999999999996589 ) ) ;
#3268=CARTESIAN_POINT ( 'NONE',  ( -16.39086977655999888, -2.839079766962000040, 314.8616023057000461 ) ) ;
#3270=CARTESIAN_POINT ( 'NONE',  ( -5.939701018627000728, 10.93065061464000109, 320.0000000000000000 ) ) ;
#3271=CARTESIAN_POINT ( 'NONE',  ( 9.773738012405997821, -10.46865777734000424, 320.0770942683900557 ) ) ;
#3272=CARTESIAN_POINT ( 'NONE',  ( -4.393607043691841518, 12.21170385155075344, 319.0000000000005116 ) ) ;
#3275=VECTOR ( 'NONE', #3747, 1000.000000000000000 ) ;
#3279=CARTESIAN_POINT ( 'NONE',  ( 13.12098914876195366, 6.031629431400056696, 314.9999999999999432 ) ) ;
#3280=CARTESIAN_POINT ( 'NONE',  ( -17.50000000000000000, 0.000000000000000000, -315.0000000000000000 ) ) ;
#3281=CARTESIAN_POINT ( 'NONE',  ( -18.32212638522000248, -3.124911926288000075, -302.5000000000129603 ) ) ;
#3286=VERTEX_POINT ( 'NONE', #5317 ) ;
#3287=CARTESIAN_POINT ( 'NONE',  ( 15.97383562432999149, 7.643564190274003245, -317.0792622552969533 ) ) ;
#3289=CARTESIAN_POINT ( 'NONE',  ( 5.939701018627000728, -10.93065061464000109, 320.0000000000000000 ) ) ;
#3294=CARTESIAN_POINT ( 'NONE',  ( 8.717693564518029348, -8.144027366771089405, -314.9999999999999432 ) ) ;
#3296=CARTESIAN_POINT ( 'NONE',  ( 17.50000000000107292, 0.7437989020622546299, -314.4963898845653603 ) ) ;
#3298=CARTESIAN_POINT ( 'NONE',  ( -18.32558628770999931, 3.116746082530000184, -317.4999999999870397 ) ) ;
#3299=ORIENTED_EDGE ( 'NONE', *, *, #10436, .F. ) ;
#3300=CARTESIAN_POINT ( 'NONE',  ( 15.02162735728999543, -8.365494092177003793, -302.9207377450070453 ) ) ;
#3301=CARTESIAN_POINT ( 'NONE',  ( 18.78102408959999536, -1.459157757289999413, -317.4928077629770087 ) ) ;
#3304=CARTESIAN_POINT ( 'NONE',  ( 15.00000000000326139, -5.136019918588313243E-17, 315.0000000000001137 ) ) ;
#3308=CARTESIAN_POINT ( 'NONE',  ( -17.80660862177001746, 5.847896592537999538, -302.9207377450070453 ) ) ;
#3311=CARTESIAN_POINT ( 'NONE',  ( -16.25556153634000367, -3.885850782616000032, -314.4150829855000211 ) ) ;
#3314=ORIENTED_EDGE ( 'NONE', *, *, #3389, .F. ) ;
#3315=CARTESIAN_POINT ( 'NONE',  ( -8.858368459239001069, -11.29793033041000250, 190.4207385301700128 ) ) ;
#3320=CARTESIAN_POINT ( 'NONE',  ( 16.21525914616999842, -2.693567875512000054, 315.0848619657999734 ) ) ;
#3323=CARTESIAN_POINT ( 'NONE',  ( 8.650961417647998530, -10.84061383582999838, 320.0770942683900557 ) ) ;
#3324=CARTESIAN_POINT ( 'NONE',  ( 9.075831286667817466, 11.14872141952138840, 319.0000000000005116 ) ) ;
#3325=CARTESIAN_POINT ( 'NONE',  ( 19.30523607465251956, 3.390426274888739488, -303.4999999999990905 ) ) ;
#3326=CARTESIAN_POINT ( 'NONE',  ( 16.90887668763000207, -0.2823175147257999673, 315.0848619657999734 ) ) ;
#3328=CARTESIAN_POINT ( 'NONE',  ( 4.856005603318365615, -12.14126555804866214, 190.9999999999995737 ) ) ;
#3332=EDGE_CURVE ( 'NONE', #9806, #1105, #5508, .T. ) ;
#3335=CARTESIAN_POINT ( 'NONE',  ( -19.58578074103510147, 1.999241607805304935E-07, -302.5000071933975505 ) ) ;
#3340=CARTESIAN_POINT ( 'NONE',  ( 18.32597195921000122, -3.115684853309999891, -302.5000000000129603 ) ) ;
#3346=CARTESIAN_POINT ( 'NONE',  ( 2.381287040813000348E-07, -10.00000001404999850, 190.0000000000000000 ) ) ;
#3347=CARTESIAN_POINT ( 'NONE',  ( -15.95659996325998087, 7.548489772182000124, -316.3802825947000201 ) ) ;
#3352=CARTESIAN_POINT ( 'NONE',  ( -15.68033135863999838, -6.468544937636000469, 320.0000000000000000 ) ) ;
#3355=CARTESIAN_POINT ( 'NONE',  ( 0.7884827272773687890, -9.499887003984508027, -315.0000000000000000 ) ) ;
#3357=CARTESIAN_POINT ( 'NONE',  ( -0.9204674644685997276, -9.999779064329263889, -314.4999424967812729 ) ) ;
#3358=ORIENTED_EDGE ( 'NONE', *, *, #10436, .T. ) ;
#3359=CARTESIAN_POINT ( 'NONE',  ( 16.13706688435999581, 6.055114415286000806, -317.5000000000000000 ) ) ;
#3361=CARTESIAN_POINT ( 'NONE',  ( -1.983590419337998734, -12.44807596301999908, -303.6197174156509391 ) ) ;
#3363=CARTESIAN_POINT ( 'NONE',  ( 12.34703828426001770, -8.590819132751997600, -317.4928077629770087 ) ) ;
#3364=CARTESIAN_POINT ( 'NONE',  ( 14.79012398733999945, -1.483731117707000058, 315.0000000000000000 ) ) ;
#3365=EDGE_CURVE ( 'NONE', #8331, #4467, #10585, .T. ) ;
#3367=CARTESIAN_POINT ( 'NONE',  ( -17.49957620160848393, -0.4465025224747954380, 314.4999504925934275 ) ) ;
#3370=CARTESIAN_POINT ( 'NONE',  ( 5.145495120689000501, 11.07694361959999974, -302.5000000000000000 ) ) ;
#3372=CARTESIAN_POINT ( 'NONE',  ( -13.97596040350999402, -9.042973024665997173, 190.4207385301700128 ) ) ;
#3373=CARTESIAN_POINT ( 'NONE',  ( -17.50000000000125056, -1.338989683019597976E-14, -315.0000000000000568 ) ) ;
#3374=CARTESIAN_POINT ( 'NONE',  ( 11.69624556101560664, 6.874206995516638052, -315.0000000000000000 ) ) ;
#3376=CARTESIAN_POINT ( 'NONE',  ( 10.00032506892000406, 10.91649673191999526, 190.4207385301700128 ) ) ;
#3377=ORIENTED_EDGE ( 'NONE', *, *, #2024, .F. ) ;
#3378=ORIENTED_EDGE ( 'NONE', *, *, #810, .F. ) ;
#3382=CARTESIAN_POINT ( 'NONE',  ( 16.20020866270998638, -5.814836367836996978, 319.9928079742500131 ) ) ;
#3383=CARTESIAN_POINT ( 'NONE',  ( -17.22665784173602788, 1.821305584325311866, 314.4999396030179355 ) ) ;
#3384=SURFACE_STYLE_FILL_AREA ( #3491 ) ;
#3385=CARTESIAN_POINT ( 'NONE',  ( 16.75097866579000083, 2.074182492207000461, 314.8616023057000461 ) ) ;
#3386=ORIENTED_EDGE ( 'NONE', *, *, #10623, .T. ) ;
#3388=EDGE_CURVE ( 'NONE', #245, #9921, #5795, .T. ) ;
#3389=EDGE_CURVE ( 'NONE', #9273, #9531, #10402, .T. ) ;
#3391=CARTESIAN_POINT ( 'NONE',  ( -8.517242506840645433, 8.210459489885888473, 315.0000000000000568 ) ) ;
#3393=EDGE_LOOP ( 'NONE', ( #4194, #2283, #9700, #4269 ) ) ;
#3394=CARTESIAN_POINT ( 'NONE',  ( -6.503149100579999953, -10.80808940222000025, -302.5000000000000000 ) ) ;
#3399=CARTESIAN_POINT ( 'NONE',  ( -11.28781796570999951, 4.951468039558000633, -284.9999999999999432 ) ) ;
#3402=CARTESIAN_POINT ( 'NONE',  ( -9.372233899709991434, 11.04684900435999495, -316.3802825947000201 ) ) ;
#3406=CARTESIAN_POINT ( 'NONE',  ( 15.52898264372802650, -3.840979768096378866, -315.0000000000000000 ) ) ;
#3408=CARTESIAN_POINT ( 'NONE',  ( -17.19853431801041665, 2.231396706186351775, -314.4963898845653603 ) ) ;
#3410=CARTESIAN_POINT ( 'NONE',  ( -10.21957842388999893, 9.686567771335999666, -317.5000000000000000 ) ) ;
#3412=CARTESIAN_POINT ( 'NONE',  ( 6.532283844592004840, -11.81967986011000704, -303.6197174156509391 ) ) ;
#3413=CARTESIAN_POINT ( 'NONE',  ( -12.29114107644999443, -8.620527874443991934, -317.4928077629770087 ) ) ;
#3414=CARTESIAN_POINT ( 'NONE',  ( -16.77957632114000219, 1.244976636274000015, -315.0848619657999734 ) ) ;
#3416=CARTESIAN_POINT ( 'NONE',  ( -15.96001947224000794, 7.545661119572996789, -303.6197174156520759 ) ) ;
#3421=CARTESIAN_POINT ( 'NONE',  ( 17.00602911426001285, -6.582783228486000837, 191.1197171614399792 ) ) ;
#3422=CARTESIAN_POINT ( 'NONE',  ( 0.000000000000000000, -10.54711710274999881, -315.0000000000001137 ) ) ;
#3423=CARTESIAN_POINT ( 'NONE',  ( 16.13978190921854861, 2.966266463780219187, -314.9999999999999432 ) ) ;
#3425=CARTESIAN_POINT ( 'NONE',  ( -14.03700484701000484, 9.005201968871000773, 190.4207385301700128 ) ) ;
#3428=CARTESIAN_POINT ( 'NONE',  ( 16.10362618234000109, -3.713712614977999760, 314.6383426456000052 ) ) ;
#3430=CARTESIAN_POINT ( 'NONE',  ( -4.863072958136998025, -11.71397411138000422, 320.0770942683900557 ) ) ;
#3433=CARTESIAN_POINT ( 'NONE',  ( 13.31399140613000043, 6.082710156904999721, 314.8616023057000461 ) ) ;
#3437=CARTESIAN_POINT ( 'NONE',  ( -14.79708307774000353, 8.514882941861998233, 319.5792614743400009 ) ) ;
#3443=CARTESIAN_POINT ( 'NONE',  ( -13.37739799451331457, 5.841934623551301442, 315.0000000000000000 ) ) ;
#3458=CARTESIAN_POINT ( 'NONE',  ( 11.84501012641003825, -6.794057347756047527, -315.0000000000000000 ) ) ;
#3460=ORIENTED_EDGE ( 'NONE', *, *, #4238, .F. ) ;
#3462=CARTESIAN_POINT ( 'NONE',  ( 3.763664787428660841, -12.29131725939111419, -316.5000000000004547 ) ) ;
#3466=CARTESIAN_POINT ( 'NONE',  ( 7.926044316621995378, -11.48136605963999024, -303.6197174156509391 ) ) ;
#3467=CARTESIAN_POINT ( 'NONE',  ( 11.29610983636999144, -9.103527074753996473, -317.4928077629770087 ) ) ;
#3472=CARTESIAN_POINT ( 'NONE',  ( -7.926044316621995378, 11.48136605963999024, -303.6197174156509391 ) ) ;
#3475=CARTESIAN_POINT ( 'NONE',  ( -17.34710322845000263, 0.4172063223308000168, -314.6383426456000052 ) ) ;
#3476=CARTESIAN_POINT ( 'NONE',  ( -6.328188536734999481, 10.84734154703999920, -302.5000000000000000 ) ) ;
#3479=CARTESIAN_POINT ( 'NONE',  ( -6.124940582141004342, -11.99257230354999315, 190.4207385301700128 ) ) ;
#3481=CARTESIAN_POINT ( 'NONE',  ( 13.89455516181870465, 5.448669939092228631, -315.0000000000000000 ) ) ;
#3482=CARTESIAN_POINT ( 'NONE',  ( 19.21810730420998681, 3.675731523933000400, 190.4207385301700128 ) ) ;
#3485=CARTESIAN_POINT ( 'NONE',  ( 16.76545246634000108, -2.037063237379999947, 314.8616023057000461 ) ) ;
#3489=CARTESIAN_POINT ( 'NONE',  ( -19.55138120870000407, -0.8505817651195003437, 320.0770942683900557 ) ) ;
#3490=CARTESIAN_POINT ( 'NONE',  ( -16.56500303248389372, 3.264221055421775652, 314.4999403627584229 ) ) ;
#3491=FILL_AREA_STYLE ('',( #9831 ) ) ;
#3492=CARTESIAN_POINT ( 'NONE',  ( 13.56771446467999986, 6.451120369226999607, 314.4150829855000211 ) ) ;
#3493=ORIENTED_EDGE ( 'NONE', *, *, #3523, .F. ) ;
#3494=CARTESIAN_POINT ( 'NONE',  ( 19.12881201168725198, -3.682481340332637743, 190.9999999999995737 ) ) ;
#3496=CARTESIAN_POINT ( 'NONE',  ( 15.70899585331000559, 7.847162746392004173, 319.5792614743400009 ) ) ;
#3498=CARTESIAN_POINT ( 'NONE',  ( 2.545396798794703042, 9.391972178232515844, 315.0000000000000568 ) ) ;
#3503=PLANE ( 'NONE',  #929 ) ;
#3507=CARTESIAN_POINT ( 'NONE',  ( 13.35558048726000635, 8.018799577237007981, 190.0071920248299477 ) ) ;
#3509=VECTOR ( 'NONE', #6454, 1000.000000000000000 ) ;
#3513=CARTESIAN_POINT ( 'NONE',  ( -10.02545106797885310, -7.672278800222116502, -315.0000000000000000 ) ) ;
#3514=ORIENTED_EDGE ( 'NONE', *, *, #8088, .F. ) ;
#3516=CARTESIAN_POINT ( 'NONE',  ( -4.978134047761750836, -12.12024670600909459, -316.5000000000004547 ) ) ;
#3520=VECTOR ( 'NONE', #3211, 1000.000000000000000 ) ;
#3522=CARTESIAN_POINT ( 'NONE',  ( -13.35621109890998959, 8.022534180767001644, -317.4928077629770087 ) ) ;
#3523=EDGE_CURVE ( 'NONE', #9383, #4786, #6703, .T. ) ;
#3525=CARTESIAN_POINT ( 'NONE',  ( 12.67153153313999070, -9.210367834107003659, -317.5770954168139610 ) ) ;
#3526=CARTESIAN_POINT ( 'NONE',  ( -16.60805916514000202, 2.908391789136000050, -314.6383426456000052 ) ) ;
#3527=CARTESIAN_POINT ( 'NONE',  ( -6.532283844592004840, 11.81967986011000704, -303.6197174156520759 ) ) ;
#3528=CARTESIAN_POINT ( 'NONE',  ( 9.526067998327799539E-10, -10.00000000005854339, 314.4999528359535361 ) ) ;
#3530=CARTESIAN_POINT ( 'NONE',  ( 18.78737820286000115, -1.762683282930000095, 190.0000000000000000 ) ) ;
#3531=CARTESIAN_POINT ( 'NONE',  ( -7.649658656166000270, 10.52693506402999901, -302.5000000000000000 ) ) ;
#3533=CARTESIAN_POINT ( 'NONE',  ( 20.08953225942999765, -0.1031351683529000418, 190.4207385301700128 ) ) ;
#3535=CARTESIAN_POINT ( 'NONE',  ( 16.88803284296001905, -5.077274453104001495, -302.5071922382879279 ) ) ;
#3537=CARTESIAN_POINT ( 'NONE',  ( -18.68134283559999531, 4.475435185431997809, 191.1197171614399792 ) ) ;
#3540=CARTESIAN_POINT ( 'NONE',  ( 10.49789511286000021, -7.639556387670999982, 314.8616023057000461 ) ) ;
#3542=CARTESIAN_POINT ( 'NONE',  ( 12.02088824526999211, -10.08549396686999522, 319.5792614743400009 ) ) ;
#3543=CARTESIAN_POINT ( 'NONE',  ( -11.54108038788630708, 7.525558202395652430, 314.4999425153563948 ) ) ;
#3544=CARTESIAN_POINT ( 'NONE',  ( -19.99999035944999903, 7.277427703818000446E-10, -303.5000000000000000 ) ) ;
#3545=CARTESIAN_POINT ( 'NONE',  ( 17.12450099635000100, -0.4005340032738999856, 314.8616023057000461 ) ) ;
#3548=CARTESIAN_POINT ( 'NONE',  ( -4.404324556173000005, 12.28809208595000335, 319.5792614743400009 ) ) ;
#3551=CARTESIAN_POINT ( 'NONE',  ( 4.648656036509398959, 9.134414902114890822, 315.0000000000000568 ) ) ;
#3554=CARTESIAN_POINT ( 'NONE',  ( -9.006891093149000938, -10.12158591819999920, -302.5000000000000000 ) ) ;
#3556=CARTESIAN_POINT ( 'NONE',  ( 8.548650239411999863, 10.26553531915999962, 190.0000000000000000 ) ) ;
#3557=CARTESIAN_POINT ( 'NONE',  ( -16.99996037728000076, 1.352916535802999941E-09, -314.9999801883000146 ) ) ;
#3558=CARTESIAN_POINT ( 'NONE',  ( -18.86316454545999832, -0.4769905026584997931, 190.0071920248299477 ) ) ;
#3565=CARTESIAN_POINT ( 'NONE',  ( 14.96969266857001557, 6.905075921034003805, 319.9928079742500131 ) ) ;
#3566=CARTESIAN_POINT ( 'NONE',  ( -15.92495094281444601, -7.583842622554347379, -316.5000000000004547 ) ) ;
#3570=CARTESIAN_POINT ( 'NONE',  ( -6.508337484872001255, 10.68452134396000375, -317.4928077629770087 ) ) ;
#3572=CARTESIAN_POINT ( 'NONE',  ( -7.885457619219000236, -11.57957576882999184, -317.0792622552969533 ) ) ;
#3577=CARTESIAN_POINT ( 'NONE',  ( 10.19111349739211292, -9.999999999041103038, 314.9999999999999432 ) ) ;
#3579=CARTESIAN_POINT ( 'NONE',  ( -12.50247260085999912, -8.641513563414997989, 190.0000000000000000 ) ) ;
#3584=ORIENTED_EDGE ( 'NONE', *, *, #3700, .F. ) ;
#3585=CARTESIAN_POINT ( 'NONE',  ( -16.53777229716873265, -2.187293290751350483, 315.0000000000000000 ) ) ;
#3586=CARTESIAN_POINT ( 'NONE',  ( -18.77308876972001173, -1.495304374661000413, -302.5071922382879279 ) ) ;
#3587=CARTESIAN_POINT ( 'NONE',  ( 20.08919666923998903, 0.07462331497654001167, 190.4207385301700128 ) ) ;
#3590=CARTESIAN_POINT ( 'NONE',  ( 18.18877801098002323, 4.514014122889999037, -302.4229045757450081 ) ) ;
#3591=CARTESIAN_POINT ( 'NONE',  ( -1.330908921489000418, -12.56946842516999041, 319.5792614743400009 ) ) ;
#3592=CARTESIAN_POINT ( 'NONE',  ( 16.97404422732000029, -2.118410180888999683, -314.6383426456000052 ) ) ;
#3593=CARTESIAN_POINT ( 'NONE',  ( -8.759386130138000937, 8.782224002452998946, 314.4150829855000211 ) ) ;
#3595=CARTESIAN_POINT ( 'NONE',  ( 11.67891759455000056, -8.922363378240000031, 190.0071920248299477 ) ) ;
#3596=ORIENTED_EDGE ( 'NONE', *, *, #6260, .F. ) ;
#3597=CARTESIAN_POINT ( 'NONE',  ( 18.70581557644998938, 4.435354026251000725, 318.8802828394900644 ) ) ;
#3598=( BOUNDED_SURFACE ( )  B_SPLINE_SURFACE ( 3, 1, ( 
 ( #4942, #3876 ),
 ( #3227, #1455 ),
 ( #7153, #7260 ),
 ( #10424, #6504 ),
 ( #3064, #8869 ),
 ( #9784, #2423 ),
 ( #3116, #4738 ) ),
 .UNSPECIFIED., .F., .F., .T. ) 
 B_SPLINE_SURFACE_WITH_KNOTS ( ( 4, 3, 4 ),
 ( 2, 2 ),
 ( 0.000000000000000000, 0.5000000000000000000, 1.000000000000000000 ),
 ( 0.000000000000000000, 1.000000000000000000 ),
 .UNSPECIFIED. ) 
 GEOMETRIC_REPRESENTATION_ITEM ( )  RATIONAL_B_SPLINE_SURFACE ( (
 ( 1.000000000000000000, 1.000000000000000000),
 ( 0.8047378540737379904, 0.8047378540737379904),
 ( 0.8047378540737379904, 0.8047378540737379904),
 ( 1.000000000000000000, 1.000000000000000000),
 ( 0.8047378540737379904, 0.8047378540737379904),
 ( 0.8047378540737379904, 0.8047378540737379904),
 ( 1.000000000000000000, 1.000000000000000000) ) ) 
 REPRESENTATION_ITEM ( '' )  SURFACE ( )  );
#3602=CARTESIAN_POINT ( 'NONE',  ( 8.717521301463110106, 8.144085127293724469, 314.9999999999999432 ) ) ;
#3603=CARTESIAN_POINT ( 'NONE',  ( 11.71572875238734213, -12.50000000010304113, 319.0000000000000568 ) ) ;
#3604=AXIS2_PLACEMENT_3D ( 'NONE', #4267, #9317, #9103 ) ;
#3607=CARTESIAN_POINT ( 'NONE',  ( 15.64479012893000132, 6.500532800106000764, 190.0000000000000000 ) ) ;
#3609=CARTESIAN_POINT ( 'NONE',  ( -13.41272981818000432, 7.983430642947998201, 190.0071920248299477 ) ) ;
#3615=CARTESIAN_POINT ( 'NONE',  ( 11.72570362167166635, -6.858483604278664103, 315.0000000000000000 ) ) ;
#3616=CARTESIAN_POINT ( 'NONE',  ( -4.061138133959000029, 9.851562218542998295, -314.4150829855000211 ) ) ;
#3617=B_SPLINE_CURVE_WITH_KNOTS ( 'NONE', 3,
 ( #669, #1524, #4806, #8079, #721, #130, #5007, #1636, #1737, #7489, #4104, #1846, #8394, #9104, #3406, #7384, #1792, #6740, #4910, #8188, #2441, #5711, #8996, #6575, #8234, #872, #4320, #8286, #925, #10014, #5810, #19, #2602, #3458, #7538, #7436, #6521, #9155, #6681, #2655, #5923, #825, #9803, #3294, #9050, #4213, #5063, #9960, #1032, #9214, #5117, #5761, #10602, #185, #5863, #1686, #8343, #9857, #2496, #4960, #4158, #73, #6631, #3355, #981, #9908, #3244, #2546, #4268, #1284, #10413, #2251, #589, #7590, #8689, #9558, #3752, #8581, #3055, #2197, #4613, #7888, #5466, #8745, #4505, #239, #1227, #5413, #1387, #3513, #484, #4671, #7043, #9454, #6990, #2041, #10261, #8637, #6935, #3868, #7782, #6323, #10312, #4562, #535, #3809, #2949, #2149, #7097, #2092, #9406, #10213, #6222, #7946, #9612, #7835, #5309, #7145, #9507, #428, #3705, #2898, #5519, #1334, #10362, #3004 ),
 .UNSPECIFIED., .F., .F.,
 ( 4, 1, 1, 1, 1, 1, 2, 2, 1, 1, 1, 1, 1, 2, 2, 1, 1, 1, 1, 1, 2, 2, 1, 1, 1, 1, 1, 2, 2, 1, 1, 1, 1, 1, 1, 2, 2, 1, 1, 1, 1, 1, 2, 2, 1, 1, 2, 2, 2, 1, 1, 2, 2, 1, 1, 1, 1, 2, 2, 1, 1, 1, 1, 1, 1, 2, 2, 1, 1, 1, 1, 1, 2, 2, 1, 1, 1, 1, 1, 2, 2, 1, 1, 1, 1, 1, 2, 2, 1, 1, 1, 1, 2, 2, 4 ),
 ( 0.000000000000000000, 0.06250000000000707767, 0.09375000000001063039, 0.1093750000000124206, 0.1171875000000132255, 0.1210937500000135308, 0.1230468750000135864, 0.1250000000000136280, 0.1562500000000150158, 0.1718750000000157374, 0.1796875000000160982, 0.1835937500000163480, 0.1855468750000164591, 0.1865234375000165423, 0.1875000000000166256, 0.2187500000000192069, 0.2343750000000205669, 0.2421875000000212608, 0.2460937500000216493, 0.2480468750000218991, 0.2490234375000220102, 0.2500000000000220934, 0.2812500000000249245, 0.2968750000000263678, 0.3046875000000271450, 0.3085937500000274780, 0.3105468750000275890, 0.3115234375000275890, 0.3125000000000275335, 0.3437500000000278666, 0.3593750000000280886, 0.3671875000000281997, 0.3710937500000282552, 0.3730468750000283107, 0.3740234375000284217, 0.3745117187500284217, 0.3750000000000284217, 0.4062500000000292544, 0.4218750000000296985, 0.4296875000000299205, 0.4335937500000300315, 0.4355468750000300870, 0.4365234375000300870, 0.4375000000000300315, 0.4531250000000301426, 0.4609375000000301981, 0.4648437500000302536, 0.4687500000000303091, 0.5000000000000306422, 0.5156250000000307532, 0.5234375000000308642, 0.5273437500000308642, 0.5312500000000308642, 0.5468750000000310862, 0.5546875000000311973, 0.5585937500000311973, 0.5605468750000311973, 0.5615234375000311973, 0.5625000000000311973, 0.5937500000000296430, 0.6093750000000288658, 0.6171875000000285327, 0.6210937500000284217, 0.6230468750000283107, 0.6240234375000283107, 0.6245117187500283107, 0.6250000000000283107, 0.6562500000000291989, 0.6718750000000295319, 0.6796875000000297540, 0.6835937500000298650, 0.6855468750000299760, 0.6865234375000299760, 0.6875000000000299760, 0.7187500000000309752, 0.7343750000000314193, 0.7421875000000316414, 0.7460937500000317524, 0.7480468750000318634, 0.7490234375000318634, 0.7500000000000318634, 0.7812500000000318634, 0.7968750000000317524, 0.8046875000000317524, 0.8085937500000317524, 0.8105468750000316414, 0.8115234375000315303, 0.8125000000000314193, 0.8437500000000285327, 0.8593750000000272005, 0.8671875000000265343, 0.8710937500000260902, 0.8730468750000258682, 0.8750000000000255351, 1.000000000000000000 ),
 .UNSPECIFIED. ) ;
#3619=CARTESIAN_POINT ( 'NONE',  ( -4.237945188771000460, 11.10223611999999704, 319.9928079742500131 ) ) ;
#3621=CARTESIAN_POINT ( 'NONE',  ( -19.86381236214655033, -1.775476277371077716, -316.5000000000004547 ) ) ;
#3624=CARTESIAN_POINT ( 'NONE',  ( 4.800908653447998553, 11.01413625319999845, -317.4928077629770087 ) ) ;
#3625=CARTESIAN_POINT ( 'NONE',  ( 19.95938911887002831, -1.720557998077001827, -317.0792622552969533 ) ) ;
#3627=CARTESIAN_POINT ( 'NONE',  ( 10.00000000000000000, -2.500000000000000000, -285.0000000000000000 ) ) ;
#3630=CARTESIAN_POINT ( 'NONE',  ( 14.24871951745999965, -7.583581010724000038, 190.0000000000000000 ) ) ;
#3637=CARTESIAN_POINT ( 'NONE',  ( 12.03935733796000562, 9.983683518723006856, 191.1197171614399792 ) ) ;
#3638=CARTESIAN_POINT ( 'NONE',  ( -19.99999721801999897, -7.771324026006999692E-11, 191.0000000000000000 ) ) ;
#3640=CARTESIAN_POINT ( 'NONE',  ( 19.85665319583999988, -1.941121513171000901, 319.5792614743400009 ) ) ;
#3642=CARTESIAN_POINT ( 'NONE',  ( 16.92217352393999974, -0.01966449385449000123, -315.0848619657999734 ) ) ;
#3643=CARTESIAN_POINT ( 'NONE',  ( -4.031301020048999817, 9.630010295875997883, 314.6383426456000052 ) ) ;
#3645=CARTESIAN_POINT ( 'NONE',  ( 6.173727351415999820, -10.75865019063000183, 190.0071920248299477 ) ) ;
#3650=CARTESIAN_POINT ( 'NONE',  ( 20.00000000000000000, 0.000000000000000000, 191.0000000000000000 ) ) ;
#3655=CARTESIAN_POINT ( 'NONE',  ( -16.99964540243389521, 0.4333634660859943533, -315.0000000000000568 ) ) ;
#3656=CARTESIAN_POINT ( 'NONE',  ( -6.173727351415999820, 10.75865019063000183, 190.0071920248299477 ) ) ;
#3661=CARTESIAN_POINT ( 'NONE',  ( 11.54746845216141082, -6.952771041492575854, 315.0000000000000000 ) ) ;
#3662=CARTESIAN_POINT ( 'NONE',  ( -14.43094748301999886, 5.211771040651000497, -314.8616023057000461 ) ) ;
#3664=CARTESIAN_POINT ( 'NONE',  ( -13.31009360926000085, 8.046300872832002682, 319.9928079742500131 ) ) ;
#3668=CARTESIAN_POINT ( 'NONE',  ( -16.90418428017002839, -6.814536637555997700, -317.0792622552969533 ) ) ;
#3671=( BOUNDED_SURFACE ( )  B_SPLINE_SURFACE ( 3, 3, ( 
 ( #3558, #1893, #9459, #1180, #10220, #10267, #8491, #4413, #1133, #7688, #7637, #332, #6839, #8643, #3609, #7584, #6892, #7739, #10159, #383, #9261, #3656, #6942, #6996, #2802, #6074, #2855, #6123, #9364, #1998, #5164, #5263, #231, #9411, #10108, #3507, #2046, #5314, #8587, #6019, #10061, #1234, #434, #2904, #5969, #8437, #4364, #2750, #9313, #10316 ),
 ( #1451, #3815, #2204, #489, #8057, #5418, #6390, #4678, #649, #9670, #7101, #4568, #3974, #4736, #8008, #4788, #3009, #7257, #1289, #5634, #10420, #10368, #702, #6284, #7842, #3925, #5524, #2369, #2313, #9513, #10526, #3172, #5582, #3757, #7048, #8806, #9564, #7204, #598, #8694, #9728, #2956, #1507, #10472, #1340, #6227, #2154, #4621, #3114, #7893 ),
 ( #540, #5474, #8751, #1394, #7952, #3874, #6332, #3061, #7151, #8865, #6446, #9617, #2257, #6815, #3425, #7613, #6705, #896, #7509, #5833, #8364, #1708, #9288, #7669, #1001, #4182, #10087, #6653, #10036, #310, #5887, #3376, #2728, #1868, #151, #1920, #8416, #4235, #7455, #4394, #4289, #7561, #206, #3482, #9236, #1819, #8465, #3587, #5192, #9181 ),
 ( #5084, #6867, #6763, #2680, #5949, #9930, #1108, #3537, #5137, #1056, #4340, #5996, #261, #9126, #4981, #2566, #10136, #8258, #2777, #8916, #99, #1761, #9982, #8311, #5031, #2624, #951, #8564, #9339, #2127, #10297, #7128, #3791, #3637, #9540, #2180, #10345, #10395, #1161, #2934, #1210, #6201, #5338, #2834, #3846, #8519, #6259, #9487, #6103, #6048 ) ),
 .UNSPECIFIED., .F., .F., .T. ) 
 B_SPLINE_SURFACE_WITH_KNOTS ( ( 4, 4 ),
 ( 4, 1, 1, 1, 1, 1, 1, 1, 1, 1, 1, 1, 1, 1, 1, 1, 1, 1, 1, 1, 1, 1, 1, 1, 1, 1, 1, 1, 1, 1, 1, 1, 1, 1, 1, 1, 1, 1, 1, 1, 1, 1, 1, 1, 1, 1, 1, 4 ),
 ( 0.000000000000000000, 1.000000000000000000 ),
 ( -0.008478179454678999930, 0.000000000000000000, 0.01942502340896999982, 0.03767429839031000149, 0.05516856733836000143, 0.07225070737889999206, 0.08921661857028999332, 0.1062419522249000020, 0.1231986756591000043, 0.1401197909732000146, 0.1574955775699000138, 0.1756558812635999889, 0.1944176066207999876, 0.2136589569993999904, 0.2335613621991999844, 0.2542018781120999882, 0.2753083038155999529, 0.2968879296931000167, 0.3196642413612000300, 0.3444503751709999673, 0.3720414184181000117, 0.4028839481288000179, 0.4370422198952000348, 0.4744802605176999810, 0.5138140658555000462, 0.5525504936030000147, 0.5886556970966999591, 0.6214671571023999697, 0.6505675624772999655, 0.6761140898808000177, 0.6991730762615999684, 0.7208971548058999979, 0.7423774111579999335, 0.7637103432859999597, 0.7842694365818000390, 0.8040102150915000578, 0.8232128915810998926, 0.8418292181656999995, 0.8596651317910000145, 0.8769212066234000069, 0.8939598742608000359, 0.9109129999441000214, 0.9278339763510999871, 0.9449158864711000305, 0.9624195949295000219, 0.9806529035300000086, 1.000000000000000000, 1.007725586608000157 ),
 .UNSPECIFIED. ) 
 GEOMETRIC_REPRESENTATION_ITEM ( )  RATIONAL_B_SPLINE_SURFACE ( (
 ( 1.236576749365999817, 1.236576749365999817, 1.236576749365999817, 1.236576749365999817, 1.236576749365999817, 1.236576749365999817, 1.236576749365999817, 1.236576749365999817, 1.236576749365999817, 1.236576749365999817, 1.236576749365999817, 1.236576749365999817, 1.236576749365999817, 1.236576749365999817, 1.236576749365999817, 1.236576749365999817, 1.236576749365999817, 1.236576749365999817, 1.236576749365999817, 1.236576749365999817, 1.236576749365999817, 1.236576749365999817, 1.236576749365999817, 1.236576749365999817, 1.236576749365999817, 1.236576749365999817, 1.236576749365999817, 1.236576749365999817, 1.236576749365999817, 1.236576749365999817, 1.236576749365999817, 1.236576749365999817, 1.236576749365999817, 1.236576749365999817, 1.236576749365999817, 1.236576749365999817, 1.236576749365999817, 1.236576749365999817, 1.236576749365999817, 1.236576749365999817, 1.236576749365999817, 1.236576749365999817, 1.236576749365999817, 1.236576749365999817, 1.236576749365999817, 1.236576749365999817, 1.236576749365999817, 1.236576749365999817, 1.236576749365999817, 1.236576749365999817),
 ( 0.9211410835446999235, 0.9211410835446999235, 0.9211410835446999235, 0.9211410835446999235, 0.9211410835446999235, 0.9211410835446999235, 0.9211410835446999235, 0.9211410835446999235, 0.9211410835446999235, 0.9211410835446999235, 0.9211410835446999235, 0.9211410835446999235, 0.9211410835446999235, 0.9211410835446999235, 0.9211410835446999235, 0.9211410835446999235, 0.9211410835446999235, 0.9211410835446999235, 0.9211410835446999235, 0.9211410835446999235, 0.9211410835446999235, 0.9211410835446999235, 0.9211410835446999235, 0.9211410835446999235, 0.9211410835446999235, 0.9211410835446999235, 0.9211410835446999235, 0.9211410835446999235, 0.9211410835446999235, 0.9211410835446999235, 0.9211410835446999235, 0.9211410835446999235, 0.9211410835446999235, 0.9211410835446999235, 0.9211410835446999235, 0.9211410835446999235, 0.9211410835446999235, 0.9211410835446999235, 0.9211410835446999235, 0.9211410835446999235, 0.9211410835446999235, 0.9211410835446999235, 0.9211410835446999235, 0.9211410835446999235, 0.9211410835446999235, 0.9211410835446999235, 0.9211410835446999235, 0.9211410835446999235, 0.9211410835446999235, 0.9211410835446999235),
 ( 0.9211410835446999235, 0.9211410835446999235, 0.9211410835446999235, 0.9211410835446999235, 0.9211410835446999235, 0.9211410835446999235, 0.9211410835446999235, 0.9211410835446999235, 0.9211410835446999235, 0.9211410835446999235, 0.9211410835446999235, 0.9211410835446999235, 0.9211410835446999235, 0.9211410835446999235, 0.9211410835446999235, 0.9211410835446999235, 0.9211410835446999235, 0.9211410835446999235, 0.9211410835446999235, 0.9211410835446999235, 0.9211410835446999235, 0.9211410835446999235, 0.9211410835446999235, 0.9211410835446999235, 0.9211410835446999235, 0.9211410835446999235, 0.9211410835446999235, 0.9211410835446999235, 0.9211410835446999235, 0.9211410835446999235, 0.9211410835446999235, 0.9211410835446999235, 0.9211410835446999235, 0.9211410835446999235, 0.9211410835446999235, 0.9211410835446999235, 0.9211410835446999235, 0.9211410835446999235, 0.9211410835446999235, 0.9211410835446999235, 0.9211410835446999235, 0.9211410835446999235, 0.9211410835446999235, 0.9211410835446999235, 0.9211410835446999235, 0.9211410835446999235, 0.9211410835446999235, 0.9211410835446999235, 0.9211410835446999235, 0.9211410835446999235),
 ( 1.236576749365999817, 1.236576749365999817, 1.236576749365999817, 1.236576749365999817, 1.236576749365999817, 1.236576749365999817, 1.236576749365999817, 1.236576749365999817, 1.236576749365999817, 1.236576749365999817, 1.236576749365999817, 1.236576749365999817, 1.236576749365999817, 1.236576749365999817, 1.236576749365999817, 1.236576749365999817, 1.236576749365999817, 1.236576749365999817, 1.236576749365999817, 1.236576749365999817, 1.236576749365999817, 1.236576749365999817, 1.236576749365999817, 1.236576749365999817, 1.236576749365999817, 1.236576749365999817, 1.236576749365999817, 1.236576749365999817, 1.236576749365999817, 1.236576749365999817, 1.236576749365999817, 1.236576749365999817, 1.236576749365999817, 1.236576749365999817, 1.236576749365999817, 1.236576749365999817, 1.236576749365999817, 1.236576749365999817, 1.236576749365999817, 1.236576749365999817, 1.236576749365999817, 1.236576749365999817, 1.236576749365999817, 1.236576749365999817, 1.236576749365999817, 1.236576749365999817, 1.236576749365999817, 1.236576749365999817, 1.236576749365999817, 1.236576749365999817) ) ) 
 REPRESENTATION_ITEM ( '' )  SURFACE ( )  );
#3673=CARTESIAN_POINT ( 'NONE',  ( 17.50000000000000000, 0.000000000000000000, -315.0000000000000000 ) ) ;
#3676=CARTESIAN_POINT ( 'NONE',  ( 14.90286285339066019, 5.148601615201705783, -314.5782021036098968 ) ) ;
#3686=CARTESIAN_POINT ( 'NONE',  ( -0.1580967862520001599, -11.39739484195000330, -302.5071922382879279 ) ) ;
#3691=CARTESIAN_POINT ( 'NONE',  ( 18.27982664221999443, 2.925785484622998922, -302.5071922382879279 ) ) ;
#3692=CARTESIAN_POINT ( 'NONE',  ( -13.19336277821000536, -9.492603533888004819, 319.5792614743400009 ) ) ;
#3693=CARTESIAN_POINT ( 'NONE',  ( 17.59298685096999648, -0.02218567204016000036, -314.4150829855000211 ) ) ;
#3694=CARTESIAN_POINT ( 'NONE',  ( 1.285290206351000108, 10.09749793447999977, 314.4150829855000211 ) ) ;
#3696=CARTESIAN_POINT ( 'NONE',  ( -19.96251415050936728, -0.9422375983257673671, 190.9999999999995737 ) ) ;
#3699=FACE_BOUND ( 'NONE', #6668, .T. ) ;
#3700=EDGE_CURVE ( 'NONE', #189, #1010, #900, .T. ) ;
#3701=CARTESIAN_POINT ( 'NONE',  ( -17.14610219660000112, -0.04370646908743999748, 314.8616023057000461 ) ) ;
#3702=CARTESIAN_POINT ( 'NONE',  ( -16.35728328174216273, 2.567538628164302228, 315.0000000000000568 ) ) ;
#3704=PRODUCT_DEFINITION_FORMATION_WITH_SPECIFIED_SOURCE ( 'ANY', '', #1232, .NOT_KNOWN. ) ;
#3705=CARTESIAN_POINT ( 'NONE',  ( -16.33391464646021518, -2.612996577909529883, -315.0000000000000000 ) ) ;
#3706=CARTESIAN_POINT ( 'NONE',  ( -20.00000000024866864, 25.00000000007771561, 191.0000000000000000 ) ) ;
#3709=CARTESIAN_POINT ( 'NONE',  ( 20.00000000000000000, 0.000000000000000000, -316.5000000000000000 ) ) ;
#3711=B_SPLINE_CURVE_WITH_KNOTS ( 'NONE', 3,
 ( #3557, #3655, #6073, #4310, #9363, #5262, #8537, #9951, #5054, #1944, #7581, #5212, #1892, #6787, #9145, #973, #1179, #4460, #10059, #2700, #5163, #8435, #1075, #4363, #278, #10219, #3756, #9410, #1606, #3813, #2407, #5675, #1288, #10266, #10367, #7100, #6941, #2903, #5313, #8586, #3712, #3873, #6994, #7150, #1393, #8749, #6172, #2854, #7788, #6226, #6122, #4676, #596, #7951, #2953, #8642, #9458, #1231, #2097, #7841, #2045, #3008, #6283, #9769, #9512, #488, #9562, #2203, #2152, #1339, #5473, #4567, #8960, #10418, #3060, #5362, #6491, #4878, #5417, #7047, #8156, #794, #539, #4509, #433, #10315, #8693, #4619, #7892, #8415, #9821, #8308, #9878, #949, #3374, #843, #1867, #6543, #4288, #4233, #4127, #2622, #3481, #205, #5728, #1653, #2461, #7352, #894, #9018, #9235, #7507, #10034, #2678, #9071, #7403, #149, #3423, #4073, #42, #4929, #1706, #5884, #4979, #8206, #2515 ),
 .UNSPECIFIED., .F., .F.,
 ( 4, 1, 1, 1, 1, 1, 2, 2, 1, 1, 1, 1, 1, 2, 2, 1, 1, 1, 1, 1, 2, 2, 1, 1, 1, 1, 1, 2, 2, 1, 1, 1, 1, 1, 1, 2, 2, 1, 1, 1, 1, 1, 2, 2, 1, 1, 2, 2, 2, 1, 1, 2, 2, 1, 1, 1, 1, 2, 2, 1, 1, 1, 1, 1, 1, 2, 2, 1, 1, 1, 1, 1, 2, 2, 1, 1, 1, 1, 1, 2, 2, 1, 1, 1, 1, 1, 2, 2, 1, 1, 1, 1, 2, 2, 4 ),
 ( 0.000000000000000000, 0.06250000000000710543, 0.09375000000001064426, 0.1093750000000124206, 0.1171875000000132394, 0.1210937500000135447, 0.1230468750000136002, 0.1250000000000136557, 0.1562500000000150158, 0.1718750000000157097, 0.1796875000000160705, 0.1835937500000162925, 0.1855468750000164035, 0.1865234375000164868, 0.1875000000000165701, 0.2187500000000191513, 0.2343750000000204836, 0.2421875000000211775, 0.2460937500000215383, 0.2480468750000217881, 0.2490234375000218991, 0.2500000000000219824, 0.2812500000000247580, 0.2968750000000262013, 0.3046875000000269784, 0.3085937500000273115, 0.3105468750000274225, 0.3115234375000274225, 0.3125000000000274225, 0.3437500000000277556, 0.3593750000000279776, 0.3671875000000280886, 0.3710937500000281442, 0.3730468750000281997, 0.3740234375000283107, 0.3745117187500283107, 0.3750000000000283107, 0.4062500000000291434, 0.4218750000000295319, 0.4296875000000297540, 0.4335937500000298650, 0.4355468750000299205, 0.4365234375000299205, 0.4375000000000299205, 0.4531250000000300315, 0.4609375000000300870, 0.4648437500000301426, 0.4687500000000301981, 0.5000000000000304201, 0.5156250000000306422, 0.5234375000000307532, 0.5273437500000307532, 0.5312500000000307532, 0.5468750000000309752, 0.5546875000000310862, 0.5585937500000310862, 0.5605468750000310862, 0.5615234375000310862, 0.5625000000000310862, 0.5937500000000295319, 0.6093750000000287548, 0.6171875000000284217, 0.6210937500000283107, 0.6230468750000281997, 0.6240234375000281997, 0.6245117187500281997, 0.6250000000000283107, 0.6562500000000291989, 0.6718750000000295319, 0.6796875000000297540, 0.6835937500000298650, 0.6855468750000299760, 0.6865234375000299760, 0.6875000000000299760, 0.7187500000000308642, 0.7343750000000313083, 0.7421875000000315303, 0.7460937500000316414, 0.7480468750000317524, 0.7490234375000317524, 0.7500000000000317524, 0.7812500000000317524, 0.7968750000000316414, 0.8046875000000316414, 0.8085937500000316414, 0.8105468750000315303, 0.8115234375000314193, 0.8125000000000313083, 0.8437500000000284217, 0.8593750000000270894, 0.8671875000000264233, 0.8710937500000259792, 0.8730468750000257572, 0.8750000000000255351, 1.000000000000000000 ),
 .UNSPECIFIED. ) ;
#3712=CARTESIAN_POINT ( 'NONE',  ( -9.142617743994909674, 7.997268146336696581, -315.0000000000000568 ) ) ;
#3716=CARTESIAN_POINT ( 'NONE',  ( 0.000000000000000000, 0.000000000000000000, 315.0000000000000000 ) ) ;
#3717=CARTESIAN_POINT ( 'NONE',  ( 16.13945612244922501, -2.966804785441415238, 314.9999999999999432 ) ) ;
#3718=CARTESIAN_POINT ( 'NONE',  ( 14.52969073417999901, 5.422537850045999974, -314.6383426456000052 ) ) ;
#3720=CARTESIAN_POINT ( 'NONE',  ( 9.801936311039993299, 9.714404437230999889, 319.9928079742500131 ) ) ;
#3724=CARTESIAN_POINT ( 'NONE',  ( -18.29581373626999508, 2.889895519923001643, -317.4928077629770087 ) ) ;
#3725=CARTESIAN_POINT ( 'NONE',  ( 18.63147570264002084, -4.749337304460001796, -317.0792622552969533 ) ) ;
#3727=CARTESIAN_POINT ( 'NONE',  ( -17.50000000000000000, 0.000000000000000000, -315.0000000000000000 ) ) ;
#3728=CARTESIAN_POINT ( 'NONE',  ( -0.9068124364724808872, 10.00021929074745231, -314.4998859403474398 ) ) ;
#3730=CARTESIAN_POINT ( 'NONE',  ( -10.60011422839999895, -9.531420659438001763, 190.0000000000000000 ) ) ;
#3733=CARTESIAN_POINT ( 'NONE',  ( -14.79481407445002183, -8.414248563823001348, 191.1197171614399792 ) ) ;
#3735=CARTESIAN_POINT ( 'NONE',  ( 8.907970405212992659, -10.02857016715000604, -302.5071922382879279 ) ) ;
#3739=CARTESIAN_POINT ( 'NONE',  ( -1.615578127792000274, 11.35484692374000737, -302.5071922382879279 ) ) ;
#3740=CARTESIAN_POINT ( 'NONE',  ( -17.64852322130001738, -5.886271888320000478, 318.8802828394900644 ) ) ;
#3742=CARTESIAN_POINT ( 'NONE',  ( -16.41165915566000066, 2.800979832323999830, 314.8616023057000461 ) ) ;
#3744=CARTESIAN_POINT ( 'NONE',  ( 9.745026809365992193, -9.735374599634990744, 190.0071920248299477 ) ) ;
#3745=ORIENTED_EDGE ( 'NONE', *, *, #1436, .T. ) ;
#3746=CARTESIAN_POINT ( 'NONE',  ( 11.22625503481000209, 10.34655023142000907, 318.8802828394900644 ) ) ;
#3747=DIRECTION ( 'NONE',  ( -1.000000000000000000, 0.000000000000000000, 0.000000000000000000 ) ) ;
#3750=CARTESIAN_POINT ( 'NONE',  ( -16.74588786138889063, 1.629246332199927538, 315.0000000000000000 ) ) ;
#3752=CARTESIAN_POINT ( 'NONE',  ( -4.578722611353294170, -9.145541810471781830, -315.0000000000000568 ) ) ;
#3753=CARTESIAN_POINT ( 'NONE',  ( -20.00000000024866864, 25.00000000007771561, 319.0000000000000000 ) ) ;
#3756=CARTESIAN_POINT ( 'NONE',  ( -13.98368610735814421, 5.377133503752142829, -315.0000000000000568 ) ) ;
#3757=CARTESIAN_POINT ( 'NONE',  ( 11.86325706386000434, 9.609314883874001012, 189.9229057364800042 ) ) ;
#3758=VERTEX_POINT ( 'NONE', #7461 ) ;
#3764=CARTESIAN_POINT ( 'NONE',  ( 16.83787941357387297, -1.297844089352232944, 315.0000000000000568 ) ) ;
#3765=CARTESIAN_POINT ( 'NONE',  ( -8.690073206612000334, 8.569658446474999636, -314.6383426456000052 ) ) ;
#3767=CARTESIAN_POINT ( 'NONE',  ( 17.33400069613001193, 5.617198899843996784, 320.0770942683900557 ) ) ;
#3771=CARTESIAN_POINT ( 'NONE',  ( -17.80394872498997927, 5.851108818846995518, -317.0792622552969533 ) ) ;
#3773=CARTESIAN_POINT ( 'NONE',  ( -17.39473599676002635, -5.562790558317003864, -317.5770954168139610 ) ) ;
#3775=( BOUNDED_CURVE ( )  B_SPLINE_CURVE ( 3, ( #4208, #7482, #6625, #3346 ),
 .UNSPECIFIED., .F., .T. ) 
 B_SPLINE_CURVE_WITH_KNOTS ( ( 4, 4 ),
 ( 1.013329913875473588E-09, 1.000000000000000000 ),
 .UNSPECIFIED. ) 
 CURVE ( )  GEOMETRIC_REPRESENTATION_ITEM ( )  RATIONAL_B_SPLINE_CURVE ( ( 0.9922218186767667314, 0.8003084390180068564, 0.8029011661257512422, 1.000000000000000000 ) ) 
 REPRESENTATION_ITEM ( '' )  );
#3776=CARTESIAN_POINT ( 'NONE',  ( -12.98706127646999953, -6.788989183774999603, -315.0000000000000000 ) ) ;
#3783=CARTESIAN_POINT ( 'NONE',  ( -11.72056399716000108, 9.035224326960999974, 190.0000000000000000 ) ) ;
#3784=CARTESIAN_POINT ( 'NONE',  ( 0.6338995735901449269, -12.51432109910909851, 319.0000000000003979 ) ) ;
#3786=CARTESIAN_POINT ( 'NONE',  ( 15.61478958302000208, -7.813810907915007320, 191.1197171614399792 ) ) ;
#3787=ORIENTED_EDGE ( 'NONE', *, *, #4113, .T. ) ;
#3788=CARTESIAN_POINT ( 'NONE',  ( -1.514431797236434930E-09, -10.00000000000000000, -302.5000000000000000 ) ) ;
#3789=CARTESIAN_POINT ( 'NONE',  ( 13.72185241754999652, -8.618935511841003816, -302.4229045757450081 ) ) ;
#3791=CARTESIAN_POINT ( 'NONE',  ( 11.02833964697000013, 10.42949886550000826, 191.1197171614399792 ) ) ;
#3794=CARTESIAN_POINT ( 'NONE',  ( 19.56012101500002132, -0.5268190066377996805, -302.4229045757450081 ) ) ;
#3796=CARTESIAN_POINT ( 'NONE',  ( 17.50000000000000000, 0.000000000000000000, -315.0000000000000000 ) ) ;
#3797=CARTESIAN_POINT ( 'NONE',  ( -6.419414596134000561, -9.427679607337001499, -314.4150829855000211 ) ) ;
#3798=CARTESIAN_POINT ( 'NONE',  ( -17.59298685096999648, 0.02218567204014999794, 314.4150829855000211 ) ) ;
#3799=ORIENTED_EDGE ( 'NONE', *, *, #6141, .T. ) ;
#3800=CARTESIAN_POINT ( 'NONE',  ( 18.89081873304001036, -0.08752760549137006407, 190.0071920248299477 ) ) ;
#3801=CARTESIAN_POINT ( 'NONE',  ( -6.038923639677001631, 11.92375595181999870, 318.8802828394900644 ) ) ;
#3808=CARTESIAN_POINT ( 'NONE',  ( -17.50000000000000000, 1.896400240175167841E-08, 314.4999014931028682 ) ) ;
#3809=CARTESIAN_POINT ( 'NONE',  ( -13.95711901494857088, -5.398584340276485705, -315.0000000000000000 ) ) ;
#3813=CARTESIAN_POINT ( 'NONE',  ( -13.12058949809353514, 6.031889286829743568, -315.0000000000000568 ) ) ;
#3815=CARTESIAN_POINT ( 'NONE',  ( -19.57080534385999471, -0.3817780055853002841, 189.9229057364800042 ) ) ;
#3816=CARTESIAN_POINT ( 'NONE',  ( 6.176342442900598861, 9.366307578403514356, 314.4999456809352978 ) ) ;
#3819=CARTESIAN_POINT ( 'NONE',  ( 7.807700195763000117, -10.48319479899000051, -317.5000000000000000 ) ) ;
#3821=CARTESIAN_POINT ( 'NONE',  ( 15.06605725946605112, -4.378913172242680396, 314.9999999999999432 ) ) ;
#3822=CARTESIAN_POINT ( 'NONE',  ( -1.409290114754000012, 9.868237606049000021, -314.6383426456000052 ) ) ;
#3825=CARTESIAN_POINT ( 'NONE',  ( -7.392698694382005442, 11.19283382348000622, 320.0770942683900557 ) ) ;
#3829=CARTESIAN_POINT ( 'NONE',  ( -19.95938911887002831, 1.720557998077001827, -317.0792622552969533 ) ) ;
#3835=CARTESIAN_POINT ( 'NONE',  ( -7.592156631695000435, 10.54118908926000131, 190.0000000000000000 ) ) ;
#3837=CARTESIAN_POINT ( 'NONE',  ( -17.50000000158811986, -0.4607171203178571650, -314.4995147730188023 ) ) ;
#3842=CARTESIAN_POINT ( 'NONE',  ( -9.619189022994751426, -7.822639675800805215, 315.0000000000000000 ) ) ;
#3843=CARTESIAN_POINT ( 'NONE',  ( 17.42451203059000520, -5.527343733032997974, -302.4229045757450081 ) ) ;
#3846=CARTESIAN_POINT ( 'NONE',  ( 19.50564046359999537, 2.789525877152000621, 191.1197171614399792 ) ) ;
#3847=ORIENTED_EDGE ( 'NONE', *, *, #9891, .T. ) ;
#3850=CLOSED_SHELL ( 'NONE', ( #2883, #9333, #8529, #8597, #3260 ) ) ;
#3851=CARTESIAN_POINT ( 'NONE',  ( -7.818484572095996121, 11.08186606788998674, -302.4229045757450081 ) ) ;
#3852=CARTESIAN_POINT ( 'NONE',  ( 19.97284803234999018, 0.5555888903174002191, 318.8802828394900644 ) ) ;
#3853=VERTEX_POINT ( 'NONE', #8620 ) ;
#3854=CARTESIAN_POINT ( 'NONE',  ( -14.23799507159000122, -5.083276007328000112, -315.0848619657999734 ) ) ;
#3856=CARTESIAN_POINT ( 'NONE',  ( 17.62021515802999971, 4.315182425209999728, -302.4999999999969873 ) ) ;
#3858=CARTESIAN_POINT ( 'NONE',  ( -7.457264729102998757, -11.17642278912000720, 189.9229057364800042 ) ) ;
#3859=CARTESIAN_POINT ( 'NONE',  ( -18.68148959551998445, 4.475099553145003739, 318.8802828394900644 ) ) ;
#3863=ORIENTED_EDGE ( 'NONE', *, *, #6141, .F. ) ;
#3864=CARTESIAN_POINT ( 'NONE',  ( -16.58659719219999928, -2.947707964209000053, 314.6383426456000052 ) ) ;
#3865=CARTESIAN_POINT ( 'NONE',  ( 10.19111474148932395, -9.999999291614226848, 315.0000000000000000 ) ) ;
#3866=CARTESIAN_POINT ( 'NONE',  ( -15.26162423979700300, 4.160529437000930031, 314.9999999999999432 ) ) ;
#3867=CARTESIAN_POINT ( 'NONE',  ( -10.79243608611000305, -9.321647281761997306, 319.9928079742500131 ) ) ;
#3868=CARTESIAN_POINT ( 'NONE',  ( -13.37774034208871754, -5.841704189632142885, -315.0000000000001137 ) ) ;
#3873=CARTESIAN_POINT ( 'NONE',  ( -8.900723324022980165, 8.081813809772741664, -315.0000000000000000 ) ) ;
#3874=CARTESIAN_POINT ( 'NONE',  ( -19.56918397773000962, 2.861069655901001152, 190.4207385301700128 ) ) ;
#3876=CARTESIAN_POINT ( 'NONE',  ( -20.00000000000000000, 7.277416212200430041E-10, -303.5000000000000000 ) ) ;
#3877=PLANE ( 'NONE',  #10166 ) ;
#3878=SHAPE_DEFINITION_REPRESENTATION ( #4584, #1806 ) ;
#3882=CARTESIAN_POINT ( 'NONE',  ( -15.57034186525998543, 6.406527364046002759, 319.9928079742500131 ) ) ;
#3886=CARTESIAN_POINT ( 'NONE',  ( 15.65816392223999820, 7.257913545763996055, -317.5770954168139610 ) ) ;
#3887=CARTESIAN_POINT ( 'NONE',  ( -19.12867493021229492, 3.682770601350500606, 319.0000000000005116 ) ) ;
#3888=CARTESIAN_POINT ( 'NONE',  ( -4.976995723842001951, -12.11314212604000318, -316.3802825947000201 ) ) ;
#3890=CARTESIAN_POINT ( 'NONE',  ( -17.48550435259291191, 0.4594173590775618710, -314.5005290240522413 ) ) ;
#3892=CARTESIAN_POINT ( 'NONE',  ( -16.94482484090575269, -2.428629253473818306, -314.5323066871360993 ) ) ;
#3895=CARTESIAN_POINT ( 'NONE',  ( -15.96117728870900088, 7.554047240424474730, -316.5000000000004547 ) ) ;
#3897=CARTESIAN_POINT ( 'NONE',  ( -8.691248314156576171, -8.152891913651146183, 315.0000000000001137 ) ) ;
#3898=CARTESIAN_POINT ( 'NONE',  ( -11.73636226353998779, -10.21860227534999943, -302.9207377450070453 ) ) ;
#3900=ADVANCED_FACE ( 'NONE', ( #364 ), #7639, .T. ) ;
#3901=CARTESIAN_POINT ( 'NONE',  ( -4.978480136836995307, 11.69377972944999478, -302.4229045757450081 ) ) ;
#3903=CARTESIAN_POINT ( 'NONE',  ( -1.327417525529001496, -12.48520226272998990, 318.8802828394900644 ) ) ;
#3905=CARTESIAN_POINT ( 'NONE',  ( 4.061138133959000029, -9.851562218542998295, -314.4150829855000211 ) ) ;
#3908=CARTESIAN_POINT ( 'NONE',  ( 11.00905209676000140, -9.989194338198000622, 189.9229057364800042 ) ) ;
#3910=CARTESIAN_POINT ( 'NONE',  ( 13.01454326516111237, 9.502166178128931051, 190.9999999999996589 ) ) ;
#3915=CARTESIAN_POINT ( 'NONE',  ( -10.50000150490000017, -7.882579085736000302, 314.6383426456000052 ) ) ;
#3918=CARTESIAN_POINT ( 'NONE',  ( -14.93129073739000034, 7.087303338045999546, 320.0000000000000000 ) ) ;
#3919=CARTESIAN_POINT ( 'NONE',  ( 2.482300462934001306, -11.29873291818999803, 319.9928079742500131 ) ) ;
#3925=CARTESIAN_POINT ( 'NONE',  ( 0.7033324871771002851, 12.09174782753000166, 189.9229057364800042 ) ) ;
#3926=FACE_OUTER_BOUND ( 'NONE', #2381, .T. ) ;
#3929=CARTESIAN_POINT ( 'NONE',  ( 16.04008061823806131, 3.141427272462999021, 315.0000000000000000 ) ) ;
#3934=CARTESIAN_POINT ( 'NONE',  ( 19.11656497511998154, 2.646905232783001605, 320.0770942683900557 ) ) ;
#3938=CARTESIAN_POINT ( 'NONE',  ( -5.336288444022999400, 12.13785676344998699, -317.0792622552969533 ) ) ;
#3939=CARTESIAN_POINT ( 'NONE',  ( 2.055393166047998932, -12.44351316864999824, -316.3802825947000201 ) ) ;
#3942=FACE_OUTER_BOUND ( 'NONE', #143, .T. ) ;
#3947=CARTESIAN_POINT ( 'NONE',  ( -9.075831286667817466, -11.14872141952138485, 319.0000000000003979 ) ) ;
#3951=CARTESIAN_POINT ( 'NONE',  ( -4.713955699089914297, -9.123860163919065513, 315.0000000000000568 ) ) ;
#3952=CARTESIAN_POINT ( 'NONE',  ( -18.60584266697000544, -4.788593885995998889, -302.9207377450070453 ) ) ;
#3955=CARTESIAN_POINT ( 'NONE',  ( -6.550050338814993545, 11.90210887660999184, -302.9207377450070453 ) ) ;
#3956=CARTESIAN_POINT ( 'NONE',  ( 15.55726960039999973, -7.859060843840002697, 318.8802828394900644 ) ) ;
#3958=CARTESIAN_POINT ( 'NONE',  ( 8.551447359560999217, -8.144527334518999240, -315.0848619657999734 ) ) ;
#3961=CARTESIAN_POINT ( 'NONE',  ( -10.87058130030999159, -10.04705985032000370, 189.9229057364800042 ) ) ;
#3962=CARTESIAN_POINT ( 'NONE',  ( -10.13048420337591615, 10.78707197045944532, 190.9999999999996589 ) ) ;
#3965=CARTESIAN_POINT ( 'NONE',  ( -15.56325459994999960, -4.731967449628999844, 314.4150829855000211 ) ) ;
#3966=DIRECTION ( 'NONE',  ( 0.000000000000000000, 0.000000000000000000, 1.000000000000000000 ) ) ;
#3967=CARTESIAN_POINT ( 'NONE',  ( 18.20902923167000154, 3.282017551273999967, 320.0000000000000000 ) ) ;
#3968=CARTESIAN_POINT ( 'NONE',  ( 12.43797004353999469, -8.540074035031999244, 319.9928079742500131 ) ) ;
#3969=CARTESIAN_POINT ( 'NONE',  ( 4.928966968695695172, 12.12973353869088200, 319.0000000000005116 ) ) ;
#3972=CARTESIAN_POINT ( 'NONE',  ( 11.28781796570999951, 4.951468039558000633, -285.0000000000000000 ) ) ;
#3974=CARTESIAN_POINT ( 'NONE',  ( -15.36042613538998758, 7.487426557894995227, 189.9229057364800042 ) ) ;
#3978=CARTESIAN_POINT ( 'NONE',  ( -19.99999035944999903, 7.277427703818000446E-10, -303.5000000000000000 ) ) ;
#3980=CARTESIAN_POINT ( 'NONE',  ( 8.037373804805000077, 9.179324345868998591, -315.0000000000000000 ) ) ;
#3981=CARTESIAN_POINT ( 'NONE',  ( 16.39086977655999888, 2.839079766962000040, -314.8616023057000461 ) ) ;
#3986=CARTESIAN_POINT ( 'NONE',  ( -16.03176714517000079, 6.932210726315004123, 320.0770942683900557 ) ) ;
#3989=CARTESIAN_POINT ( 'NONE',  ( 18.92046274781997894, 3.214434834450002221, -317.5770954168139610 ) ) ;
#3990=CARTESIAN_POINT ( 'NONE',  ( 0.2363117521398999110, -12.51008298726001300, -316.3802825947000201 ) ) ;
#3991=CARTESIAN_POINT ( 'NONE',  ( -7.608551686289999338, -10.53686309807999955, 320.0000000000000000 ) ) ;
#3997=ORIENTED_EDGE ( 'NONE', *, *, #1423, .T. ) ;
#3998=( BOUNDED_SURFACE ( )  B_SPLINE_SURFACE ( 3, 3, ( 
 ( #4538, #9338, #7717, #3586, #8464, #5393, #5290, #6972, #7023, #6917, #10189, #6102, #9389, #4393, #2023, #6866, #1055, #7763, #4339, #405, #3686, #2880, #6150, #5995, #2074, #5337, #3735, #8614, #1261, #7816, #462, #10295, #7612, #260, #3535, #6813, #10086, #2727, #1107, #5552, #8840 ),
 ( #3201, #5611, #1422, #8086, #9591, #8779, #6258, #2233, #6473, #7076, #8724, #9755, #1484, #3087, #10344, #10446, #4762, #2179, #10561, #2395, #3145, #1367, #7232, #729, #4815, #2982, #9539, #518, #1315, #5500, #3789, #8673, #4005, #4596, #3843, #7285, #8893, #2287, #7127, #8032, #5446 ),
 ( #4705, #677, #7869, #624, #4650, #3952, #7920, #567, #10394, #7984, #3034, #6307, #3898, #10499, #7177, #1532, #6364, #9645, #6418, #9702, #2342, #3250, #7545, #9914, #934, #988, #9864, #5768, #2502, #6581, #9003, #3300, #4917, #10021, #9056, #6748, #1692, #5816, #4966, #2552, #10608 ),
 ( #8350, #8241, #879, #9111, #1745, #4164, #82, #5014, #7390, #4275, #5869, #8292, #8194, #4219, #7495, #7442, #26, #192, #2608, #3361, #5069, #6638, #136, #6528, #3412, #3466, #4061, #5717, #5661, #6687, #9967, #7337, #9161, #1800, #9809, #8946, #1590, #4866, #1642, #8142, #781 ) ),
 .UNSPECIFIED., .F., .F., .F. ) 
 B_SPLINE_SURFACE_WITH_KNOTS ( ( 4, 4 ),
 ( 4, 1, 1, 1, 1, 1, 1, 1, 1, 1, 1, 1, 1, 1, 1, 1, 1, 1, 1, 1, 1, 1, 1, 1, 1, 1, 1, 1, 1, 1, 1, 1, 1, 1, 1, 1, 1, 1, 4 ),
 ( 0.000000000000000000, 1.000000000000000000 ),
 ( -0.008481365240538999567, 0.000000000000000000, 0.03418499052141999589, 0.06705543243986999968, 0.09609225505224000541, 0.1212689627326999919, 0.1445858237144000136, 0.1683350686350000014, 0.1924153997444999764, 0.2163475385441999965, 0.2400901845063000140, 0.2638872993326000227, 0.2883641926465000394, 0.3138739111173999841, 0.3400736664824999811, 0.3669224033080000225, 0.3952263667259999780, 0.4258975072560999831, 0.4597904367344000098, 0.4962938553987999990, 0.5331571951194999937, 0.5680640359449000698, 0.5998794348263000176, 0.6292819723868000592, 0.6571102200006999627, 0.6841458463841999516, 0.7104758728877998974, 0.7357936615436999617, 0.7602320418247999756, 0.7841586104491999887, 0.8079717864086000123, 0.8319769714029000562, 0.8557114603086999338, 0.8789861807339000022, 0.9040973669459999584, 0.9330567862467999962, 0.9658526712421000582, 1.000000000000000000, 1.007721702948999987 ),
 .UNSPECIFIED. ) 
 GEOMETRIC_REPRESENTATION_ITEM ( )  RATIONAL_B_SPLINE_SURFACE ( (
 ( 1.236577362560999926, 1.236577362560999926, 1.236577362560999926, 1.236577362560999926, 1.236577362560999926, 1.236577362560999926, 1.236577362560999926, 1.236577362560999926, 1.236577362560999926, 1.236577362560999926, 1.236577362560999926, 1.236577362560999926, 1.236577362560999926, 1.236577362560999926, 1.236577362560999926, 1.236577362560999926, 1.236577362560999926, 1.236577362560999926, 1.236577362560999926, 1.236577362560999926, 1.236577362560999926, 1.236577362560999926, 1.236577362560999926, 1.236577362560999926, 1.236577362560999926, 1.236577362560999926, 1.236577362560999926, 1.236577362560999926, 1.236577362560999926, 1.236577362560999926, 1.236577362560999926, 1.236577362560999926, 1.236577362560999926, 1.236577362560999926, 1.236577362560999926, 1.236577362560999926, 1.236577362560999926, 1.236577362560999926, 1.236577362560999926, 1.236577362560999926, 1.236577362560999926),
 ( 0.9211408791463999712, 0.9211408791463999712, 0.9211408791463999712, 0.9211408791463999712, 0.9211408791463999712, 0.9211408791463999712, 0.9211408791463999712, 0.9211408791463999712, 0.9211408791463999712, 0.9211408791463999712, 0.9211408791463999712, 0.9211408791463999712, 0.9211408791463999712, 0.9211408791463999712, 0.9211408791463999712, 0.9211408791463999712, 0.9211408791463999712, 0.9211408791463999712, 0.9211408791463999712, 0.9211408791463999712, 0.9211408791463999712, 0.9211408791463999712, 0.9211408791463999712, 0.9211408791463999712, 0.9211408791463999712, 0.9211408791463999712, 0.9211408791463999712, 0.9211408791463999712, 0.9211408791463999712, 0.9211408791463999712, 0.9211408791463999712, 0.9211408791463999712, 0.9211408791463999712, 0.9211408791463999712, 0.9211408791463999712, 0.9211408791463999712, 0.9211408791463999712, 0.9211408791463999712, 0.9211408791463999712, 0.9211408791463999712, 0.9211408791463999712),
 ( 0.9211408791463999712, 0.9211408791463999712, 0.9211408791463999712, 0.9211408791463999712, 0.9211408791463999712, 0.9211408791463999712, 0.9211408791463999712, 0.9211408791463999712, 0.9211408791463999712, 0.9211408791463999712, 0.9211408791463999712, 0.9211408791463999712, 0.9211408791463999712, 0.9211408791463999712, 0.9211408791463999712, 0.9211408791463999712, 0.9211408791463999712, 0.9211408791463999712, 0.9211408791463999712, 0.9211408791463999712, 0.9211408791463999712, 0.9211408791463999712, 0.9211408791463999712, 0.9211408791463999712, 0.9211408791463999712, 0.9211408791463999712, 0.9211408791463999712, 0.9211408791463999712, 0.9211408791463999712, 0.9211408791463999712, 0.9211408791463999712, 0.9211408791463999712, 0.9211408791463999712, 0.9211408791463999712, 0.9211408791463999712, 0.9211408791463999712, 0.9211408791463999712, 0.9211408791463999712, 0.9211408791463999712, 0.9211408791463999712, 0.9211408791463999712),
 ( 1.236577362560999926, 1.236577362560999926, 1.236577362560999926, 1.236577362560999926, 1.236577362560999926, 1.236577362560999926, 1.236577362560999926, 1.236577362560999926, 1.236577362560999926, 1.236577362560999926, 1.236577362560999926, 1.236577362560999926, 1.236577362560999926, 1.236577362560999926, 1.236577362560999926, 1.236577362560999926, 1.236577362560999926, 1.236577362560999926, 1.236577362560999926, 1.236577362560999926, 1.236577362560999926, 1.236577362560999926, 1.236577362560999926, 1.236577362560999926, 1.236577362560999926, 1.236577362560999926, 1.236577362560999926, 1.236577362560999926, 1.236577362560999926, 1.236577362560999926, 1.236577362560999926, 1.236577362560999926, 1.236577362560999926, 1.236577362560999926, 1.236577362560999926, 1.236577362560999926, 1.236577362560999926, 1.236577362560999926, 1.236577362560999926, 1.236577362560999926, 1.236577362560999926) ) ) 
 REPRESENTATION_ITEM ( '' )  SURFACE ( )  );
#4004=CARTESIAN_POINT ( 'NONE',  ( -14.21175436428723771, -5.188485551603381651, 315.0000000000000000 ) ) ;
#4005=CARTESIAN_POINT ( 'NONE',  ( 15.69672544750998888, -7.226176219113002119, -302.4229045757450081 ) ) ;
#4009=( NAMED_UNIT ( * ) PLANE_ANGLE_UNIT ( ) SI_UNIT ( $, .RADIAN. ) );
#4010=CARTESIAN_POINT ( 'NONE',  ( 19.95002954278003315, 1.762942793154997911, -302.9207377450070453 ) ) ;
#4012=VERTEX_POINT ( 'NONE', #3627 ) ;
#4013=CARTESIAN_POINT ( 'NONE',  ( -15.89383674730000173, -3.622219875512000087, -314.8616023057000461 ) ) ;
#4016=CARTESIAN_POINT ( 'NONE',  ( -13.71790339694999439, -8.616951602761004025, 189.9229057364800042 ) ) ;
#4017=CARTESIAN_POINT ( 'NONE',  ( 8.835721849737728562, 11.22420793802478123, 190.9999999999996589 ) ) ;
#4022=CARTESIAN_POINT ( 'NONE',  ( -3.874983216044999956, -9.425407904674999671, 314.8616023057000461 ) ) ;
#4024=CARTESIAN_POINT ( 'NONE',  ( 9.820740202793000861, 9.834836518498999425, 320.0000000000000000 ) ) ;
#4026=CARTESIAN_POINT ( 'NONE',  ( -15.56166711177641560, 7.864757419948934292, 319.0000000000005116 ) ) ;
#4030=CARTESIAN_POINT ( 'NONE',  ( -20.00000000000000000, -4.642018570833219964E-09, -316.5000000000000000 ) ) ;
#4036=ADVANCED_FACE ( 'NONE', ( #4528 ), #1307, .T. ) ;
#4037=CARTESIAN_POINT ( 'NONE',  ( 12.45718924559404250, 6.445992642206118006, 315.0000000000000568 ) ) ;
#4039=CARTESIAN_POINT ( 'NONE',  ( -19.99999035944999903, 7.277427703818000446E-10, -303.5000000000000000 ) ) ;
#4040=EDGE_CURVE ( 'NONE', #22, #9921, #9279, .T. ) ;
#4041=CARTESIAN_POINT ( 'NONE',  ( 16.90887668763000207, -0.2823175147257999673, -315.0848619657999734 ) ) ;
#4044=CARTESIAN_POINT ( 'NONE',  ( 17.04162109443001683, 6.546751591322998109, 318.8802828394900644 ) ) ;
#4047=EDGE_LOOP ( 'NONE', ( #9778, #577, #9554, #9446, #4375 ) ) ;
#4048=CARTESIAN_POINT ( 'NONE',  ( 20.01656911870001920, 0.3693805509907998053, -316.3802825947000201 ) ) ;
#4051=CARTESIAN_POINT ( 'NONE',  ( -14.26294315260000012, -7.573769859179999564, 320.0000000000000000 ) ) ;
#4055=CARTESIAN_POINT ( 'NONE',  ( -17.21226690345150701, 1.804990710747427007, -314.5172708043663192 ) ) ;
#4056=ORIENTED_EDGE ( 'NONE', *, *, #2343, .T. ) ;
#4057=CARTESIAN_POINT ( 'NONE',  ( 8.037373804805000077, 9.179324345868998591, -315.0000000000001137 ) ) ;
#4059=CARTESIAN_POINT ( 'NONE',  ( -8.094664229193854865, 11.44201740537352663, -316.5000000000004547 ) ) ;
#4061=CARTESIAN_POINT ( 'NONE',  ( 9.252434838928003558, -11.08696499602999630, -303.6197174156509391 ) ) ;
#4065=CARTESIAN_POINT ( 'NONE',  ( 20.05662131630997536, -0.5622531596958006972, -302.9207377450070453 ) ) ;
#4067=VERTEX_POINT ( 'NONE', #7015 ) ;
#4068=CARTESIAN_POINT ( 'NONE',  ( -17.42228208267999889, -1.444224815522999972, -314.4150829855000211 ) ) ;
#4069=CARTESIAN_POINT ( 'NONE',  ( -17.34693632642999717, -0.4167404706239999923, 314.6383426456000052 ) ) ;
#4071=CARTESIAN_POINT ( 'NONE',  ( -18.87182479219000442, 0.3569112016842001522, 190.0071920248299477 ) ) ;
#4073=CARTESIAN_POINT ( 'NONE',  ( 16.25556775813545940, 2.760696635281385092, -314.9999999999999432 ) ) ;
#4075=CARTESIAN_POINT ( 'NONE',  ( -11.89238025184999792, -6.701939844102000166, 315.0848619657999734 ) ) ;
#4077=CARTESIAN_POINT ( 'NONE',  ( 18.53598399141000286, 2.541378258162000137, 320.0000000000000000 ) ) ;
#4080=CARTESIAN_POINT ( 'NONE',  ( -12.96318846091385346, 9.529552999724863582, 319.0000000000005116 ) ) ;
#4084=CARTESIAN_POINT ( 'NONE',  ( -14.79012398733999945, 1.483731117707000058, -285.0000000000000000 ) ) ;
#4089=CARTESIAN_POINT ( 'NONE',  ( 13.98386538276810498, 5.376986245914816109, 315.0000000000000568 ) ) ;
#4090=CARTESIAN_POINT ( 'NONE',  ( 12.98706127646999953, 6.788989183774999603, -315.0000000000000000 ) ) ;
#4097=CARTESIAN_POINT ( 'NONE',  ( -3.772811979575000141, 12.36790329786001763, -317.0792622552969533 ) ) ;
#4100=PLANE ( 'NONE',  #2371 ) ;
#4103=FACE_OUTER_BOUND ( 'NONE', #80, .T. ) ;
#4104=CARTESIAN_POINT ( 'NONE',  ( 16.24410010525431503, -2.791089382272744501, -315.0000000000000568 ) ) ;
#4106=CARTESIAN_POINT ( 'NONE',  ( 17.50000000000125056, 1.338989683019597976E-14, -314.4963898845653034 ) ) ;
#4108=CARTESIAN_POINT ( 'NONE',  ( 7.617198281494000689, 10.53565010756000042, -317.5000000000000000 ) ) ;
#4113=EDGE_CURVE ( 'NONE', #4804, #9921, #666, .T. ) ;
#4116=CARTESIAN_POINT ( 'NONE',  ( 13.57573464316000056, -3.225916527208000151, 315.0000000000000000 ) ) ;
#4118=CARTESIAN_POINT ( 'NONE',  ( 14.92452513360000310, 8.330674305060012941, -303.6197174156509391 ) ) ;
#4121=CARTESIAN_POINT ( 'NONE',  ( -17.34089965840999881, -0.6440164457022999889, -314.6383426456000052 ) ) ;
#4125=CARTESIAN_POINT ( 'NONE',  ( 14.87873868498998498, -8.458320990069003287, 190.4207385301700128 ) ) ;
#4126=CARTESIAN_POINT ( 'NONE',  ( -17.50000000000107292, -0.7437989020622546299, -315.0000000000001137 ) ) ;
#4127=CARTESIAN_POINT ( 'NONE',  ( 13.67659370612792280, 5.618803873927791237, -315.0000000000000000 ) ) ;
#4131=CARTESIAN_POINT ( 'NONE',  ( 6.488017178959999853, -9.182784307579000327, 314.6383426456000052 ) ) ;
#4132=CARTESIAN_POINT ( 'NONE',  ( 16.69571944143998365, -6.308604365468005071, 320.0770942683900557 ) ) ;
#4134=CARTESIAN_POINT ( 'NONE',  ( 17.13182678275000370, -0.2945984483948000388, 314.8616023057000461 ) ) ;
#4136=ORIENTED_EDGE ( 'NONE', *, *, #3365, .F. ) ;
#4137=CARTESIAN_POINT ( 'NONE',  ( 18.18198898035900157, -5.227591177500494624, 190.9999999999995737 ) ) ;
#4139=ORIENTED_EDGE ( 'NONE', *, *, #2343, .F. ) ;
#4145=CARTESIAN_POINT ( 'NONE',  ( -2.001531325394999783, -11.45199047667999892, -302.5000000000000000 ) ) ;
#4146=LINE ( 'NONE', #10537, #3509 ) ;
#4150=CARTESIAN_POINT ( 'NONE',  ( 14.79012398733999767, 1.483731117707002278, -284.9999999999999432 ) ) ;
#4151=ORIENTED_EDGE ( 'NONE', *, *, #5879, .F. ) ;
#4152=CARTESIAN_POINT ( 'NONE',  ( -19.97263891460998764, -0.5563097477957001935, -316.3802825947000201 ) ) ;
#4154=CARTESIAN_POINT ( 'NONE',  ( 0.6600210488075000104, -11.51366633668999917, 320.0000000000000000 ) ) ;
#4158=CARTESIAN_POINT ( 'NONE',  ( 2.545630254023275807, -9.391959925330706227, -314.9999999999999432 ) ) ;
#4160=CARTESIAN_POINT ( 'NONE',  ( 17.42734739651272946, -0.9144542625322006346, -314.5039539236788642 ) ) ;
#4164=CARTESIAN_POINT ( 'NONE',  ( -18.53523119387001117, -4.742105934366003694, -303.6197174156509391 ) ) ;
#4166=CARTESIAN_POINT ( 'NONE',  ( -16.06911929583999310, -5.954958506906000260, -317.4928077629770087 ) ) ;
#4170=CARTESIAN_POINT ( 'NONE',  ( -13.93620031452002728, 8.972937827676991773, -303.6197174156509391 ) ) ;
#4177=ORIENTED_EDGE ( 'NONE', *, *, #4224, .F. ) ;
#4178=CARTESIAN_POINT ( 'NONE',  ( -0.7143903809592004883, -12.58977731883000750, 190.4207385301700128 ) ) ;
#4182=CARTESIAN_POINT ( 'NONE',  ( 0.7143903809590995690, 12.58977731883000750, 190.4207385301700128 ) ) ;
#4184=CARTESIAN_POINT ( 'NONE',  ( 17.34500932694999875, -0.6070218422356999932, 314.6383426456000052 ) ) ;
#4187=CARTESIAN_POINT ( 'NONE',  ( 19.56036991370999800, 0.5261966905397996719, 320.0770942683900557 ) ) ;
#4189=CARTESIAN_POINT ( 'NONE',  ( 5.255569329967310743, 12.07344867603089611, -303.5000000000000000 ) ) ;
#4190=CARTESIAN_POINT ( 'NONE',  ( 14.23799507159000122, 5.083276007328000112, 315.0848619657999734 ) ) ;
#4194=ORIENTED_EDGE ( 'NONE', *, *, #4113, .F. ) ;
#4198=CARTESIAN_POINT ( 'NONE',  ( -11.65165375873240450, 6.897932327036405020, 315.0000000000000568 ) ) ;
#4199=CARTESIAN_POINT ( 'NONE',  ( 7.006889269069000115, -6.844138725329000472, -285.0000000000000000 ) ) ;
#4207=CARTESIAN_POINT ( 'NONE',  ( 15.00000000000071587, 0.4945770392355663403, -284.9999999999999432 ) ) ;
#4208=CARTESIAN_POINT ( 'NONE',  ( 17.49999999954662044, -9.625715914672042649E-06, 190.0000000000000000 ) ) ;
#4209=CARTESIAN_POINT ( 'NONE',  ( 3.356563794682998925, 12.33103673683000423, -316.3802825947000201 ) ) ;
#4213=CARTESIAN_POINT ( 'NONE',  ( 8.673912564134326431, -8.158689640371338925, -315.0000000000000000 ) ) ;
#4215=CARTESIAN_POINT ( 'NONE',  ( -4.557748955467412877, -9.652551271539406841, -314.5171779026347281 ) ) ;
#4219=CARTESIAN_POINT ( 'NONE',  ( -10.53744240725999681, -10.62869657088999986, -303.6197174156509391 ) ) ;
#4220=CARTESIAN_POINT ( 'NONE',  ( -1.546121016139999638, -11.35842264293001591, -317.4928077629770087 ) ) ;
#4223=( GEOMETRIC_REPRESENTATION_CONTEXT ( 3 ) GLOBAL_UNCERTAINTY_ASSIGNED_CONTEXT ( ( #5061 ) ) GLOBAL_UNIT_ASSIGNED_CONTEXT ( ( #9060, #9759, #1596 ) ) REPRESENTATION_CONTEXT ( 'NONE', 'WORKASPACE' ) );
#4224=EDGE_CURVE ( 'NONE', #7676, #245, #3617, .T. ) ;
#4225=CARTESIAN_POINT ( 'NONE',  ( 6.686361683900003072, 11.78513185998999546, -303.6197174156509391 ) ) ;
#4226=CARTESIAN_POINT ( 'NONE',  ( 19.99998650234378417, -8.894530540522598959E-07, -302.9142199863263158 ) ) ;
#4228=CARTESIAN_POINT ( 'NONE',  ( -16.75097866579000083, -2.074182492207000461, -314.8616023057000461 ) ) ;
#4230=ORIENTED_EDGE ( 'NONE', *, *, #7181, .T. ) ;
#4231=CARTESIAN_POINT ( 'NONE',  ( 15.66663193639001506, -7.880331994043005217, 190.4207385301700128 ) ) ;
#4232=CARTESIAN_POINT ( 'NONE',  ( -12.98706127646999953, -6.788989183774999603, -314.4944826805095772 ) ) ;
#4233=CARTESIAN_POINT ( 'NONE',  ( 13.37774034208871399, 5.841704189632139332, -314.9999999999999432 ) ) ;
#4235=CARTESIAN_POINT ( 'NONE',  ( 15.65104815535000071, 7.893060908445997725, 190.4207385301700128 ) ) ;
#4236=CARTESIAN_POINT ( 'NONE',  ( -18.86318716375000193, 0.4770217013004998119, 319.9928079742500131 ) ) ;
#4237=EDGE_CURVE ( 'NONE', #563, #6747, #5859, .T. ) ;
#4238=EDGE_CURVE ( 'NONE', #1396, #4540, #1556, .T. ) ;
#4239=CARTESIAN_POINT ( 'NONE',  ( 17.13090252310000139, 0.3058267005333999977, 314.8616023057000461 ) ) ;
#4241=CARTESIAN_POINT ( 'NONE',  ( -6.386114867952997542, -11.42839325896998481, 320.0770942683900557 ) ) ;
#4242=CARTESIAN_POINT ( 'NONE',  ( -14.91207365418872044, 5.270756744682541850, 314.4999413757458342 ) ) ;
#4243=CARTESIAN_POINT ( 'NONE',  ( 16.39086977655999888, 2.839079766962000040, 314.8616023057000461 ) ) ;
#4245=CARTESIAN_POINT ( 'NONE',  ( -13.01454326516111237, -9.502166178128929275, 190.9999999999995737 ) ) ;
#4247=CARTESIAN_POINT ( 'NONE',  ( 20.04731132535002303, 0.9079451813825001327, 319.5792614743400009 ) ) ;
#4252=CARTESIAN_POINT ( 'NONE',  ( -11.74237836840727311, 6.849546447955716211, 315.0000000000000000 ) ) ;
#4254=CARTESIAN_POINT ( 'NONE',  ( -7.006889269069000115, -6.844138725329000472, -285.0000000000000000 ) ) ;
#4255=ORIENTED_EDGE ( 'NONE', *, *, #5245, .F. ) ;
#4256=CARTESIAN_POINT ( 'NONE',  ( 6.328188536734999481, -10.84734154703999920, -302.5000000000000000 ) ) ;
#4260=CARTESIAN_POINT ( 'NONE',  ( 17.22665784523203669, -1.821305572729455813, 314.4999396030180492 ) ) ;
#4262=CARTESIAN_POINT ( 'NONE',  ( 2.381287040813000348E-07, -10.00000001404999850, 190.0000000000000000 ) ) ;
#4267=CARTESIAN_POINT ( 'NONE',  ( -18.99999441908000009, -1.671652456891999947E-07, 319.0000000000000000 ) ) ;
#4268=CARTESIAN_POINT ( 'NONE',  ( -2.157987297531679616, -9.422522223986293355, -314.9999999999999432 ) ) ;
#4269=ORIENTED_EDGE ( 'NONE', *, *, #3388, .T. ) ;
#4270=CARTESIAN_POINT ( 'NONE',  ( 11.51453371961018490, -7.479120141997832150, -314.5676927934670175 ) ) ;
#4272=ORIENTED_EDGE ( 'NONE', *, *, #8378, .F. ) ;
#4273=CARTESIAN_POINT ( 'NONE',  ( -11.32071836301000012, 9.223563301002998926, -317.5000000000000000 ) ) ;
#4275=CARTESIAN_POINT ( 'NONE',  ( -14.92452513360000310, -8.330674305060012941, -303.6197174156509391 ) ) ;
#4276=CARTESIAN_POINT ( 'NONE',  ( 7.982667963825995194, -11.03627960042998701, -317.5770954168139610 ) ) ;
#4278=CARTESIAN_POINT ( 'NONE',  ( -16.55686070535999832, 1.955716293870999767, -315.0848619657999734 ) ) ;
#4280=CARTESIAN_POINT ( 'NONE',  ( -1.673754838359998498, 12.46646309164999522, -303.6197174156520759 ) ) ;
#4283=CARTESIAN_POINT ( 'NONE',  ( -16.90887668763000207, 0.2823175147257999673, -315.0848619657999734 ) ) ;
#4284=CARTESIAN_POINT ( 'NONE',  ( -8.922355960362999383, 10.14988298126000110, -302.5000000000000000 ) ) ;
#4286=CARTESIAN_POINT ( 'NONE',  ( 12.19509678855998835, -10.00267306739999640, 190.4207385301700128 ) ) ;
#4288=CARTESIAN_POINT ( 'NONE',  ( 12.75178873474798991, 6.273979344207472941, -315.0000000000000000 ) ) ;
#4289=CARTESIAN_POINT ( 'NONE',  ( 17.70739197152998656, 5.947706840970997888, 190.4207385301700128 ) ) ;
#4291=CARTESIAN_POINT ( 'NONE',  ( 16.28527389671999970, -3.844447514156999812, 314.4150829855000211 ) ) ;
#4294=CARTESIAN_POINT ( 'NONE',  ( -8.948397653779995409, -10.74758637870000477, 320.0770942683900557 ) ) ;
#4295=CARTESIAN_POINT ( 'NONE',  ( -13.64750600793954227, 6.290789886748213711, 314.4999418822394546 ) ) ;
#4296=( LENGTH_UNIT ( ) NAMED_UNIT ( * ) SI_UNIT ( .MILLI., .METRE. ) );
#4297=CARTESIAN_POINT ( 'NONE',  ( 14.67553856548000013, 5.592168771406000438, 314.4150829855000211 ) ) ;
#4299=CARTESIAN_POINT ( 'NONE',  ( 19.99997381626590709, -0.3203551279404398544, 190.9999999999995737 ) ) ;
#4300=CARTESIAN_POINT ( 'NONE',  ( 19.97284365803998796, -0.5561741493802002667, 318.8802828394900644 ) ) ;
#4304=CARTESIAN_POINT ( 'NONE',  ( -6.369677570987301252, 8.818560138237836910, 315.0000000000000000 ) ) ;
#4306=ORIENTED_EDGE ( 'NONE', *, *, #5162, .T. ) ;
#4310=CARTESIAN_POINT ( 'NONE',  ( -16.68824139745838409, 1.819223930145250856, -315.0000000000000000 ) ) ;
#4320=CARTESIAN_POINT ( 'NONE',  ( 13.98368610735813888, -5.377133503752140165, -315.0000000000000568 ) ) ;
#4321=EDGE_LOOP ( 'NONE', ( #6540, #7792, #8836, #8997 ) ) ;
#4323=CARTESIAN_POINT ( 'NONE',  ( -14.93376631645305253, -8.332910267862528642, -316.5000000000004547 ) ) ;
#4328=CARTESIAN_POINT ( 'NONE',  ( 6.660995095996002924, -11.36691212455000333, -317.5770954168139610 ) ) ;
#4329=CARTESIAN_POINT ( 'NONE',  ( -17.57673583306999632, -0.3313182897943000582, -314.4150829855000211 ) ) ;
#4330=CARTESIAN_POINT ( 'NONE',  ( -20.01694242003000568, 0.3416920405409001327, -303.6197174156520759 ) ) ;
#4331=CARTESIAN_POINT ( 'NONE',  ( 10.32803372116435270, 10.00000000000000178, 314.4999507458385324 ) ) ;
#4333=CARTESIAN_POINT ( 'NONE',  ( 8.751711036432999080, -10.20177972100999853, 190.0000000000000000 ) ) ;
#4334=CARTESIAN_POINT ( 'NONE',  ( -15.28688047792000049, 6.812924772642000804, -302.5000000000000000 ) ) ;
#4337=CARTESIAN_POINT ( 'NONE',  ( 18.24410766404003326, -5.273389473771006308, 190.4207385301700128 ) ) ;
#4339=CARTESIAN_POINT ( 'NONE',  ( -3.563286991701002382, -11.18699815210999660, -302.5071922382879279 ) ) ;
#4340=CARTESIAN_POINT ( 'NONE',  ( -17.00602911426001285, 6.582783228486000837, 191.1197171614399792 ) ) ;
#4342=CARTESIAN_POINT ( 'NONE',  ( 8.690073206612000334, -8.569658446474999636, 314.6383426456000052 ) ) ;
#4345=VECTOR ( 'NONE', #2416, 1000.000000000000000 ) ;
#4346=CARTESIAN_POINT ( 'NONE',  ( 18.89077695122000122, -0.08689258194099000465, 319.9928079742500131 ) ) ;
#4347=CARTESIAN_POINT ( 'NONE',  ( -6.176507045891521663, 9.366274624700933416, 314.4999436549672964 ) ) ;
#4348=CARTESIAN_POINT ( 'NONE',  ( 10.54003729909880960, 10.63540770771157717, -303.5000000000000000 ) ) ;
#4349=CARTESIAN_POINT ( 'NONE',  ( 3.903842856253999738, 9.647088721075000706, 314.6383426456000052 ) ) ;
#4351=CARTESIAN_POINT ( 'NONE',  ( 19.95972666420564323, -0.9723020053077987557, 190.9999999999995737 ) ) ;
#4352=CARTESIAN_POINT ( 'NONE',  ( 14.92426358056000701, 8.426786174986000688, 319.5792614743400009 ) ) ;
#4355=CARTESIAN_POINT ( 'NONE',  ( -4.298491262593391760, 9.188587546143761386, 314.9999999999999432 ) ) ;
#4356=FACE_OUTER_BOUND ( 'NONE', #9247, .T. ) ;
#4362=CARTESIAN_POINT ( 'NONE',  ( -4.792833739245000224, 11.13811509850999926, 190.0000000000000000 ) ) ;
#4363=CARTESIAN_POINT ( 'NONE',  ( -14.08970834377950787, 5.290460773273633954, -314.9999999999999432 ) ) ;
#4364=CARTESIAN_POINT ( 'NONE',  ( 18.85519295008999663, 0.7686777388422003643, 190.0071920248299477 ) ) ;
#4373=CARTESIAN_POINT ( 'NONE',  ( -0.6117794464027001000, 11.39410369034999704, 319.9928079742500131 ) ) ;
#4375=ORIENTED_EDGE ( 'NONE', *, *, #10494, .F. ) ;
#4380=CARTESIAN_POINT ( 'NONE',  ( -18.86306334786000605, -0.4771235332117997885, -317.4928077629770087 ) ) ;
#4381=CARTESIAN_POINT ( 'NONE',  ( -8.850998676319990821, -10.04707221382999194, -317.4928077629770087 ) ) ;
#4384=CARTESIAN_POINT ( 'NONE',  ( 17.20152651095803975, 1.793788947124328681, -314.5180462286796796 ) ) ;
#4385=CARTESIAN_POINT ( 'NONE',  ( -7.551285642361038164, -9.031218629016434463, 314.4999459341803458 ) ) ;
#4386=VERTEX_POINT ( 'NONE', #9189 ) ;
#4387=CARTESIAN_POINT ( 'NONE',  ( 18.20429351259000228, -3.291556992836000006, 190.0000000000000000 ) ) ;
#4390=CARTESIAN_POINT ( 'NONE',  ( -7.559362580479000115, -11.57734716366000072, 191.1197171614399792 ) ) ;
#4393=CARTESIAN_POINT ( 'NONE',  ( -10.13603924037000326, -9.590552501249007378, -302.5071922382879279 ) ) ;
#4394=CARTESIAN_POINT ( 'NONE',  ( 17.08426003144000305, 6.624354047749995367, 190.4207385301700128 ) ) ;
#4397=CARTESIAN_POINT ( 'NONE',  ( -14.33246323392999422, 7.385748264902002092, -302.5071922382879279 ) ) ;
#4398=CARTESIAN_POINT ( 'NONE',  ( 6.055260875802999543, -12.00648505189998971, 319.5792614743400009 ) ) ;
#4399=CARTESIAN_POINT ( 'NONE',  ( 14.57772014836000096, -5.380605385836000565, -314.6383426456000052 ) ) ;
#4400=CARTESIAN_POINT ( 'NONE',  ( -1.409290114754000012, 9.868237606049000021, 314.6383426456000052 ) ) ;
#4402=CARTESIAN_POINT ( 'NONE',  ( 14.93050028969001808, -6.935770771621001529, 190.0071920248299477 ) ) ;
#4404=CARTESIAN_POINT ( 'NONE',  ( -12.99935040274999487, 9.597679858163006728, 319.5792614743400009 ) ) ;
#4407=CARTESIAN_POINT ( 'NONE',  ( 1.573733331195987573, 9.469132543440894167, 315.0000000000001137 ) ) ;
#4408=CARTESIAN_POINT ( 'NONE',  ( 0.000000000000000000, -7.937240849781000307, -284.9999999999999432 ) ) ;
#4411=CARTESIAN_POINT ( 'NONE',  ( 1.604652481465360658, -9.999950686259090560, 314.4999444147077838 ) ) ;
#4413=CARTESIAN_POINT ( 'NONE',  ( -17.73236801841998300, 3.892024484092002634, 190.0071920248299477 ) ) ;
#4421=CARTESIAN_POINT ( 'NONE',  ( 18.14104367554000774, 3.149620910056999623, 319.9928079742500131 ) ) ;
#4422=CARTESIAN_POINT ( 'NONE',  ( -9.195128512800469167, -11.11313767369120775, -316.5000000000004547 ) ) ;
#4423=CARTESIAN_POINT ( 'NONE',  ( 0.000000000000000000, 0.000000000000000000, 320.0000000000000000 ) ) ;
#4425=CARTESIAN_POINT ( 'NONE',  ( -9.022589772749004311, 9.990182113135000819, -317.4928077629770087 ) ) ;
#4426=CARTESIAN_POINT ( 'NONE',  ( 15.01674827698000314, -8.369013993811000418, -317.0792622552969533 ) ) ;
#4430=CARTESIAN_POINT ( 'NONE',  ( 17.50000000000000000, 0.000000000000000000, -314.4999343908002629 ) ) ;
#4431=B_SPLINE_SURFACE_WITH_KNOTS ( 'NONE', 3, 3, ( 
 ( #1503, #3545, #1769, #8322 ),
 ( #3326, #4134, #7622, #7464 ),
 ( #5040, #9298, #2736, #957 ),
 ( #6606, #2523, #7411, #9079 ),
 ( #1826, #6771, #8373, #1929 ),
 ( #10096, #3385, #268, #8423 ),
 ( #6661, #4243, #5091, #5956 ),
 ( #53, #9886, #7515, #6825 ),
 ( #6003, #10045, #1009, #9191 ),
 ( #4190, #159, #5147, #4297 ),
 ( #8213, #3433, #7569, #3492 ),
 ( #5788, #851, #214, #2688 ),
 ( #6712, #9990, #2632, #1716 ),
 ( #4988, #107, #8265, #5895 ),
 ( #904, #9246, #9936, #2574 ),
 ( #1876, #1063, #4349, #5842 ),
 ( #9133, #8623, #1118, #3694 ),
 ( #2991, #6876, #4400, #8572 ),
 ( #6981, #7771, #3643, #5298 ),
 ( #1216, #4494, #6210, #4447 ),
 ( #9346, #9495, #6267, #3593 ),
 ( #9445, #4549, #5200, #5250 ),
 ( #7823, #7087, #415, #1270 ),
 ( #10143, #2135, #1169, #470 ),
 ( #7675, #367, #319, #2786 ),
 ( #7726, #6926, #5402, #8680 ),
 ( #6057, #8473, #10199, #1321 ),
 ( #4604, #3742, #1983, #8524 ),
 ( #2841, #6109, #2031, #7878 ),
 ( #7031, #9546, #10252, #9396 ),
 ( #2888, #6157, #2083, #10303 ),
 ( #5347, #525, #2939, #3798 ),
 ( #10353, #632, #6429, #738 ),
 ( #3261, #8152, #4069, #7994 ) ),
 .UNSPECIFIED., .F., .F., .F.,
 ( 4, 1, 1, 1, 1, 1, 1, 1, 1, 1, 1, 1, 1, 1, 1, 1, 1, 1, 1, 1, 1, 1, 1, 1, 1, 1, 1, 1, 1, 1, 1, 4 ),
 ( 4, 4 ),
 ( -0.01574130609828000224, 0.000000000000000000, 0.03448275862069000164, 0.06896551724138000328, 0.1034482758621000087, 0.1379310344828000023, 0.1724137931033999926, 0.2068965517240999863, 0.2413793103448000077, 0.2758620689655000291, 0.3103448275861999672, 0.3448275862069000164, 0.3793103448276000100, 0.4137931034483000037, 0.4482758620689999973, 0.4827586206897000465, 0.5172413793103000090, 0.5517241379310000582, 0.5862068965516999963, 0.6206896551723999345, 0.6551724137930999836, 0.6896551724138000328, 0.7241379310344999709, 0.7586206896552000201, 0.7931034482758999582, 0.8275862068966000074, 0.8620689655171999144, 0.8965517241379000746, 0.9310344827586000127, 0.9655172413793000619, 1.000000000000000000, 1.014026462982999810 ),
 ( -0.1697239316932999953, 1.169834029081999960 ),
 .UNSPECIFIED. ) ;
#4433=CARTESIAN_POINT ( 'NONE',  ( -18.78940217795999956, -1.754852253524999961, 190.0000000000000000 ) ) ;
#4437=CARTESIAN_POINT ( 'NONE',  ( -6.108404012864005139, -11.90988283206001519, 191.1197171614399792 ) ) ;
#4443=EDGE_CURVE ( 'NONE', #189, #8110, #8867, .T. ) ;
#4444=CARTESIAN_POINT ( 'NONE',  ( 16.85751871341000907, 5.113642021703998175, -302.5071922382879279 ) ) ;
#4445=CARTESIAN_POINT ( 'NONE',  ( -7.868470208275999411, -11.58296045169998401, 319.5792614743400009 ) ) ;
#4447=CARTESIAN_POINT ( 'NONE',  ( -6.537559671572000575, 9.400791339334000796, 314.4150829855000211 ) ) ;
#4449=CARTESIAN_POINT ( 'NONE',  ( -17.02940347669787613, -6.570098831661550953, 190.9999999999995737 ) ) ;
#4450=CARTESIAN_POINT ( 'NONE',  ( -4.392607225559004291, 12.20457772578000366, 318.8802828394900644 ) ) ;
#4451=AXIS2_PLACEMENT_3D ( 'NONE', #6520, #2279, #4859 ) ;
#4454=CARTESIAN_POINT ( 'NONE',  ( -13.94549574055089458, 5.407931305651876741, 315.0000000000001137 ) ) ;
#4460=CARTESIAN_POINT ( 'NONE',  ( -15.46045765806406891, 3.925441769934806757, -315.0000000000000568 ) ) ;
#4463=CARTESIAN_POINT ( 'NONE',  ( 0.2188334844704999949, -11.51755598686999882, -317.5000000000000000 ) ) ;
#4465=CARTESIAN_POINT ( 'NONE',  ( 15.44313366109816599, -3.946504251847836819, 315.0000000000000568 ) ) ;
#4466=CARTESIAN_POINT ( 'NONE',  ( 10.50000150490000017, 7.882579085736000302, -314.6383426456000052 ) ) ;
#4467=VERTEX_POINT ( 'NONE', #2554 ) ;
#4468=CARTESIAN_POINT ( 'NONE',  ( -12.43797004353999469, 8.540074035031999244, 319.9928079742500131 ) ) ;
#4469=CARTESIAN_POINT ( 'NONE',  ( -7.865580335751168661, -11.50505378538359125, -316.5000000000004547 ) ) ;
#4472=CARTESIAN_POINT ( 'NONE',  ( 8.850998676319990821, 10.04707221382999194, -317.4928077629770087 ) ) ;
#4473=CARTESIAN_POINT ( 'NONE',  ( -19.57077664853002119, 0.3812814288523002082, -317.5770954168139610 ) ) ;
#4475=CARTESIAN_POINT ( 'NONE',  ( 16.39561153668567428, 3.420321068896136296, -314.5539561507842450 ) ) ;
#4477=CARTESIAN_POINT ( 'NONE',  ( -18.99997815069999874, -0.3119984768183999835, 190.0000000000100044 ) ) ;
#4490=CARTESIAN_POINT ( 'NONE',  ( -10.11757849520999031, 9.598459870364994373, -302.5071922382879279 ) ) ;
#4491=CARTESIAN_POINT ( 'NONE',  ( -20.04731132535002303, -0.9079451813825001327, 319.5792614743400009 ) ) ;
#4494=CARTESIAN_POINT ( 'NONE',  ( -6.438474686349000997, 8.964777275824999947, 314.8616023057000461 ) ) ;
#4496=CARTESIAN_POINT ( 'NONE',  ( -5.890130794754004029, -10.81842929378999330, 190.0071920248299477 ) ) ;
#4503=CARTESIAN_POINT ( 'NONE',  ( 19.00000000000000000, 0.000000000000000000, 319.9999999999899956 ) ) ;
#4505=CARTESIAN_POINT ( 'NONE',  ( -8.586696445213114259, -8.187646113561793726, -314.9999999999999432 ) ) ;
#4508=CARTESIAN_POINT ( 'NONE',  ( 20.00000000000000000, 7.322330471414334241, -316.5000000000000000 ) ) ;
#4509=CARTESIAN_POINT ( 'NONE',  ( 8.517086849895166623, 8.210518282650744126, -314.9999999999999432 ) ) ;
#4511=CARTESIAN_POINT ( 'NONE',  ( 16.99996037728000076, -1.352915083302999933E-09, -314.9999801883000146 ) ) ;
#4512=VERTEX_POINT ( 'NONE', #29 ) ;
#4513=CARTESIAN_POINT ( 'NONE',  ( -16.89340345063000015, -5.253727359668999952, -317.4999999999989768 ) ) ;
#4517=CARTESIAN_POINT ( 'NONE',  ( 15.88661950543927404, -3.373766516133892335, 315.0000000000000000 ) ) ;
#4518=CARTESIAN_POINT ( 'NONE',  ( 6.273744347102000241, 8.772995918477999311, -315.0848619657999734 ) ) ;
#4520=CARTESIAN_POINT ( 'NONE',  ( -17.50000000000000000, 1.896400240175167841E-08, 314.4999014931028682 ) ) ;
#4524=CARTESIAN_POINT ( 'NONE',  ( 14.29183324405000732, 7.414293696095001884, -317.4928077629770087 ) ) ;
#4525=CARTESIAN_POINT ( 'NONE',  ( -9.065820074235004356, -10.71255845790999572, -317.5770954168139610 ) ) ;
#4528=FACE_OUTER_BOUND ( 'NONE', #5896, .T. ) ;
#4532=CARTESIAN_POINT ( 'NONE',  ( 14.98664244983999971, -7.043920630080999778, 190.0000000000000000 ) ) ;
#4533=CARTESIAN_POINT ( 'NONE',  ( -17.04674817168135803, -6.551802883975634373, 319.0000000000003979 ) ) ;
#4535=CARTESIAN_POINT ( 'NONE',  ( -11.02833964697000013, -10.42949886550000826, 191.1197171614399792 ) ) ;
#4537=CARTESIAN_POINT ( 'NONE',  ( 17.50000000000000711, -8.653813013134384923E-10, -302.5000000000000568 ) ) ;
#4538=CARTESIAN_POINT ( 'NONE',  ( -18.86301435545000871, 0.4770680115090000228, -302.5071922382879279 ) ) ;
#4539=CARTESIAN_POINT ( 'NONE',  ( -16.99996037728000076, 1.352916535802999941E-09, -314.9999801883000146 ) ) ;
#4540=VERTEX_POINT ( 'NONE', #9114 ) ;
#4545=CARTESIAN_POINT ( 'NONE',  ( 11.24500836742999610, 9.126642939585995151, -302.5071922382879279 ) ) ;
#4547=CARTESIAN_POINT ( 'NONE',  ( -18.20466326549998470, -5.184475519960003886, 318.8802828394900644 ) ) ;
#4548=CARTESIAN_POINT ( 'NONE',  ( 16.77957632114000219, -1.244976636274000015, -315.0848619657999734 ) ) ;
#4549=CARTESIAN_POINT ( 'NONE',  ( -10.49789511286000021, 7.639556387670999982, 314.8616023057000461 ) ) ;
#4553=CARTESIAN_POINT ( 'NONE',  ( -9.912528015309003848, 10.85837313990000474, 318.8802828394900644 ) ) ;
#4558=CARTESIAN_POINT ( 'NONE',  ( 16.99965680672947954, -0.4176726732850533641, 314.9999999999998863 ) ) ;
#4559=CARTESIAN_POINT ( 'NONE',  ( -13.95695539824072640, 5.398716172439862682, 315.0000000000000568 ) ) ;
#4561=CARTESIAN_POINT ( 'NONE',  ( 14.99960151356000004, 7.033824075090999273, 320.0000000000000000 ) ) ;
#4562=CARTESIAN_POINT ( 'NONE',  ( -13.92525118639320070, -5.424153755683055245, -314.9999999999999432 ) ) ;
#4567=CARTESIAN_POINT ( 'NONE',  ( 3.309734165293447550, 9.320883339027414394, -315.0000000000000568 ) ) ;
#4568=CARTESIAN_POINT ( 'NONE',  ( -16.06649953495000105, 6.900914778667005756, 189.9229057364800042 ) ) ;
#4571=VERTEX_POINT ( 'NONE', #6530 ) ;
#4575=CARTESIAN_POINT ( 'NONE',  ( 16.80170962578117155, -1.436180489853609688, 315.0000000000000568 ) ) ;
#4576=CARTESIAN_POINT ( 'NONE',  ( -13.62823431091000081, 6.408810695481999886, -314.4150829855000211 ) ) ;
#4577=EDGE_CURVE ( 'NONE', #2473, #8913, #4780, .T. ) ;
#4578=CARTESIAN_POINT ( 'NONE',  ( -1.604641474886230768, -9.999988122786408695, 314.4999449211996989 ) ) ;
#4579=CARTESIAN_POINT ( 'NONE',  ( 8.948397653779995409, 10.74758637870000477, 320.0770942683900557 ) ) ;
#4581=ORIENTED_EDGE ( 'NONE', *, *, #7985, .F. ) ;
#4582=CARTESIAN_POINT ( 'NONE',  ( 1.581094244357999612, 12.05691037822999867, -317.5770954168139610 ) ) ;
#4583=CARTESIAN_POINT ( 'NONE',  ( 11.79032227421999757, -10.19419839316000065, -317.0792622552969533 ) ) ;
#4584=PRODUCT_DEFINITION_SHAPE ( 'NONE', 'NONE',  #2387 ) ;
#4589=CARTESIAN_POINT ( 'NONE',  ( -16.27944536538999998, 5.903984566639000064, 190.0000000000000000 ) ) ;
#4592=VERTEX_POINT ( 'NONE', #10503 ) ;
#4593=CARTESIAN_POINT ( 'NONE',  ( 12.15874467096999645, -9.926591843472005294, 191.1197171614399792 ) ) ;
#4596=CARTESIAN_POINT ( 'NONE',  ( 16.59121592455001348, -6.423372090527998068, -302.4229045757450081 ) ) ;
#4600=B_SPLINE_CURVE_WITH_KNOTS ( 'NONE', 3,
 ( #4511, #5364, #8752, #7789 ),
 .UNSPECIFIED., .F., .F.,
 ( 4, 4 ),
 ( 0.000000000000000000, 1.000000000000000000 ),
 .UNSPECIFIED. ) ;
#4601=CARTESIAN_POINT ( 'NONE',  ( -18.86312040460998674, -0.4763280864498002920, -302.5071922382879279 ) ) ;
#4602=CARTESIAN_POINT ( 'NONE',  ( 11.00353245304999739, -10.53087951318999593, 319.5792614743400009 ) ) ;
#4604=CARTESIAN_POINT ( 'NONE',  ( -16.21525914616999842, 2.693567875512000054, 315.0848619657999734 ) ) ;
#4611=CARTESIAN_POINT ( 'NONE',  ( -15.43580712988967107, 3.955371400427518669, 315.0000000000000568 ) ) ;
#4612=CARTESIAN_POINT ( 'NONE',  ( -17.49999996772987743, -5.857864456328762515, 314.9999999999999432 ) ) ;
#4613=CARTESIAN_POINT ( 'NONE',  ( -7.529234060647197246, -8.513083068079142279, -315.0000000000000000 ) ) ;
#4616=CARTESIAN_POINT ( 'NONE',  ( -3.713614856666575144E-09, 12.50000000000000000, -316.5000000000000000 ) ) ;
#4619=CARTESIAN_POINT ( 'NONE',  ( 8.647412455283767230, 8.167526177888579042, -315.0000000000000000 ) ) ;
#4621=CARTESIAN_POINT ( 'NONE',  ( 19.59059457349998823, 0.06993619660358003920, 189.9229057364800042 ) ) ;
#4622=CARTESIAN_POINT ( 'NONE',  ( 17.22664556582829931, 1.821222547514791623, 314.4999497328577718 ) ) ;
#4623=CARTESIAN_POINT ( 'NONE',  ( 18.87000901094000227, -1.611639242563999819, -317.5000000000470095 ) ) ;
#4628=CARTESIAN_POINT ( 'NONE',  ( 11.33727843270404634, -7.061073773682574384, 315.0000000000000000 ) ) ;
#4630=CARTESIAN_POINT ( 'NONE',  ( 10.32396869588999877, 7.471487098147999717, -315.0848619657999734 ) ) ;
#4632=CARTESIAN_POINT ( 'NONE',  ( 16.10430118153999857, 6.867346955731005842, 320.0770942683900557 ) ) ;
#4636=CARTESIAN_POINT ( 'NONE',  ( -9.242264416715993747, 10.65406548831999878, -317.5770954168139610 ) ) ;
#4638=CARTESIAN_POINT ( 'NONE',  ( -15.92039057294001125, -7.578271297757998681, -316.3802825947000201 ) ) ;
#4639=CARTESIAN_POINT ( 'NONE',  ( 15.67978886374999803, -4.575336738469999887, -315.0000000000000000 ) ) ;
#4644=CARTESIAN_POINT ( 'NONE',  ( -18.95640219669000004, 0.9217981998336000071, 190.0000000000000000 ) ) ;
#4645=CARTESIAN_POINT ( 'NONE',  ( 16.99398431597747461, -6.605820200493085714, 319.0000000000003979 ) ) ;
#4646=ORIENTED_EDGE ( 'NONE', *, *, #5584, .F. ) ;
#4648=ORIENTED_EDGE ( 'NONE', *, *, #9438, .F. ) ;
#4649=CARTESIAN_POINT ( 'NONE',  ( -13.12098914876195366, -6.031629431400056696, 314.9999999999999432 ) ) ;
#4650=CARTESIAN_POINT ( 'NONE',  ( -19.37583693248997108, -3.422417436021003123, -302.9207377450070453 ) ) ;
#4655=CARTESIAN_POINT ( 'NONE',  ( 15.97017057534000450, 7.646575558462997080, -302.9207377450070453 ) ) ;
#4659=CARTESIAN_POINT ( 'NONE',  ( -10.58801790939999954, -8.088125079530000150, -314.4150829855000211 ) ) ;
#4660=CARTESIAN_POINT ( 'NONE',  ( 18.32212638522000248, 3.124911926288000075, -302.5000000000129603 ) ) ;
#4662=CARTESIAN_POINT ( 'NONE',  ( 17.84297720825001221, -4.977647671642006166, 189.9229057364800042 ) ) ;
#4667=CARTESIAN_POINT ( 'NONE',  ( 4.001463906138999604, -9.408458373209999337, 314.8616023057000461 ) ) ;
#4668=CARTESIAN_POINT ( 'NONE',  ( 17.59656075795390606, 5.807225057570236437, 315.0000000000000000 ) ) ;
#4669=CARTESIAN_POINT ( 'NONE',  ( -15.06605725946605112, 4.378913172242680396, 314.9999999999999432 ) ) ;
#4670=CARTESIAN_POINT ( 'NONE',  ( -14.24138406224000342, -7.443131114976996976, 319.9928079742500131 ) ) ;
#4671=CARTESIAN_POINT ( 'NONE',  ( -11.33749276371199066, -7.060967193034008993, -315.0000000000000568 ) ) ;
#4675=DIRECTION ( 'NONE',  ( -1.000000000000000000, 0.000000000000000000, 0.000000000000000000 ) ) ;
#4676=CARTESIAN_POINT ( 'NONE',  ( -4.934865307815709201, 9.087242801873953724, -315.0000000000000568 ) ) ;
#4678=CARTESIAN_POINT ( 'NONE',  ( -18.32859070493001852, 4.258570244206002720, 189.9229057364800042 ) ) ;
#4680=CARTESIAN_POINT ( 'NONE',  ( -16.13706688435999581, -6.055114415286000806, -317.5000000000000000 ) ) ;
#4684=CARTESIAN_POINT ( 'NONE',  ( -12.98706127646999953, 6.788989183774999603, -315.0000000000000000 ) ) ;
#4685=CARTESIAN_POINT ( 'NONE',  ( 1.257430124576000008, 9.427442400486999219, -315.0848619657999734 ) ) ;
#4688=CARTESIAN_POINT ( 'NONE',  ( 20.06710154196001739, -0.4210530330733002757, 319.5792614743400009 ) ) ;
#4691=CARTESIAN_POINT ( 'NONE',  ( -12.90264537120001798, 9.651629027462002242, -317.0792622552969533 ) ) ;
#4692=( BOUNDED_CURVE ( )  B_SPLINE_CURVE ( 3, ( #1931, #4299, #4351, #8476, #9888, #3494, #10047, #4137, #7466, #2690, #5202, #6608, #7624, #1878, #270, #55, #2738, #161, #6827, #109, #5897, #3328, #959, #2525, #5790, #6663, #5844, #10098, #2577, #9135, #1771, #5042, #8324, #4245, #6715, #5093, #7880, #10145, #4449, #6878, #1323, #10202, #2890, #9498, #2994, #3696, #2788, #2137 ),
 .UNSPECIFIED., .F., .F. ) 
 B_SPLINE_CURVE_WITH_KNOTS ( ( 4, 1, 1, 1, 1, 1, 1, 1, 1, 1, 1, 1, 1, 1, 1, 1, 1, 1, 1, 1, 1, 1, 1, 1, 1, 1, 1, 1, 1, 1, 1, 1, 1, 1, 1, 1, 1, 1, 1, 1, 1, 1, 1, 1, 1, 4 ),
 ( 0.000000000000000000, 0.01773478386796093625, 0.03606240600880961100, 0.05363178075044110205, 0.07078725724691559140, 0.08782600590454361922, 0.1049244321358663995, 0.1219539535917413542, 0.1389477140559601531, 0.1563980977818870410, 0.1746363666666245484, 0.1934786392176567060, 0.2128025958997298850, 0.2327904454208187812, 0.2535195744865274547, 0.2747166135707201362, 0.2963888843556201080, 0.3192629785013859078, 0.3441555232881252091, 0.3718650194528618225, 0.4028399612510209504, 0.4371448801346000668, 0.4747436484650962574, 0.5142463203427470875, 0.5531490499891791313, 0.5894092591003683435, 0.6223615841373315583, 0.6515869223714276792, 0.6772431252474833130, 0.7004011076753005050, 0.7222184512862198646, 0.7437909259358920222, 0.7652154438741737286, 0.7858628007620039879, 0.8056883297028475388, 0.8249734464625108066, 0.8436696960199348005, 0.8615821821759909183, 0.8789123401951898229, 0.8960241576542987696, 0.9130500659135333263, 0.9300436868743009455, 0.9471989324631484575, 0.9647777872405111088, 0.9830893744542027468, 1.000000000000000000 ),
 .UNSPECIFIED. ) 
 CURVE ( )  GEOMETRIC_REPRESENTATION_ITEM ( )  RATIONAL_B_SPLINE_CURVE ( ( 1.171573003563706195, 1.171573003563706195, 1.171573003563706195, 1.171573003563706195, 1.171573003563706195, 1.171573003563706195, 1.171573003563706195, 1.171573003563706195, 1.171573003563706195, 1.171573003563706195, 1.171573003563706195, 1.171573003563706195, 1.171573003563706195, 1.171573003563706195, 1.171573003563706195, 1.171573003563706195, 1.171573003563706195, 1.171573003563706195, 1.171573003563706195, 1.171573003563706195, 1.171573003563706195, 1.171573003563706195, 1.171573003563706195, 1.171573003563706195, 1.171573003563706195, 1.171573003563706195, 1.171573003563706195, 1.171573003563706195, 1.171573003563706195, 1.171573003563706195, 1.171573003563706195, 1.171573003563706195, 1.171573003563706195, 1.171573003563706195, 1.171573003563706195, 1.171573003563706195, 1.171573003563706195, 1.171573003563706195, 1.171573003563706195, 1.171573003563706195, 1.171573003563706195, 1.171573003563706195, 1.171573003563706195, 1.171573003563706195, 1.171573003563706195, 1.171573003563706195, 1.171573003563706195, 1.171573003563706195 ) ) 
 REPRESENTATION_ITEM ( '' )  );
#4693=CARTESIAN_POINT ( 'NONE',  ( -1.601785992426999705, -12.47016740323998718, -316.3802825947000201 ) ) ;
#4699=CARTESIAN_POINT ( 'NONE',  ( -13.84663869404836412, -6.024484023773889696, -314.5809261257323897 ) ) ;
#4704=CARTESIAN_POINT ( 'NONE',  ( -15.60753896450557221, -3.741771784933492828, 315.0000000000000568 ) ) ;
#4705=CARTESIAN_POINT ( 'NONE',  ( -20.05662131630997536, 0.5622531596958006972, -302.9207377450070453 ) ) ;
#4708=PLANE ( 'NONE',  #6613 ) ;
#4712=VECTOR ( 'NONE', #2899, 1000.000000000000000 ) ;
#4713=CARTESIAN_POINT ( 'NONE',  ( 14.97282077145999679, 8.399840787735001868, -302.9207377450070453 ) ) ;
#4716=CARTESIAN_POINT ( 'NONE',  ( -15.07109120124999890, -4.275483045295999318, -315.0848619657999734 ) ) ;
#4720=CARTESIAN_POINT ( 'NONE',  ( -4.407678726681998782, -11.78447947993998390, 189.9229057364800042 ) ) ;
#4721=CARTESIAN_POINT ( 'NONE',  ( -19.99997381626591064, 0.3203551279404593388, 190.9999999999996589 ) ) ;
#4726=CARTESIAN_POINT ( 'NONE',  ( -16.95904175860000151, -2.156867278632000229, 314.6383426456000052 ) ) ;
#4728=CARTESIAN_POINT ( 'NONE',  ( 13.47907531561000027, 8.083075672345000129, 320.0000000000000000 ) ) ;
#4729=CARTESIAN_POINT ( 'NONE',  ( -17.75416867407000154, -3.856294574926997232, 319.9928079742500131 ) ) ;
#4736=CARTESIAN_POINT ( 'NONE',  ( -14.59598702685000760, 8.048254220853003460, 189.9229057364800042 ) ) ;
#4737=CARTESIAN_POINT ( 'NONE',  ( 14.91230751981324154, 5.270530829718880206, 314.4999479601416965 ) ) ;
#4738=CARTESIAN_POINT ( 'NONE',  ( 20.00000000000000000, 4.642020101641720348E-09, -303.5000000000000000 ) ) ;
#4740=CARTESIAN_POINT ( 'NONE',  ( 15.48936016237493973, 3.890032586757016908, 315.0000000000000000 ) ) ;
#4742=CARTESIAN_POINT ( 'NONE',  ( -0.1638132020714603843, -12.51773231663031538, -303.4999999999996589 ) ) ;
#4745=CARTESIAN_POINT ( 'NONE',  ( -18.69275906597000869, 1.650694058049998469, 319.9928079742500131 ) ) ;
#4749=CARTESIAN_POINT ( 'NONE',  ( -9.398723296112997616, 11.12690316796998324, -317.0792622552969533 ) ) ;
#4750=CARTESIAN_POINT ( 'NONE',  ( 19.31691132429000390, -3.346581979927999217, -316.3802825947000201 ) ) ;
#4756=EDGE_LOOP ( 'NONE', ( #10079, #6301 ) ) ;
#4757=CARTESIAN_POINT ( 'NONE',  ( -7.848637230397551789, -11.50843006260753931, 319.0000000000003979 ) ) ;
#4759=CARTESIAN_POINT ( 'NONE',  ( 18.54292857607040546, 4.743390938996658868, -316.5000000000004547 ) ) ;
#4761=CARTESIAN_POINT ( 'NONE',  ( -8.900624420096743705, -8.081841135676405941, 314.9999999999999432 ) ) ;
#4762=CARTESIAN_POINT ( 'NONE',  ( -6.596975511883001353, -11.38119116100000028, -302.4229045757450081 ) ) ;
#4765=CARTESIAN_POINT ( 'NONE',  ( 10.56785312427999735, 10.70734743398999811, -302.9207377450070453 ) ) ;
#4766=CARTESIAN_POINT ( 'NONE',  ( 11.98520373079999679, -10.00909632395999438, 318.8802828394900644 ) ) ;
#4768=CARTESIAN_POINT ( 'NONE',  ( 4.001463906138999604, -9.408458373209999337, -314.8616023057000461 ) ) ;
#4771=CARTESIAN_POINT ( 'NONE',  ( -18.85519295008999663, -0.7686777388422003643, 190.0071920248299477 ) ) ;
#4773=CARTESIAN_POINT ( 'NONE',  ( 19.79199150660973672, 1.880421430186972387, 190.9999999999996589 ) ) ;
#4775=( BOUNDED_CURVE ( )  B_SPLINE_CURVE ( 3, ( #4039, #7318, #6560, #7263, #8117, #10427, #5531, #8982, #10477, #3119, #4893, #755, #1461, #3067, #6339, #6398, #2320, #4793, #1622, #4742, #10588, #8013, #9677, #5588, #7366, #5, #4843, #3230, #3178, #9842, #8923, #8064, #10534, #6452, #1567, #9788, #9732, #2375, #2426 ),
 .UNSPECIFIED., .F., .T. ) 
 B_SPLINE_CURVE_WITH_KNOTS ( ( 4, 1, 1, 1, 1, 1, 1, 1, 1, 1, 1, 1, 1, 1, 1, 1, 1, 1, 1, 1, 1, 1, 1, 1, 1, 1, 1, 1, 1, 1, 1, 1, 1, 1, 1, 1, 4 ),
 ( 0.000000000000000000, 0.03255837131920313876, 0.06556990764360209889, 0.09473136908033905068, 0.1200161462726948014, 0.1434330934855738704, 0.1672842806195496690, 0.1914679751100890337, 0.2155028411842019875, 0.2393474010340431724, 0.2632466635524260967, 0.2878286224669094340, 0.3134478398786056941, 0.3397600561265991526, 0.3667240395490957150, 0.3951494960372031739, 0.4259522906035831946, 0.4599907034545276940, 0.4966508108602697424, 0.5336723842619189861, 0.5687290606137788140, 0.6006810251919934007, 0.6302097713864017736, 0.6581574700887727891, 0.6853091452815190943, 0.7117521918490830046, 0.7371786555985277989, 0.7617219361653213561, 0.7857512081544899551, 0.8096666007474261351, 0.8337748265625605226, 0.8576111943424252759, 0.8809858201129860955, 0.9062047945899976975, 0.9352885204660792429, 0.9682251798361949380, 1.000000000000000000 ),
 .UNSPECIFIED. ) 
 CURVE ( )  GEOMETRIC_REPRESENTATION_ITEM ( )  RATIONAL_B_SPLINE_CURVE ( ( 1.171573374055207672, 1.171573374055207672, 1.171573374055207895, 1.171573374055207895, 1.171573374055207895, 1.171573374055207895, 1.171573374055207895, 1.171573374055207895, 1.171573374055207895, 1.171573374055207895, 1.171573374055207895, 1.171573374055207895, 1.171573374055207895, 1.171573374055207895, 1.171573374055207895, 1.171573374055207895, 1.171573374055207895, 1.171573374055207895, 1.171573374055207895, 1.171573374055207895, 1.171573374055207895, 1.171573374055207895, 1.171573374055207895, 1.171573374055207895, 1.171573374055207895, 1.171573374055207895, 1.171573374055207895, 1.171573374055207895, 1.171573374055207895, 1.171573374055207895, 1.171573374055207895, 1.171573374055207895, 1.171573374055207895, 1.171573374055207895, 1.171573374055207895, 1.171573374055207895, 1.171573374055207895, 1.171573374055207895, 1.171573374055207895 ) ) 
 REPRESENTATION_ITEM ( '' )  );
#4777=CARTESIAN_POINT ( 'NONE',  ( -6.419414596134000561, -9.427679607337001499, 314.4150829855000211 ) ) ;
#4780=B_SPLINE_CURVE_WITH_KNOTS ( 'NONE', 3,
 ( #4969, #834, #9867, #9811, #5017, #8196, #8244, #7234, #2347, #4116, #3364, #7444, #3304 ),
 .UNSPECIFIED., .F., .F.,
 ( 4, 1, 1, 1, 1, 1, 1, 1, 1, 1, 4 ),
 ( 0.000000000000000000, 0.08333333333333001192, 0.1666666666667000196, 0.2500000000000000000, 0.3333333333333000081, 0.5000000000000000000, 0.6666666666667000474, 0.7500000000000000000, 0.8333333333333000637, 0.9166666666667000474, 1.000000000000000000 ),
 .UNSPECIFIED. ) ;
#4781=CARTESIAN_POINT ( 'NONE',  ( -14.17215049938999982, 7.636433089049000422, 320.0000000000000000 ) ) ;
#4782=CARTESIAN_POINT ( 'NONE',  ( 11.51418862744999139, -9.000691300089004088, 319.9928079742500131 ) ) ;
#4783=CARTESIAN_POINT ( 'NONE',  ( -19.99999721132999753, 3.518711422920000253E-10, 319.0000000000000000 ) ) ;
#4786=VERTEX_POINT ( 'NONE', #6854 ) ;
#4788=CARTESIAN_POINT ( 'NONE',  ( -12.90475631688000746, 9.082603241465001531, 189.9229057364800042 ) ) ;
#4793=CARTESIAN_POINT ( 'NONE',  ( -3.693615097834042516, -12.29963531854552272, -303.4999999999996589 ) ) ;
#4795=CARTESIAN_POINT ( 'NONE',  ( -16.89041368998000081, -5.257268626091000208, -302.5000000000009663 ) ) ;
#4797=CARTESIAN_POINT ( 'NONE',  ( -4.335116381453002710, 11.79481621787999757, 320.0770942683900557 ) ) ;
#4800=CARTESIAN_POINT ( 'NONE',  ( -13.71837527932998491, 8.620941849619004671, -317.5770954168139610 ) ) ;
#4804=VERTEX_POINT ( 'NONE', #6752 ) ;
#4806=CARTESIAN_POINT ( 'NONE',  ( 16.91992689674542660, -1.077645906677548338, -315.0000000000000000 ) ) ;
#4807=ADVANCED_FACE ( 'NONE', ( #936 ), #6062, .F. ) ;
#4810=CARTESIAN_POINT ( 'NONE',  ( 14.75365836417945431, -8.451130538707891660, 319.0000000000003979 ) ) ;
#4812=CARTESIAN_POINT ( 'NONE',  ( -18.99984327789000105, 0.5550485914519999175, -317.4999999998989892 ) ) ;
#4814=CARTESIAN_POINT ( 'NONE',  ( -4.648656036509398959, -9.134414902114890822, 315.0000000000000568 ) ) ;
#4815=CARTESIAN_POINT ( 'NONE',  ( 6.445113046380004818, -11.41524423681998712, -302.4229045757450081 ) ) ;
#4820=CARTESIAN_POINT ( 'NONE',  ( 20.10115407781998442, 0.3730669878444000664, -302.9207377450070453 ) ) ;
#4821=CARTESIAN_POINT ( 'NONE',  ( -11.22625503481000209, -10.34655023142000907, 318.8802828394900644 ) ) ;
#4823=CARTESIAN_POINT ( 'NONE',  ( -15.71297435277999810, -3.490404421959999670, -315.0848619657999734 ) ) ;
#4826=CARTESIAN_POINT ( 'NONE',  ( -9.832070176257998284, -10.44777315889000313, 189.9229057364800042 ) ) ;
#4827=CARTESIAN_POINT ( 'NONE',  ( 0.7126779659676973910, 12.51265294199208000, 190.9999999999996589 ) ) ;
#4830=CARTESIAN_POINT ( 'NONE',  ( -3.903842856253999738, -9.647088721075000706, 314.6383426456000052 ) ) ;
#4831=CARTESIAN_POINT ( 'NONE',  ( -12.48775874806000097, 8.649334263351001084, 320.0000000000000000 ) ) ;
#4833=CARTESIAN_POINT ( 'NONE',  ( 7.848637230397552678, 11.50843006260754109, 319.0000000000005116 ) ) ;
#4834=LINE ( 'NONE', #9613, #5906 ) ;
#4835=ORIENTED_EDGE ( 'NONE', *, *, #833, .T. ) ;
#4836=CARTESIAN_POINT ( 'NONE',  ( -15.00000000000000000, 0.4945770392355999800, -285.0000000000000000 ) ) ;
#4840=EDGE_LOOP ( 'NONE', ( #2175, #7200, #9739, #8356 ) ) ;
#4842=CARTESIAN_POINT ( 'NONE',  ( 16.68818136459866253, 1.819152193222137059, 315.0000000000000000 ) ) ;
#4843=CARTESIAN_POINT ( 'NONE',  ( 10.52063983335276731, -10.64371280159997468, -303.4999999999996589 ) ) ;
#4844=CARTESIAN_POINT ( 'NONE',  ( 15.07109120124999890, 4.275483045295999318, -315.0848619657999734 ) ) ;
#4848=CARTESIAN_POINT ( 'NONE',  ( -19.85665319583999988, 1.941121513171000901, 319.5792614743400009 ) ) ;
#4853=CARTESIAN_POINT ( 'NONE',  ( 7.885457619219000236, 11.57957576882999184, -317.0792622552969533 ) ) ;
#4854=CARTESIAN_POINT ( 'NONE',  ( 16.87780931964001141, -6.722286650069999148, -316.3802825947000201 ) ) ;
#4856=CARTESIAN_POINT ( 'NONE',  ( 17.80730577449000052, -3.998365122558999563, 320.0000000000000000 ) ) ;
#4859=DIRECTION ( 'NONE',  ( -2.134661488198361529E-05, -5.799867325201099395E-11, -0.9999999997721611411 ) ) ;
#4860=CARTESIAN_POINT ( 'NONE',  ( -6.348506474365286145, 9.305625771097020049, -314.5281326612878843 ) ) ;
#4862=CARTESIAN_POINT ( 'NONE',  ( 19.95988936745280640, -0.9706423173584770581, 319.0000000000003979 ) ) ;
#4864=CARTESIAN_POINT ( 'NONE',  ( -3.763664787428660841, 12.29131725939111597, -316.5000000000004547 ) ) ;
#4866=CARTESIAN_POINT ( 'NONE',  ( 19.87644374459000929, -1.701742232560001788, -303.6197174156520759 ) ) ;
#4869=CARTESIAN_POINT ( 'NONE',  ( 12.85183647427999176, 9.678193536939003749, -302.9207377450070453 ) ) ;
#4873=CARTESIAN_POINT ( 'NONE',  ( -1.285290206351000108, -10.09749793447999977, -314.4150829855000211 ) ) ;
#4874=CARTESIAN_POINT ( 'NONE',  ( 14.32653628403999946, 7.536184728883000616, -302.5000000000000000 ) ) ;
#4876=CARTESIAN_POINT ( 'NONE',  ( -6.027267673561996553, -11.50416862954998365, 189.9229057364800042 ) ) ;
#4878=CARTESIAN_POINT ( 'NONE',  ( 4.603216684274966219, 9.141664750100051862, -315.0000000000000568 ) ) ;
#4881=CARTESIAN_POINT ( 'NONE',  ( -16.75097866579000083, -2.074182492207000461, 314.8616023057000461 ) ) ;
#4884=CARTESIAN_POINT ( 'NONE',  ( -18.87181153733000016, 0.3572136203155001355, 319.9928079742500131 ) ) ;
#4885=CARTESIAN_POINT ( 'NONE',  ( -2.572515036489481766, 12.41549478438273724, 319.0000000000005116 ) ) ;
#4886=CARTESIAN_POINT ( 'NONE',  ( 14.79012398733999945, 1.483731117707000058, 315.0000000000000000 ) ) ;
#4891=CARTESIAN_POINT ( 'NONE',  ( -15.00000000000000000, 0.000000000000000000, 315.0000000000000000 ) ) ;
#4892=CARTESIAN_POINT ( 'NONE',  ( 16.40981772118269788, 2.462276419762760682, 314.9999999999999432 ) ) ;
#4893=CARTESIAN_POINT ( 'NONE',  ( -12.81623431846863603, -9.609762277177447132, -303.4999999999996589 ) ) ;
#4894=CARTESIAN_POINT ( 'NONE',  ( 17.36972170382999892, 0.04551883977364000466, -314.6383426456000052 ) ) ;
#4895=EDGE_CURVE ( 'NONE', #8331, #4386, #5394, .T. ) ;
#4899=EDGE_CURVE ( 'NONE', #4067, #4512, #1020, .T. ) ;
#4902=CARTESIAN_POINT ( 'NONE',  ( 3.365463313584999838, 12.41489380075000604, -317.0792622552969533 ) ) ;
#4905=CARTESIAN_POINT ( 'NONE',  ( -8.770005493155000664, -10.19600538561000036, 320.0000000000000000 ) ) ;
#4908=CARTESIAN_POINT ( 'NONE',  ( -19.00000000000000000, 0.000000000000000000, -317.4999999998989892 ) ) ;
#4910=CARTESIAN_POINT ( 'NONE',  ( 15.45543459605807968, -3.931565522428362325, -315.0000000000000568 ) ) ;
#4911=ORIENTED_EDGE ( 'NONE', *, *, #9496, .F. ) ;
#4913=CARTESIAN_POINT ( 'NONE',  ( 15.67978886374999803, 4.575336738469999887, -314.4963898845653603 ) ) ;
#4915=CARTESIAN_POINT ( 'NONE',  ( 1.614076495133000000, 11.47540331082000087, -317.5000000000000000 ) ) ;
#4917=CARTESIAN_POINT ( 'NONE',  ( 16.01368207331000093, -7.610776120867003947, -302.9207377450070453 ) ) ;
#4920=CARTESIAN_POINT ( 'NONE',  ( 18.53523119387001117, 4.742105934366003694, -303.6197174156509391 ) ) ;
#4922=CARTESIAN_POINT ( 'NONE',  ( 1.279516016521960085E-07, 10.00000000000000000, 315.0000000000000000 ) ) ;
#4924=CARTESIAN_POINT ( 'NONE',  ( -16.95904175860000151, -2.156867278632000229, -314.6383426456000052 ) ) ;
#4926=EDGE_LOOP ( 'NONE', ( #3030, #3847, #6589, #3377 ) ) ;
#4927=CARTESIAN_POINT ( 'NONE',  ( -15.65104815535000071, -7.893060908445997725, 190.4207385301700128 ) ) ;
#4928=CARTESIAN_POINT ( 'NONE',  ( -19.95972666420564323, 0.9723020053078084146, 190.9999999999996305 ) ) ;
#4929=CARTESIAN_POINT ( 'NONE',  ( 16.33391464646021873, 2.612996577909529439, -314.9999999999999432 ) ) ;
#4931=CARTESIAN_POINT ( 'NONE',  ( 16.89986669904000394, -0.5583209492923999484, 315.0848619657999734 ) ) ;
#4933=CARTESIAN_POINT ( 'NONE',  ( -15.40147079910000372, -7.455286574312999903, 320.0770942683900557 ) ) ;
#4935=CARTESIAN_POINT ( 'NONE',  ( -18.18176685080253918, 5.227975112149439774, 319.0000000000005116 ) ) ;
#4936=CARTESIAN_POINT ( 'NONE',  ( 11.70471109486296868, 10.14826236475114740, -303.5000000000000000 ) ) ;
#4939=CARTESIAN_POINT ( 'NONE',  ( 17.49999999954662044, -9.625715914672042649E-06, 190.0000000000000000 ) ) ;
#4942=CARTESIAN_POINT ( 'NONE',  ( -20.00000000000000000, 7.277416212200430041E-10, -316.5000000000000000 ) ) ;
#4943=CARTESIAN_POINT ( 'NONE',  ( 16.37744599325981909, 2.527607301898085801, 314.9999999999999432 ) ) ;
#4944=CARTESIAN_POINT ( 'NONE',  ( 15.00000000000000000, -0.4945770392355999800, -285.0000000000000000 ) ) ;
#4945=CARTESIAN_POINT ( 'NONE',  ( 17.59334121105999671, 0.04733121045982999903, -314.4150829855000211 ) ) ;
#4948=CARTESIAN_POINT ( 'NONE',  ( -14.98664244983999971, 7.043920630080999778, 190.0000000000000000 ) ) ;
#4950=CARTESIAN_POINT ( 'NONE',  ( -19.99999721132999753, 3.518711422920000253E-10, 319.0000000000000000 ) ) ;
#4952=CARTESIAN_POINT ( 'NONE',  ( -14.96823785528000528, 8.299997444912003530, -316.3802825947000201 ) ) ;
#4955=CARTESIAN_POINT ( 'NONE',  ( 9.597846547914999249, -9.915773017694000657, 320.0000000000000000 ) ) ;
#4960=CARTESIAN_POINT ( 'NONE',  ( 2.737251867098380753, -9.374957062059573687, -315.0000000000000000 ) ) ;
#4962=CARTESIAN_POINT ( 'NONE',  ( 8.037373804805000077, 9.179324345868998591, -314.4963898845653603 ) ) ;
#4964=CARTESIAN_POINT ( 'NONE',  ( -3.698987565691999713, 11.29118203779999874, -317.5000000000000000 ) ) ;
#4966=CARTESIAN_POINT ( 'NONE',  ( 20.10149561490999659, -0.3453761138107002138, -302.9207377450070453 ) ) ;
#4968=CARTESIAN_POINT ( 'NONE',  ( 5.133129775586001031, -10.95790389472999316, -317.4928077629770087 ) ) ;
#4969=CARTESIAN_POINT ( 'NONE',  ( -15.00000000000000000, 0.000000000000000000, 315.0000000000000000 ) ) ;
#4971=CARTESIAN_POINT ( 'NONE',  ( -15.02162735728999543, 8.365494092177003793, -302.9207377450070453 ) ) ;
#4973=ORIENTED_EDGE ( 'NONE', *, *, #1113, .T. ) ;
#4977=CARTESIAN_POINT ( 'NONE',  ( -20.06711733022002164, 0.4206966322103999900, 190.4207385301700128 ) ) ;
#4978=CARTESIAN_POINT ( 'NONE',  ( 17.50000000000125056, 1.380497925828168986E-12, -314.4944826805096341 ) ) ;
#4979=CARTESIAN_POINT ( 'NONE',  ( 16.78721195431734259, 1.718634075882272239, -314.9999999999999432 ) ) ;
#4981=CARTESIAN_POINT ( 'NONE',  ( -13.99304003883001180, 8.933243331610997373, 191.1197171614399792 ) ) ;
#4986=CARTESIAN_POINT ( 'NONE',  ( -16.10430118153999857, -6.867346955731005842, 320.0770942683900557 ) ) ;
#4988=CARTESIAN_POINT ( 'NONE',  ( 8.450675645183000739, 8.177559542660000957, 315.0848619657999734 ) ) ;
#4989=VECTOR ( 'NONE', #8099, 1000.000000000000000 ) ;
#4990=ORIENTED_EDGE ( 'NONE', *, *, #3001, .T. ) ;
#4993=CARTESIAN_POINT ( 'NONE',  ( -10.02519493912904380, 7.672398658596809362, 315.0000000000000568 ) ) ;
#4998=CARTESIAN_POINT ( 'NONE',  ( 18.53584076651999979, 2.541936159385000060, 190.0000000000000000 ) ) ;
#5001=CARTESIAN_POINT ( 'NONE',  ( -2.055393166047998932, 12.44351316864999824, -316.3802825947000201 ) ) ;
#5007=CARTESIAN_POINT ( 'NONE',  ( 16.40967564559107572, -2.462589562615133065, -315.0000000000000000 ) ) ;
#5010=CARTESIAN_POINT ( 'NONE',  ( 12.98706127646999953, 6.788989183774999603, -315.0000000000001137 ) ) ;
#5012=CARTESIAN_POINT ( 'NONE',  ( 11.26076953950000004, 9.251451169536998975, -317.5000000000000000 ) ) ;
#5014=CARTESIAN_POINT ( 'NONE',  ( -16.84215363705000712, -6.757103037815999969, -303.6197174156509391 ) ) ;
#5016=CARTESIAN_POINT ( 'NONE',  ( 13.35621109890998959, -8.022534180767001644, -317.4928077629770087 ) ) ;
#5017=CARTESIAN_POINT ( 'NONE',  ( -11.28781796570999951, -4.951468039558000633, 315.0000000000000000 ) ) ;
#5018=( NAMED_UNIT ( * ) SI_UNIT ( $, .STERADIAN. ) SOLID_ANGLE_UNIT ( ) );
#5019=CARTESIAN_POINT ( 'NONE',  ( -20.05676974677001922, -0.5613724988767001545, -302.9207377450070453 ) ) ;
#5022=FACE_OUTER_BOUND ( 'NONE', #4321, .T. ) ;
#5023=ADVANCED_FACE ( 'NONE', ( #10363 ), #2900, .T. ) ;
#5026=CARTESIAN_POINT ( 'NONE',  ( -20.04745173227997768, -0.9063373766989004654, 190.4207385301700128 ) ) ;
#5029=EDGE_CURVE ( 'NONE', #8305, #4804, #7684, .T. ) ;
#5031=CARTESIAN_POINT ( 'NONE',  ( -1.248913580286000302, 12.48838264809999643, 191.1197171614399792 ) ) ;
#5033=CARTESIAN_POINT ( 'NONE',  ( 8.759386130138000937, -8.782224002452998946, 314.4150829855000211 ) ) ;
#5036=CARTESIAN_POINT ( 'NONE',  ( -11.06499621481999895, -9.965574156584002807, 320.0770942683900557 ) ) ;
#5039=B_SPLINE_CURVE_WITH_KNOTS ( 'NONE', 3,
 ( #2721, #6911, #6807, #3530, #10080, #4387, #6041, #6144, #2067, #8410, #2825, #4532, #3630, #1914, #399, #1254, #5331, #5236, #4333, #6965, #5284, #8607, #5987, #9282, #7606, #5186, #6858, #2017, #10239, #8556, #9480, #3730, #10287, #3579, #7810, #456, #1202, #10129, #7757, #8459, #301, #7017, #2926, #1101, #4433, #8511, #4477, #1153 ),
 .UNSPECIFIED., .F., .F.,
 ( 4, 1, 1, 1, 1, 1, 1, 1, 1, 1, 1, 1, 1, 1, 1, 1, 1, 1, 1, 1, 1, 1, 1, 1, 1, 1, 1, 1, 1, 1, 1, 1, 1, 1, 1, 1, 1, 1, 1, 1, 1, 1, 1, 1, 1, 4 ),
 ( 0.000000000000000000, 0.02222222222221999915, 0.04444444444443999831, 0.06666666666666999641, 0.08888888888889000250, 0.1111111111111000027, 0.1333333333332999970, 0.1555555555555999947, 0.1777777777777999890, 0.2000000000000000111, 0.2222222222222000054, 0.2444444444443999997, 0.2666666666666999697, 0.2888888888889000195, 0.3111111111111000138, 0.3333333333333000081, 0.3555555555556000336, 0.3777777777777999724, 0.4000000000000000222, 0.4222222222221999610, 0.4444444444444000109, 0.4666666666666999808, 0.4888888888889000306, 0.5111111111110999694, 0.5333333333333000192, 0.5555555555555999891, 0.5777777777778000390, 0.5999999999999999778, 0.6222222222222000276, 0.6444444444443999664, 0.6666666666667000474, 0.6888888888888999862, 0.7111111111111000360, 0.7333333333333000859, 0.7555555555556000558, 0.7777777777777999946, 0.8000000000000000444, 0.8222222222221999832, 0.8444444444443999220, 0.8666666666667000030, 0.8888888888888999418, 0.9111111111110999916, 0.9333333333333000414, 0.9555555555556000114, 0.9777777777778000612, 1.000000000000000000 ),
 .UNSPECIFIED. ) ;
#5040=CARTESIAN_POINT ( 'NONE',  ( 16.92248268936999978, 0.04189409840125999512, 315.0848619657999734 ) ) ;
#5042=CARTESIAN_POINT ( 'NONE',  ( -11.03108320835583278, -10.43614982842405681, 190.9999999999995737 ) ) ;
#5043=CARTESIAN_POINT ( 'NONE',  ( -19.56939737065003015, 2.860667089442002986, 319.5792614743400009 ) ) ;
#5046=CARTESIAN_POINT ( 'NONE',  ( 0.7882946689300455168, 9.499899501988618766, 315.0000000000000000 ) ) ;
#5047=CARTESIAN_POINT ( 'NONE',  ( -11.28781796570999951, -4.951468039558000633, -285.0000000000000000 ) ) ;
#5054=CARTESIAN_POINT ( 'NONE',  ( -16.37727794820371585, 2.527950228764471952, -315.0000000000001137 ) ) ;
#5057=CARTESIAN_POINT ( 'NONE',  ( 9.192918156740001123, 11.10629030388999894, -316.3802825947000201 ) ) ;
#5061=UNCERTAINTY_MEASURE_WITH_UNIT (LENGTH_MEASURE( 1.000000000000000082E-05 ), #9060, 'distance_accuracy_value', 'NONE');
#5063=CARTESIAN_POINT ( 'NONE',  ( 8.666289393444031930, -8.161235200486094854, -315.0000000000000000 ) ) ;
#5065=CARTESIAN_POINT ( 'NONE',  ( 17.21226690345150701, -1.804990710747416571, -314.5172708043664898 ) ) ;
#5067=CARTESIAN_POINT ( 'NONE',  ( 12.33668477992999968, 8.731648389349999206, -317.5000000000000000 ) ) ;
#5069=CARTESIAN_POINT ( 'NONE',  ( -0.1637764853584998959, -12.51053635490000282, -303.6197174156509391 ) ) ;
#5070=CARTESIAN_POINT ( 'NONE',  ( 14.73022282720999598, -7.961369676960005748, -317.5770954168139610 ) ) ;
#5071=CARTESIAN_POINT ( 'NONE',  ( -16.90171868104999930, -0.3834349726278000192, -315.0848619657999734 ) ) ;
#5074=CARTESIAN_POINT ( 'NONE',  ( 12.81291305286001858, 9.603378439332990624, -303.6197174156509391 ) ) ;
#5080=CARTESIAN_POINT ( 'NONE',  ( 20.06806562977000752, 0.4074806926876002322, 190.4207385301700128 ) ) ;
#5081=CARTESIAN_POINT ( 'NONE',  ( 17.50000000000126832, -0.7437989020612977287, -315.0000000000001705 ) ) ;
#5084=CARTESIAN_POINT ( 'NONE',  ( -19.97280825118999914, -0.5561396363675005228, 191.1197171614399792 ) ) ;
#5086=CARTESIAN_POINT ( 'NONE',  ( 17.59298685096999648, -0.02218567204013999900, 314.4150829855000211 ) ) ;
#5088=CARTESIAN_POINT ( 'NONE',  ( -12.95511329522999233, -9.055231460430995583, 320.0770942683900557 ) ) ;
#5091=CARTESIAN_POINT ( 'NONE',  ( 16.58659719219999928, 2.947707964209000053, 314.6383426456000052 ) ) ;
#5093=CARTESIAN_POINT ( 'NONE',  ( -14.79888371878074693, -8.420183212156704400, 190.9999999999995737 ) ) ;
#5095=CARTESIAN_POINT ( 'NONE',  ( -9.940815099545000422, 10.93780185275999983, 319.5792614743400009 ) ) ;
#5096=( BOUNDED_CURVE ( )  B_SPLINE_CURVE ( 3, ( #8397, #5224, #1142, #10017, #5174, #6085, #2710, #6901, #1902, #188, #6797, #5120, #7647, #984, #8548, #10230, #288, #3462, #2008, #9217, #1955, #2864, #3516, #7748, #4469, #4422, #1087, #7698, #1036, #242, #4323, #3566, #341, #6135, #6847, #2056, #3621, #2658, #1850 ),
 .UNSPECIFIED., .F., .F. ) 
 B_SPLINE_CURVE_WITH_KNOTS ( ( 4, 1, 1, 1, 1, 1, 1, 1, 1, 1, 1, 1, 1, 1, 1, 1, 1, 1, 1, 1, 1, 1, 1, 1, 1, 1, 1, 1, 1, 1, 1, 1, 1, 1, 1, 1, 4 ),
 ( 0.000000000000000000, 0.03177462182248536743, 0.06473445752888724869, 0.09385364856954842017, 0.1191010430400946118, 0.1424790257418310502, 0.1662901096498168863, 0.1904342604133079375, 0.2144298290992798506, 0.2382345388122189267, 0.2620932284128464906, 0.2866356387947044948, 0.3122179111685366992, 0.3384928023102440897, 0.3654153534982623741, 0.3937977678961502859, 0.4245599715672168095, 0.4585656223635954931, 0.4952131905531249600, 0.5322445193856789603, 0.5673324073471927020, 0.5993259174520090271, 0.6288994963735405896, 0.6568908825538779528, 0.6840816459652389048, 0.7105624348628040154, 0.7360296225686681071, 0.7606150911898692524, 0.7846847747132010831, 0.8086388669220148095, 0.8327860209783324308, 0.8566619651612988884, 0.8800749352578085549, 0.9053303401216608037, 0.9344548807899611953, 0.9674420121560727281, 1.000000000000000000 ),
 .UNSPECIFIED. ) 
 CURVE ( )  GEOMETRIC_REPRESENTATION_ITEM ( )  RATIONAL_B_SPLINE_CURVE ( ( 1.171573374019466929, 1.171573374019466707, 1.171573374019466929, 1.171573374019466929, 1.171573374019466929, 1.171573374019466929, 1.171573374019466929, 1.171573374019466929, 1.171573374019466929, 1.171573374019466929, 1.171573374019466929, 1.171573374019466929, 1.171573374019466929, 1.171573374019466929, 1.171573374019466929, 1.171573374019466929, 1.171573374019466929, 1.171573374019466929, 1.171573374019466929, 1.171573374019466929, 1.171573374019466929, 1.171573374019466929, 1.171573374019466929, 1.171573374019466929, 1.171573374019466929, 1.171573374019466929, 1.171573374019466929, 1.171573374019466929, 1.171573374019466929, 1.171573374019466929, 1.171573374019466929, 1.171573374019466929, 1.171573374019466929, 1.171573374019466929, 1.171573374019466929, 1.171573374019466929, 1.171573374019466929, 1.171573374019466929, 1.171573374019466929 ) ) 
 REPRESENTATION_ITEM ( '' )  );
#5101=CARTESIAN_POINT ( 'NONE',  ( -2.257382111677873393, 9.415175415973715545, 315.0000000000000000 ) ) ;
#5104=CARTESIAN_POINT ( 'NONE',  ( 18.86992372454000133, -1.611776198549999872, -302.4999999999529905 ) ) ;
#5107=CARTESIAN_POINT ( 'NONE',  ( 17.44869542667227691, -0.8969788568403171958, 314.4999390965244288 ) ) ;
#5117=CARTESIAN_POINT ( 'NONE',  ( 5.242074483217282754, -9.033702059254418160, -314.9999999999999432 ) ) ;
#5119=CARTESIAN_POINT ( 'NONE',  ( 17.50000000000000000, 0.000000000000000000, -314.4999343908002629 ) ) ;
#5120=CARTESIAN_POINT ( 'NONE',  ( 11.75848697160781064, -10.12394145745024687, -316.5000000000004547 ) ) ;
#5122=CARTESIAN_POINT ( 'NONE',  ( -17.62858316411999837, 4.302404616280000482, -317.5000000000030127 ) ) ;
#5123=EDGE_LOOP ( 'NONE', ( #9174, #6405, #7867, #1687 ) ) ;
#5125=CARTESIAN_POINT ( 'NONE',  ( 18.93734960604998463, -3.176822791883000985, -317.5770954168139610 ) ) ;
#5128=CARTESIAN_POINT ( 'NONE',  ( -14.97309261602000419, 8.296494983500004139, -303.6197174156520759 ) ) ;
#5129=CARTESIAN_POINT ( 'NONE',  ( -6.176342266831065686, -9.366307616516619916, 314.4999456809351273 ) ) ;
#5134=CARTESIAN_POINT ( 'NONE',  ( 4.867894159875999271, -12.21747625305000007, 190.4207385301700128 ) ) ;
#5137=CARTESIAN_POINT ( 'NONE',  ( -18.17619403612001250, 5.223318733890998544, 191.1197171614399792 ) ) ;
#5139=AXIS2_PLACEMENT_3D ( 'NONE', #2334, #871, #3243 ) ;
#5142=CARTESIAN_POINT ( 'NONE',  ( 16.41165915566000066, -2.800979832323999830, 314.8616023057000461 ) ) ;
#5144=CARTESIAN_POINT ( 'NONE',  ( 19.37251270682998694, -1.820313540576997680, 320.0770942683900557 ) ) ;
#5145=CARTESIAN_POINT ( 'NONE',  ( -3.206477623445924685, 9.870911232215625830, 314.4999441614609736 ) ) ;
#5146=CARTESIAN_POINT ( 'NONE',  ( 8.032401884333960851, 11.45915766226284482, -303.4999999999990905 ) ) ;
#5147=CARTESIAN_POINT ( 'NONE',  ( 14.52969073417999901, 5.422537850045999974, 314.6383426456000052 ) ) ;
#5150=CARTESIAN_POINT ( 'NONE',  ( 3.213253768582002845, 12.43294388789000138, 319.5792614743400009 ) ) ;
#5152=ADVANCED_FACE ( 'NONE', ( #6551 ), #8726, .T. ) ;
#5155=CARTESIAN_POINT ( 'NONE',  ( -2.158263635479988896, 9.422507356620213770, 315.0000000000001137 ) ) ;
#5159=CARTESIAN_POINT ( 'NONE',  ( 16.90628502044000214, -5.238535436438000126, -302.5000000000009663 ) ) ;
#5162=EDGE_CURVE ( 'NONE', #1953, #4467, #1388, .T. ) ;
#5163=CARTESIAN_POINT ( 'NONE',  ( -14.89798725392377321, 4.565017050278197708, -315.0000000000000568 ) ) ;
#5164=CARTESIAN_POINT ( 'NONE',  ( 8.506801009283002202, 10.15345907998999486, 190.0071920248299477 ) ) ;
#5170=BREP_WITH_VOIDS ( 'NONE', #8143, ( #100, #8823 ) );
#5172=B_SPLINE_CURVE_WITH_KNOTS ( 'NONE', 3,
 ( #8054, #2421, #8974, #1616, #3972, #7255, #9727, #5633, #9834, #7361, #4084, #4836, #1831 ),
 .UNSPECIFIED., .F., .F.,
 ( 4, 1, 1, 1, 1, 1, 1, 1, 1, 1, 4 ),
 ( 0.000000000000000000, 0.08333333333333001192, 0.1666666666667000196, 0.2500000000000000000, 0.3333333333333000081, 0.5000000000000000000, 0.6666666666667000474, 0.7500000000000000000, 0.8333333333333000637, 0.9166666666667000474, 1.000000000000000000 ),
 .UNSPECIFIED. ) ;
#5173=CARTESIAN_POINT ( 'NONE',  ( 1.281333103385001726, 11.37293729856000368, 319.9928079742500131 ) ) ;
#5174=CARTESIAN_POINT ( 'NONE',  ( 18.56670159326493064, -4.707099758006331847, -316.5000000000004547 ) ) ;
#5178=CARTESIAN_POINT ( 'NONE',  ( -10.19016500772999656, 9.569509725303996461, -317.4928077629770087 ) ) ;
#5179=CARTESIAN_POINT ( 'NONE',  ( 16.88563860788000781, -5.080169144092001154, -317.4928077629770087 ) ) ;
#5182=CARTESIAN_POINT ( 'NONE',  ( -17.18263598829999950, 2.199757124398999952, -314.4150829855000211 ) ) ;
#5184=CARTESIAN_POINT ( 'NONE',  ( -9.995120163707431615, -8.217201912095820404, 314.4999464406706693 ) ) ;
#5186=CARTESIAN_POINT ( 'NONE',  ( -2.585384220735000405, -11.41066401029999966, 190.0000000000000000 ) ) ;
#5187=CARTESIAN_POINT ( 'NONE',  ( -19.99996733365994928, -0.3063832366037745891, 319.0000000000003979 ) ) ;
#5192=CARTESIAN_POINT ( 'NONE',  ( 20.06711733022002164, -0.4206966322103001255, 190.4207385301700128 ) ) ;
#5197=CARTESIAN_POINT ( 'NONE',  ( 19.19790409518002861, -3.716965664678998582, 319.5792614743400009 ) ) ;
#5199=CARTESIAN_POINT ( 'NONE',  ( 16.21525914616999842, -2.693567875512000054, -315.0848619657999734 ) ) ;
#5200=CARTESIAN_POINT ( 'NONE',  ( -10.58688533405000065, 7.844683714540999553, 314.6383426456000052 ) ) ;
#5202=CARTESIAN_POINT ( 'NONE',  ( 16.34529002343605697, -7.216405960070772174, 190.9999999999995737 ) ) ;
#5203=CARTESIAN_POINT ( 'NONE',  ( 20.00482943604999164, 0.07455149923640995435, 318.8802828394900644 ) ) ;
#5205=CARTESIAN_POINT ( 'NONE',  ( 9.619189022994751426, 7.822639675800805215, 315.0000000000000000 ) ) ;
#5206=CARTESIAN_POINT ( 'NONE',  ( -17.50000003227012613, 5.857864393370422640, 314.9999999999999432 ) ) ;
#5212=CARTESIAN_POINT ( 'NONE',  ( -16.03969916442341415, 3.142024325209860081, -314.9999999999999432 ) ) ;
#5213=FACE_OUTER_BOUND ( 'NONE', #6845, .T. ) ;
#5224=CARTESIAN_POINT ( 'NONE',  ( 19.99979366059626074, -0.5741561031401761772, -316.5000000000005684 ) ) ;
#5226=ORIENTED_EDGE ( 'NONE', *, *, #8269, .T. ) ;
#5228=CARTESIAN_POINT ( 'NONE',  ( -18.90091799877999179, 0.2928069713013998765, -317.4928077629770087 ) ) ;
#5230=CARTESIAN_POINT ( 'NONE',  ( -18.92046274781997894, -3.214434834450002221, -317.5770954168139610 ) ) ;
#5236=CARTESIAN_POINT ( 'NONE',  ( 9.801682940292002044, -9.841837802148999614, 190.0000000000000000 ) ) ;
#5237=CARTESIAN_POINT ( 'NONE',  ( -19.96236207922240879, -0.9438262771025411890, 319.0000000000003979 ) ) ;
#5238=APPLICATION_CONTEXT ( 'automotive_design' ) ;
#5240=CARTESIAN_POINT ( 'NONE',  ( -19.99979366059625718, 0.5741561031401783977, -316.5000000000005116 ) ) ;
#5245=EDGE_CURVE ( 'NONE', #9105, #8720, #9920, .T. ) ;
#5248=CARTESIAN_POINT ( 'NONE',  ( 7.514439085588995759, -11.67576679883001667, 319.5792614743400009 ) ) ;
#5249=CARTESIAN_POINT ( 'NONE',  ( 16.41165915566000066, -2.800979832323999830, -314.8616023057000461 ) ) ;
#5250=CARTESIAN_POINT ( 'NONE',  ( -10.67587555525000020, 8.049811041412000989, 314.4150829855000211 ) ) ;
#5252=CARTESIAN_POINT ( 'NONE',  ( 12.57201637590000942, -8.467554047266999007, 190.0071920248299477 ) ) ;
#5254=CARTESIAN_POINT ( 'NONE',  ( 12.21300849950000433, 9.900542285453001412, 318.8802828394900644 ) ) ;
#5256=CARTESIAN_POINT ( 'NONE',  ( -17.56970546055000071, 0.4338786413876999926, 314.4150829855000211 ) ) ;
#5257=CARTESIAN_POINT ( 'NONE',  ( -16.13945612244922501, 2.966804785441415238, 314.9999999999999432 ) ) ;
#5259=CARTESIAN_POINT ( 'NONE',  ( 15.00000000000325961, 7.547804830080786473E-15, 315.0000000000001705 ) ) ;
#5262=CARTESIAN_POINT ( 'NONE',  ( -16.45380452100018687, 2.370995337294541816, -315.0000000000000568 ) ) ;
#5263=CARTESIAN_POINT ( 'NONE',  ( 9.595833218033995138, 9.789665514059997520, 190.0071920248299477 ) ) ;
#5265=CARTESIAN_POINT ( 'NONE',  ( -19.00000000000000000, 0.000000000000000000, -317.4999999998989892 ) ) ;
#5268=CARTESIAN_POINT ( 'NONE',  ( 13.94549574055089458, -5.407931305651876741, 315.0000000000001137 ) ) ;
#5269=CARTESIAN_POINT ( 'NONE',  ( -12.07130791617000121, 6.858215270785999351, -314.8616023057000461 ) ) ;
#5272=CARTESIAN_POINT ( 'NONE',  ( -9.539154743984001428, 9.809959732869000248, 319.9928079742500131 ) ) ;
#5276=CARTESIAN_POINT ( 'NONE',  ( 6.235150775465998052, 10.74512744517000407, -317.4928077629770087 ) ) ;
#5277=ADVANCED_FACE ( 'NONE', ( #6056 ), #7691, .F. ) ;
#5278=CARTESIAN_POINT ( 'NONE',  ( 3.772811979575000141, -12.36790329786001763, -317.0792622552969533 ) ) ;
#5280=CARTESIAN_POINT ( 'NONE',  ( 17.19853431800999743, -2.231396706187000145, -315.0000000000000000 ) ) ;
#5283=ORIENTED_EDGE ( 'NONE', *, *, #7709, .F. ) ;
#5284=CARTESIAN_POINT ( 'NONE',  ( 6.280550016735999996, -10.85821747223999978, 190.0000000000000000 ) ) ;
#5285=CARTESIAN_POINT ( 'NONE',  ( -18.21047658595729857, -5.188723016677323052, 319.0000000000003979 ) ) ;
#5287=CARTESIAN_POINT ( 'NONE',  ( -17.02428600387000301, -6.565037456673000982, 191.1197171614399792 ) ) ;
#5290=CARTESIAN_POINT ( 'NONE',  ( -16.85751871341000907, -5.113642021703998175, -302.5071922382879279 ) ) ;
#5295=CARTESIAN_POINT ( 'NONE',  ( -3.306880204566999382, 11.21686954173999951, -302.5071922382879279 ) ) ;
#5296=CARTESIAN_POINT ( 'NONE',  ( -17.04162109443001683, -6.546751591322998109, 318.8802828394900644 ) ) ;
#5297=CARTESIAN_POINT ( 'NONE',  ( 17.56954514911999965, 0.4333932196220999788, -314.4150829855000211 ) ) ;
#5298=CARTESIAN_POINT ( 'NONE',  ( -4.061138133959000029, 9.851562218542998295, 314.4150829855000211 ) ) ;
#5300=CARTESIAN_POINT ( 'NONE',  ( -2.556522775252001445, -11.29259618907000196, 190.0071920248299477 ) ) ;
#5302=CARTESIAN_POINT ( 'NONE',  ( -11.98520373079999679, 10.00909632395999438, 318.8802828394900644 ) ) ;
#5307=CARTESIAN_POINT ( 'NONE',  ( -14.79012398733999767, -1.483731117707002278, -284.9999999999999432 ) ) ;
#5309=CARTESIAN_POINT ( 'NONE',  ( -15.88699210612483981, -3.373196549223931306, -314.9999999999999432 ) ) ;
#5311=CARTESIAN_POINT ( 'NONE',  ( 17.33328289455321425, 2.867118450878387397E-08, 314.6666162271451981 ) ) ;
#5313=CARTESIAN_POINT ( 'NONE',  ( -10.54249803899487326, 7.451732067202640586, -315.0000000000000000 ) ) ;
#5314=CARTESIAN_POINT ( 'NONE',  ( 14.91611818836001824, 6.947523351336002406, 190.0071920248299477 ) ) ;
#5316=CARTESIAN_POINT ( 'NONE',  ( -1.614076495133000000, -11.47540331082000087, -317.5000000000000000 ) ) ;
#5317=CARTESIAN_POINT ( 'NONE',  ( 19.00000000000000000, 0.000000000000000000, -317.4999999998989892 ) ) ;
#5318=CARTESIAN_POINT ( 'NONE',  ( 13.67632236045006167, -5.618997091738346050, 315.0000000000000000 ) ) ;
#5319=CARTESIAN_POINT ( 'NONE',  ( -11.96281778373999849, 6.662668310474999522, -315.0848619657999734 ) ) ;
#5324=CARTESIAN_POINT ( 'NONE',  ( 11.21026319665000948, 9.143022107836994650, -317.4928077629770087 ) ) ;
#5325=ADVANCED_FACE ( 'NONE', ( #5022 ), #944, .F. ) ;
#5326=CARTESIAN_POINT ( 'NONE',  ( 5.336288444022999400, -12.13785676344998699, -317.0792622552969533 ) ) ;
#5329=CARTESIAN_POINT ( 'NONE',  ( 17.44177680037102007, 0.9115828329869209989, -314.5029970719331232 ) ) ;
#5331=CARTESIAN_POINT ( 'NONE',  ( 10.77777196380999847, -9.457622649256999026, 190.0000000000000000 ) ) ;
#5333=CARTESIAN_POINT ( 'NONE',  ( -19.99999036626000048, -4.642009783819999925E-09, -316.5000000000000000 ) ) ;
#5337=CARTESIAN_POINT ( 'NONE',  ( 7.636686903722000430, -10.40663048292000070, -302.5071922382879279 ) ) ;
#5338=CARTESIAN_POINT ( 'NONE',  ( 18.70579689905999032, 4.435290649195002821, 191.1197171614399792 ) ) ;
#5343=CARTESIAN_POINT ( 'NONE',  ( 18.77308876972001173, 1.495304374661000413, -302.5071922382879279 ) ) ;
#5344=CARTESIAN_POINT ( 'NONE',  ( -19.14248421182001891, -3.638193899013998145, 318.8802828394900644 ) ) ;
#5346=CARTESIAN_POINT ( 'NONE',  ( 17.36938240862999905, -0.02134527931160000100, -314.6383426456000052 ) ) ;
#5347=CARTESIAN_POINT ( 'NONE',  ( -16.92217352393999974, 0.01966449385449000123, 315.0848619657999734 ) ) ;
#5354=EDGE_CURVE ( 'NONE', #4571, #2720, #5039, .T. ) ;
#5357=CARTESIAN_POINT ( 'NONE',  ( 18.78897325516000194, 1.756194273835000041, 320.0000000000000000 ) ) ;
#5358=CARTESIAN_POINT ( 'NONE',  ( 15.00000000000072120, -0.4945770392355430256, -284.9999999999999432 ) ) ;
#5362=CARTESIAN_POINT ( 'NONE',  ( 4.532042191365901473, 9.152867265080528725, -315.0000000000000568 ) ) ;
#5364=CARTESIAN_POINT ( 'NONE',  ( 17.16660215780888166, 1.253876006774286806E-08, -314.8332688233516024 ) ) ;
#5365=ORIENTED_EDGE ( 'NONE', *, *, #9764, .T. ) ;
#5371=CARTESIAN_POINT ( 'NONE',  ( 11.69610966801475449, -6.874282731906364852, 315.0000000000000000 ) ) ;
#5372=CARTESIAN_POINT ( 'NONE',  ( 14.67553856548000013, 5.592168771406000438, -314.4150829855000211 ) ) ;
#5375=CARTESIAN_POINT ( 'NONE',  ( -18.85102544288001170, 0.8044398135754999846, 319.9928079742500131 ) ) ;
#5379=CARTESIAN_POINT ( 'NONE',  ( -14.73022282720999598, 7.961369676960005748, -317.5770954168139610 ) ) ;
#5380=CARTESIAN_POINT ( 'NONE',  ( -19.95007997204999839, -1.762487863542002486, -317.0792622552969533 ) ) ;
#5384=CARTESIAN_POINT ( 'NONE',  ( 17.50000000158812696, 0.4607171203178882513, -314.4995147730188592 ) ) ;
#5393=CARTESIAN_POINT ( 'NONE',  ( -17.60320223513998172, -4.128492944088002048, -302.5071922382879279 ) ) ;
#5394=B_SPLINE_CURVE_WITH_KNOTS ( 'NONE', 3,
 ( #7212, #3120, #5589, #3281, #1515, #4795, #8066, #5639, #8924, #9789, #2427, #5695, #1568, #3554, #10104, #3394, #7632, #8431, #4145, #970, #10056, #8276, #5910, #4256, #7477, #5801, #9203, #1887, #8384, #6784, #6725, #2746, #1837, #5159, #1939, #3340, #5104, #5851, #7527 ),
 .UNSPECIFIED., .F., .F.,
 ( 4, 1, 1, 1, 1, 1, 1, 1, 1, 1, 1, 1, 1, 1, 1, 1, 1, 1, 1, 1, 1, 1, 1, 1, 1, 1, 1, 1, 1, 1, 1, 1, 1, 1, 1, 1, 4 ),
 ( 0.000000000000000000, 0.02777777777778000015, 0.05555555555556000030, 0.08333333333333001192, 0.1111111111111000027, 0.1388888888888999973, 0.1666666666667000196, 0.1944444444444000109, 0.2222222222222000054, 0.2500000000000000000, 0.2777777777777999946, 0.3055555555555999891, 0.3333333333333000081, 0.3611111111111000027, 0.3888888888888999973, 0.4166666666666999919, 0.4444444444444000109, 0.4722222222222000054, 0.5000000000000000000, 0.5277777777777999946, 0.5555555555555999891, 0.5833333333333000637, 0.6111111111111000582, 0.6388888888888999418, 0.6666666666667000474, 0.6944444444444000109, 0.7222222222222000054, 0.7500000000000000000, 0.7777777777777999946, 0.8055555555555999891, 0.8333333333333000637, 0.8611111111111000582, 0.8888888888888999418, 0.9166666666667000474, 0.9444444444444000109, 0.9722222222222000054, 1.000000000000000000 ),
 .UNSPECIFIED. ) ;
#5399=CARTESIAN_POINT ( 'NONE',  ( 18.86301435545000871, -0.4770680115090000228, -302.5071922382879279 ) ) ;
#5400=CARTESIAN_POINT ( 'NONE',  ( -11.25912153621000300, -10.42419777155999938, 319.5792614743400009 ) ) ;
#5401=CARTESIAN_POINT ( 'NONE',  ( 17.34500932694999875, -0.6070218422356999932, -314.6383426456000052 ) ) ;
#5402=CARTESIAN_POINT ( 'NONE',  ( -15.43693218238999876, 4.538485726840999490, 314.6383426456000052 ) ) ;
#5404=CARTESIAN_POINT ( 'NONE',  ( 4.927840600415999361, 12.12262669806999149, 318.8802828394900644 ) ) ;
#5409=CARTESIAN_POINT ( 'NONE',  ( 17.40348244433856806, -5.898854237752688690, 315.0000000000000000 ) ) ;
#5410=CARTESIAN_POINT ( 'NONE',  ( -16.84526280568076118, 1.268064982489031545, 315.0000000000000568 ) ) ;
#5411=CARTESIAN_POINT ( 'NONE',  ( -20.00000000032979131, -7.322330470066152230, 190.9999999999999432 ) ) ;
#5413=CARTESIAN_POINT ( 'NONE',  ( -8.647412455283770782, -8.167526177888579042, -315.0000000000000000 ) ) ;
#5414=CARTESIAN_POINT ( 'NONE',  ( 20.00000000000000355, 25.00000000015544543, 191.0000000000000000 ) ) ;
#5417=CARTESIAN_POINT ( 'NONE',  ( 5.334282155825492033, 9.025044196641820449, -314.9999999999999432 ) ) ;
#5418=CARTESIAN_POINT ( 'NONE',  ( -19.10187173594998811, 2.686732971880998910, 189.9229057364800042 ) ) ;
#5419=CARTESIAN_POINT ( 'NONE',  ( 17.50000000000002487, 1.995060298004523415E-08, 314.4999385900306947 ) ) ;
#5426=CARTESIAN_POINT ( 'NONE',  ( 16.95014751240671913, -0.8318069206872660271, 315.0000000000000000 ) ) ;
#5427=CARTESIAN_POINT ( 'NONE',  ( 13.31399140613000043, 6.082710156904999721, -314.8616023057000461 ) ) ;
#5429=CARTESIAN_POINT ( 'NONE',  ( -18.89077695122000122, 0.08689258194099000465, 319.9928079742500131 ) ) ;
#5432=EDGE_LOOP ( 'NONE', ( #1144, #4151, #8847, #9643 ) ) ;
#5433=CARTESIAN_POINT ( 'NONE',  ( 4.911540754813998433, 11.70462039183999892, -317.5770954168139610 ) ) ;
#5434=( BOUNDED_SURFACE ( )  B_SPLINE_SURFACE ( 3, 1, ( 
 ( #436, #8807 ),
 ( #10421, #599 ),
 ( #6391, #9671 ),
 ( #2205, #9618 ),
 ( #3062, #2314 ),
 ( #5525, #1235 ),
 ( #10317, #6228 ) ),
 .UNSPECIFIED., .F., .F., .T. ) 
 B_SPLINE_SURFACE_WITH_KNOTS ( ( 4, 3, 4 ),
 ( 2, 2 ),
 ( 0.006576891565977380054, 0.5000000000000000000, 0.9934231084340230389 ),
 ( 0.000000000000000000, 1.000000000000000000 ),
 .UNSPECIFIED. ) 
 GEOMETRIC_REPRESENTATION_ITEM ( )  RATIONAL_B_SPLINE_SURFACE ( (
 ( 0.9922222087809804414, 0.9922222087809804414),
 ( 0.8003084355045906317, 0.8003084355045906317),
 ( 0.8029010325775971513, 0.8029010325775971513),
 ( 1.000000000000000000, 1.000000000000000000),
 ( 0.8029010325775969292, 0.8029010325775969292),
 ( 0.8003084355045906317, 0.8003084355045906317),
 ( 0.9922222087809811075, 0.9922222087809811075) ) ) 
 REPRESENTATION_ITEM ( '' )  SURFACE ( )  );
#5435=CARTESIAN_POINT ( 'NONE',  ( -1.581094244357999612, -12.05691037822999867, -317.5770954168139610 ) ) ;
#5440=CARTESIAN_POINT ( 'NONE',  ( -16.83327205402999738, 5.309787193942999473, 190.0000000000000000 ) ) ;
#5443=CARTESIAN_POINT ( 'NONE',  ( -12.86685525668169383, 9.583295652123236863, -316.5000000000004547 ) ) ;
#5446=CARTESIAN_POINT ( 'NONE',  ( 19.56025181625999920, 0.5259968871555997794, -302.4229045757450081 ) ) ;
#5451=CARTESIAN_POINT ( 'NONE',  ( 12.29914730983998972, 8.615864166288998760, -302.5071922382879279 ) ) ;
#5452=CARTESIAN_POINT ( 'NONE',  ( 2.571935587102001985, -12.40832180828999398, 318.8802828394900644 ) ) ;
#5454=CARTESIAN_POINT ( 'NONE',  ( -13.31399140613000043, -6.082710156904999721, -314.8616023057000461 ) ) ;
#5459=CARTESIAN_POINT ( 'NONE',  ( -15.00000000000072120, 0.4945770392355430256, 315.0000000000001705 ) ) ;
#5462=CARTESIAN_POINT ( 'NONE',  ( -10.41198510038999991, -7.677033091942000453, 314.8616023057000461 ) ) ;
#5465=CARTESIAN_POINT ( 'NONE',  ( -15.63927740852997950, -6.344868560643003974, 319.9928079742500131 ) ) ;
#5466=CARTESIAN_POINT ( 'NONE',  ( -8.377487131979357571, -8.255758461348163380, -315.0000000000000000 ) ) ;
#5467=CARTESIAN_POINT ( 'NONE',  ( 17.49999999911143433, -5.867334123717693473, 190.0000000000003411 ) ) ;
#5470=CARTESIAN_POINT ( 'NONE',  ( -10.00000000000000000, -2.500000000000000000, -315.0000000000000000 ) ) ;
#5471=EDGE_CURVE ( 'NONE', #2720, #4571, #8628, .T. ) ;
#5473=CARTESIAN_POINT ( 'NONE',  ( 2.737481088004029228, 9.377302004685557080, -315.0000000000000000 ) ) ;
#5474=CARTESIAN_POINT ( 'NONE',  ( -20.06806562977000752, -0.4074806926876002322, 190.4207385301700128 ) ) ;
#5475=CARTESIAN_POINT ( 'NONE',  ( 9.425114110370859777, 8.435515975020026147, 314.4999463140482021 ) ) ;
#5480=CARTESIAN_POINT ( 'NONE',  ( 4.603463306792016319, -9.141632142122212201, 315.0000000000000568 ) ) ;
#5481=CARTESIAN_POINT ( 'NONE',  ( 14.38384290288000145, 5.252906928686999599, -314.8616023057000461 ) ) ;
#5484=CARTESIAN_POINT ( 'NONE',  ( -16.69571944143998365, 6.308604365468005071, 320.0770942683900557 ) ) ;
#5488=CARTESIAN_POINT ( 'NONE',  ( -16.93681971163998057, 6.782628217974004059, -317.0792622552969533 ) ) ;
#5490=CARTESIAN_POINT ( 'NONE',  ( -18.53690224725999514, -4.739426065905003149, -316.3802825947000201 ) ) ;
#5491=CARTESIAN_POINT ( 'NONE',  ( -15.67978886374999803, -4.575336738469999887, -315.0000000000000000 ) ) ;
#5493=CARTESIAN_POINT ( 'NONE',  ( -17.42734739651273301, 0.9144542625322023000, -314.5039539236788073 ) ) ;
#5495=CARTESIAN_POINT ( 'NONE',  ( -16.63787452912266929, -3.035984518719815561, -314.5459997954131950 ) ) ;
#5496=ORIENTED_EDGE ( 'NONE', *, *, #7702, .F. ) ;
#5497=CARTESIAN_POINT ( 'NONE',  ( 14.93376631645305075, 8.332910267862528642, -316.5000000000004547 ) ) ;
#5499=CARTESIAN_POINT ( 'NONE',  ( -4.934712326437797003, -9.087261561615623151, 315.0000000000000000 ) ) ;
#5500=CARTESIAN_POINT ( 'NONE',  ( 12.66297984401999166, -9.215363186789998551, -302.4229045757450081 ) ) ;
#5501=DIRECTION ( 'NONE',  ( 1.000000000000000000, 0.000000000000000000, 0.000000000000000000 ) ) ;
#5503=CARTESIAN_POINT ( 'NONE',  ( -18.21470573400001669, 4.474143576597000127, -302.4229045757450081 ) ) ;
#5507=CARTESIAN_POINT ( 'NONE',  ( 1.409290114754000012, -9.868237606049000021, -314.6383426456000052 ) ) ;
#5508=B_SPLINE_CURVE_WITH_KNOTS ( 'NONE', 1,
 ( #3117, #707 ),
 .UNSPECIFIED., .F., .F.,
 ( 2, 2 ),
 ( 0.01907785912498588185, 0.8020667992272814129 ),
 .UNSPECIFIED. ) ;
#5509=CARTESIAN_POINT ( 'NONE',  ( 11.29198477113000010, 9.236539717938999416, -302.5000000000000000 ) ) ;
#5511=CARTESIAN_POINT ( 'NONE',  ( 19.54676335584001023, -0.8901129224502002391, 189.9229057364800042 ) ) ;
#5515=CARTESIAN_POINT ( 'NONE',  ( -16.78232460783999969, -3.056336161456999712, 314.4150829855000211 ) ) ;
#5517=CARTESIAN_POINT ( 'NONE',  ( 15.68033135863999838, 6.468544937636000469, 320.0000000000000000 ) ) ;
#5518=CARTESIAN_POINT ( 'NONE',  ( -11.73041118561999951, -8.897639792529000502, 319.9928079742500131 ) ) ;
#5519=CARTESIAN_POINT ( 'NONE',  ( -16.35767260765813447, -2.566771890333038542, -315.0000000000000568 ) ) ;
#5524=CARTESIAN_POINT ( 'NONE',  ( 2.614541635441999468, 11.98958966642998902, 189.9229057364800042 ) ) ;
#5525=CARTESIAN_POINT ( 'NONE',  ( -17.49999999911142723, 5.867334123717705907, -302.5000000000003411 ) ) ;
#5531=CARTESIAN_POINT ( 'NONE',  ( -16.84717009645851249, -6.762270094121639374, -303.4999999999996589 ) ) ;
#5532=CARTESIAN_POINT ( 'NONE',  ( 16.75097866579000083, 2.074182492207000461, -314.8616023057000461 ) ) ;
#5534=CARTESIAN_POINT ( 'NONE',  ( -2.538616493050997569, 11.99586634586999523, 320.0770942683900557 ) ) ;
#5538=CARTESIAN_POINT ( 'NONE',  ( -15.01674827698000314, 8.369013993811000418, -317.0792622552969533 ) ) ;
#5539=CARTESIAN_POINT ( 'NONE',  ( 15.95659996325998087, -7.548489772182000124, -316.3802825947000201 ) ) ;
#5542=DIRECTION ( 'NONE',  ( 0.000000000000000000, 0.000000000000000000, 1.000000000000000000 ) ) ;
#5546=CARTESIAN_POINT ( 'NONE',  ( -9.017403168880006703, -8.607149246413708710, -314.5455549245388056 ) ) ;
#5549=CARTESIAN_POINT ( 'NONE',  ( -13.93637444108895096, 8.981144148067276234, -316.5000000000004547 ) ) ;
#5551=CARTESIAN_POINT ( 'NONE',  ( -13.98386538276810498, -5.376986245914816109, 315.0000000000000568 ) ) ;
#5552=CARTESIAN_POINT ( 'NONE',  ( 18.87180507196998747, 0.3567823988189002815, -302.5071922382879279 ) ) ;
#5560=CARTESIAN_POINT ( 'NONE',  ( -10.36918760129999484, 10.25095399663999451, -302.4229045757450081 ) ) ;
#5561=CARTESIAN_POINT ( 'NONE',  ( -9.073652982438993320, -11.14186456285000126, 318.8802828394900644 ) ) ;
#5563=CARTESIAN_POINT ( 'NONE',  ( -10.41198510038999991, -7.677033091942000453, -314.8616023057000461 ) ) ;
#5564=CARTESIAN_POINT ( 'NONE',  ( 19.00000000000000000, 0.000000000000000000, 319.9999999999899956 ) ) ;
#5566=CARTESIAN_POINT ( 'NONE',  ( -19.55151251130001100, -0.8490756357253000930, 189.9229057364800042 ) ) ;
#5567=CARTESIAN_POINT ( 'NONE',  ( -3.129133257132351353, 12.36387889853562960, 190.9999999999996589 ) ) ;
#5573=CARTESIAN_POINT ( 'NONE',  ( -16.77099092997999819, -1.279831385791999843, 315.0848619657999734 ) ) ;
#5575=CARTESIAN_POINT ( 'NONE',  ( -8.531707904373998730, 10.27069628977000093, 320.0000000000000000 ) ) ;
#5576=CARTESIAN_POINT ( 'NONE',  ( 5.823281502584001679, -10.83177932830000501, 319.9928079742500131 ) ) ;
#5577=CARTESIAN_POINT ( 'NONE',  ( -19.99997414083857450, 0.3194320646935535080, 319.0000000000005116 ) ) ;
#5582=CARTESIAN_POINT ( 'NONE',  ( 10.87058130030999159, 10.04705985032000370, 189.9229057364800042 ) ) ;
#5584=EDGE_CURVE ( 'NONE', #1376, #9806, #9840, .T. ) ;
#5586=CARTESIAN_POINT ( 'NONE',  ( 15.52919946924948569, 3.840693445095582081, 314.9999999999999432 ) ) ;
#5588=CARTESIAN_POINT ( 'NONE',  ( 6.533799827619672485, -11.82671337997187599, -303.4999999999996589 ) ) ;
#5589=CARTESIAN_POINT ( 'NONE',  ( -18.86954045039000150, -1.614942466016999978, -302.4999999999529905 ) ) ;
#5591=CARTESIAN_POINT ( 'NONE',  ( -13.67063500649000396, 8.645526204113002322, 320.0770942683900557 ) ) ;
#5596=CARTESIAN_POINT ( 'NONE',  ( -11.58474654271000048, 9.740515853135002899, -317.5770954168139610 ) ) ;
#5606=CARTESIAN_POINT ( 'NONE',  ( 4.393607043691841518, -12.21170385155074989, 319.0000000000003979 ) ) ;
#5610=CARTESIAN_POINT ( 'NONE',  ( -13.64105609808563457, -5.653588212731087026, 315.0000000000000000 ) ) ;
#5611=CARTESIAN_POINT ( 'NONE',  ( -19.57075148197997549, 0.3818783754278996523, -302.4229045757450081 ) ) ;
#5612=ADVANCED_FACE ( 'NONE', ( #2201 ), #6171, .F. ) ;
#5615=CARTESIAN_POINT ( 'NONE',  ( 13.67213454565999875, 8.648884013374997792, -302.4229045757450081 ) ) ;
#5616=LINE ( 'NONE', #10399, #2060 ) ;
#5618=CARTESIAN_POINT ( 'NONE',  ( -8.655660348039997842, -8.816209662726999241, -314.4150829855000211 ) ) ;
#5621=ORIENTED_EDGE ( 'NONE', *, *, #7840, .F. ) ;
#5622=CARTESIAN_POINT ( 'NONE',  ( -2.614541635441999468, -11.98958966642998902, 189.9229057364800042 ) ) ;
#5626=CARTESIAN_POINT ( 'NONE',  ( -15.71297435277999810, -3.490404421959999670, 315.0848619657999734 ) ) ;
#5627=CARTESIAN_POINT ( 'NONE',  ( -11.54587391409000041, 9.118162486329000060, 320.0000000000000000 ) ) ;
#5628=CARTESIAN_POINT ( 'NONE',  ( 0.6117794464027001000, -11.39410369034999704, 319.9928079742500131 ) ) ;
#5633=CARTESIAN_POINT ( 'NONE',  ( -7.006889269069000115, 6.844138725329000472, -285.0000000000000000 ) ) ;
#5634=CARTESIAN_POINT ( 'NONE',  ( -8.887010007670999912, 10.76703833147000822, 189.9229057364800042 ) ) ;
#5638=CARTESIAN_POINT ( 'NONE',  ( -15.67978886374999803, 4.575336738469999887, -315.0000000000000000 ) ) ;
#5639=CARTESIAN_POINT ( 'NONE',  ( -15.26659686508999947, -6.829480052022000258, -302.5000000000000000 ) ) ;
#5642=CARTESIAN_POINT ( 'NONE',  ( 14.08562033053999585, 8.975362299151996126, 319.5792614743400009 ) ) ;
#5645=ORIENTED_EDGE ( 'NONE', *, *, #8567, .F. ) ;
#5646=CARTESIAN_POINT ( 'NONE',  ( 13.88920775975001298, 9.001345760802989204, -316.3802825947000201 ) ) ;
#5650=CARTESIAN_POINT ( 'NONE',  ( 15.63367387165999922, -6.510275065263000371, 320.0000000000000000 ) ) ;
#5656=CARTESIAN_POINT ( 'NONE',  ( -14.90286285339068151, -5.148601615201680026, -314.5782021036098399 ) ) ;
#5657=ORIENTED_EDGE ( 'NONE', *, *, #5731, .F. ) ;
#5658=CARTESIAN_POINT ( 'NONE',  ( -16.88284456999480199, 6.727435487264397551, -316.5000000000004547 ) ) ;
#5660=CARTESIAN_POINT ( 'NONE',  ( -11.93437769929943926, -6.745090416342686801, 315.0000000000000568 ) ) ;
#5661=CARTESIAN_POINT ( 'NONE',  ( 11.71875184657000091, -10.13482718352000944, -303.6197174156509391 ) ) ;
#5667=CARTESIAN_POINT ( 'NONE',  ( 17.77274276690001287, 5.888218767436999457, -302.9207377450070453 ) ) ;
#5668=CARTESIAN_POINT ( 'NONE',  ( 19.95862339310001943, -0.9382979884530006087, 318.8802828394900644 ) ) ;
#5670=CARTESIAN_POINT ( 'NONE',  ( 6.438474686349000997, -8.964777275824999947, -314.8616023057000461 ) ) ;
#5671=CARTESIAN_POINT ( 'NONE',  ( 18.99987386368999864, 0.5560526133780999691, -302.5000000001010108 ) ) ;
#5673=CARTESIAN_POINT ( 'NONE',  ( 16.71231899867997583, -6.291214601299001785, 189.9229057364800042 ) ) ;
#5675=CARTESIAN_POINT ( 'NONE',  ( -12.11078853722071180, 6.646648371397081867, -315.0000000000000000 ) ) ;
#5676=LINE ( 'NONE', #1548, #4989 ) ;
#5678=CARTESIAN_POINT ( 'NONE',  ( -17.11849373668000140, -0.6181952683021000317, 314.8616023057000461 ) ) ;
#5679=ADVANCED_FACE ( 'NONE', ( #2044 ), #9085, .T. ) ;
#5680=CARTESIAN_POINT ( 'NONE',  ( -19.00000000000000000, 0.000000000000000000, 319.9999999999899956 ) ) ;
#5682=CARTESIAN_POINT ( 'NONE',  ( 1.327715439883789150, 12.49239253839650843, 319.0000000000005116 ) ) ;
#5683=CARTESIAN_POINT ( 'NONE',  ( 17.50000000000001776, -8.653793959161173735E-10, 190.0000000000001137 ) ) ;
#5687=ORIENTED_EDGE ( 'NONE', *, *, #6260, .T. ) ;
#5692=CARTESIAN_POINT ( 'NONE',  ( 14.44906369208900365, 4.983045831585199537, 315.0000000000000568 ) ) ;
#5695=CARTESIAN_POINT ( 'NONE',  ( -11.29198477113000010, -9.236539717938999416, -302.5000000000000000 ) ) ;
#5699=CARTESIAN_POINT ( 'NONE',  ( -18.24388381812998361, 5.273776366776003144, 319.5792614743400009 ) ) ;
#5702=CARTESIAN_POINT ( 'NONE',  ( -7.006889269069000115, 6.844138725329000472, -284.9999999999999432 ) ) ;
#5704=CARTESIAN_POINT ( 'NONE',  ( 19.97262988322000865, -0.5553097472237004117, -316.3802825947000201 ) ) ;
#5711=CARTESIAN_POINT ( 'NONE',  ( 14.44867893690424232, -4.983401360453106221, -315.0000000000000000 ) ) ;
#5713=CARTESIAN_POINT ( 'NONE',  ( 1.822666172895148984, -9.956379168149531722, -314.5031572587576534 ) ) ;
#5717=CARTESIAN_POINT ( 'NONE',  ( 10.51805095810000346, -10.63699911018001210, -303.6197174156509391 ) ) ;
#5720=CARTESIAN_POINT ( 'NONE',  ( -3.435942420224999072, 12.40730057411998821, -302.9207377450070453 ) ) ;
#5722=FACE_OUTER_BOUND ( 'NONE', #1969, .T. ) ;
#5723=ORIENTED_EDGE ( 'NONE', *, *, #30, .F. ) ;
#5725=CARTESIAN_POINT ( 'NONE',  ( 6.503149100579999953, 10.80808940222000025, -302.5000000000000000 ) ) ;
#5727=CARTESIAN_POINT ( 'NONE',  ( -12.07524870805000639, -10.05998438363999981, 190.4207385301700128 ) ) ;
#5728=CARTESIAN_POINT ( 'NONE',  ( 13.94567317170587195, 5.407789506212603570, -315.0000000000000000 ) ) ;
#5731=EDGE_CURVE ( 'NONE', #8720, #1105, #297, .T. ) ;
#5732=CARTESIAN_POINT ( 'NONE',  ( 15.10708484062000068, -4.236041382665999500, 315.0848619657999734 ) ) ;
#5735=CARTESIAN_POINT ( 'NONE',  ( 13.67063500649000396, -8.645526204113002322, 320.0770942683900557 ) ) ;
#5737=CARTESIAN_POINT ( 'NONE',  ( -7.927914882803703378, 11.48831374418035089, -303.4999999999990905 ) ) ;
#5740=CARTESIAN_POINT ( 'NONE',  ( -20.00000000435073133, 7.322330466772325686, -303.5000000000000000 ) ) ;
#5747=CARTESIAN_POINT ( 'NONE',  ( 16.45391189178886293, 2.370722300009959760, 315.0000000000001705 ) ) ;
#5749=CARTESIAN_POINT ( 'NONE',  ( 16.78232460783999969, 3.056336161456999712, -314.4150829855000211 ) ) ;
#5754=CARTESIAN_POINT ( 'NONE',  ( 14.79012398733999767, 1.483731117707002278, 315.0000000000001705 ) ) ;
#5756=CARTESIAN_POINT ( 'NONE',  ( 20.05669107747999291, -0.5612988332226998001, -317.0792622552969533 ) ) ;
#5761=CARTESIAN_POINT ( 'NONE',  ( 4.934865307815709201, -9.087242801873950171, -315.0000000000000568 ) ) ;
#5764=CARTESIAN_POINT ( 'NONE',  ( -8.037373804805000077, 9.179324345868998591, -315.0000000000001137 ) ) ;
#5766=CARTESIAN_POINT ( 'NONE',  ( 19.00000000000000000, 0.000000000000000000, -317.4999999998989892 ) ) ;
#5768=CARTESIAN_POINT ( 'NONE',  ( 10.54839116401999988, -10.71567991178000057, -302.9207377450070453 ) ) ;
#5769=CARTESIAN_POINT ( 'NONE',  ( 17.62591998684001027, -4.093640041088997705, -317.4928077629770087 ) ) ;
#5771=CARTESIAN_POINT ( 'NONE',  ( 3.692777996438003196, 12.29248881612998190, -303.6197174156520759 ) ) ;
#5772=CARTESIAN_POINT ( 'NONE',  ( -17.05557420093911958, -2.295407597284876644, 314.4999494796127806 ) ) ;
#5777=CARTESIAN_POINT ( 'NONE',  ( 20.05687582562997662, 0.5621360437329007143, 190.4207385301700128 ) ) ;
#5778=CARTESIAN_POINT ( 'NONE',  ( 0.000000000000000000, -10.54711710274999881, -314.4944826805095772 ) ) ;
#5782=CARTESIAN_POINT ( 'NONE',  ( 16.90798586812000082, 0.2930809059028999797, 315.0848619657999734 ) ) ;
#5784=CARTESIAN_POINT ( 'NONE',  ( -1.310287062331999319, -12.07175205226999815, 320.0770942683900557 ) ) ;
#5787=( NAMED_UNIT ( * ) PLANE_ANGLE_UNIT ( ) SI_UNIT ( $, .RADIAN. ) );
#5788=CARTESIAN_POINT ( 'NONE',  ( 11.89238025184999792, 6.701939844102000166, 315.0848619657999734 ) ) ;
#5790=CARTESIAN_POINT ( 'NONE',  ( -0.7126779659677977552, -12.51265294199207823, 190.9999999999995737 ) ) ;
#5795=B_SPLINE_CURVE_WITH_KNOTS ( 'NONE', 3,
 ( #6505, #1565, #8115, #2477 ),
 .UNSPECIFIED., .F., .F.,
 ( 4, 4 ),
 ( 0.000000000000000000, 1.000000000000000000 ),
 .UNSPECIFIED. ) ;
#5797=CARTESIAN_POINT ( 'NONE',  ( 8.673721998911229747, 8.158754989085133857, 315.0000000000000568 ) ) ;
#5798=CARTESIAN_POINT ( 'NONE',  ( 13.57573464316000056, -3.225916527208000151, -285.0000000000000000 ) ) ;
#5801=CARTESIAN_POINT ( 'NONE',  ( 8.922355960362999383, -10.14988298126000110, -302.5000000000000000 ) ) ;
#5802=CARTESIAN_POINT ( 'NONE',  ( 19.00000000000000000, 0.000000000000000000, 190.0000000000100044 ) ) ;
#5806=CARTESIAN_POINT ( 'NONE',  ( -8.092749801746995431, 11.43508185634000007, -316.3802825947000201 ) ) ;
#5810=CARTESIAN_POINT ( 'NONE',  ( 12.45686666771074336, -6.446195019498007106, -315.0000000000000568 ) ) ;
#5812=CARTESIAN_POINT ( 'NONE',  ( 17.19853431800999743, 2.231396706187000145, -314.4963898845653603 ) ) ;
#5816=CARTESIAN_POINT ( 'NONE',  ( 19.95943119690998557, -1.720147047185998757, -302.9207377450070453 ) ) ;
#5819=CARTESIAN_POINT ( 'NONE',  ( 1.983867121666000877, -11.33269556189999960, -317.4928077629770087 ) ) ;
#5825=CARTESIAN_POINT ( 'NONE',  ( -14.91230748276000817, -5.270530864637949620, 314.4999479601418102 ) ) ;
#5827=CARTESIAN_POINT ( 'NONE',  ( -16.92248268936999978, -0.04189409840124999618, -315.0848619657999734 ) ) ;
#5828=CARTESIAN_POINT ( 'NONE',  ( -4.912752152484999968, 11.11695209346000013, -302.5000000000000000 ) ) ;
#5829=EDGE_LOOP ( 'NONE', ( #10583, #2006 ) ) ;
#5830=CARTESIAN_POINT ( 'NONE',  ( -16.39938580555998726, -7.272241081627004000, 190.4207385301700128 ) ) ;
#5833=CARTESIAN_POINT ( 'NONE',  ( -9.036610176479998202, 11.24204914511999398, 190.4207385301700128 ) ) ;
#5836=CARTESIAN_POINT ( 'NONE',  ( 14.72449281369000040, -5.549439731021000632, 314.4150829855000211 ) ) ;
#5839=CARTESIAN_POINT ( 'NONE',  ( -13.82465948680000878, -8.551125454139995696, 320.0770942683900557 ) ) ;
#5842=CARTESIAN_POINT ( 'NONE',  ( 3.932702496464000497, 9.868769537474999964, 314.4150829855000211 ) ) ;
#5844=CARTESIAN_POINT ( 'NONE',  ( -4.467179684046219457, -12.20122392890712781, 190.9999999999995737 ) ) ;
#5847=CARTESIAN_POINT ( 'NONE',  ( -8.636532331090950976, 8.171139803988637595, 315.0000000000000568 ) ) ;
#5851=CARTESIAN_POINT ( 'NONE',  ( 18.99984306468000028, -0.5551939808346000316, -302.5000000001010108 ) ) ;
#5854=CARTESIAN_POINT ( 'NONE',  ( 12.89381010047549303, -6.798165292128601322, 314.4999421354863784 ) ) ;
#5856=CARTESIAN_POINT ( 'NONE',  ( -17.50000000000000000, 0.000000000000000000, -315.0000000000000000 ) ) ;
#5857=CARTESIAN_POINT ( 'NONE',  ( -10.59417419979999586, 10.60664446758999446, -316.3802825947000201 ) ) ;
#5859=( BOUNDED_CURVE ( )  B_SPLINE_CURVE ( 3, ( #6279, #8801, #1443, #2850, #6118, #7409, #746, #8911, #1612, #8163, #10578, #9775, #800, #6440, #6383, #644, #8105, #6550, #3324, #4833, #9664, #3969, #2306, #5682, #9024, #4885, #3272, #3221, #9885, #8970, #1660, #9077, #10467, #4080, #10519, #7357, #4026, #1501, #2521, #7197, #4935, #6497, #3887, #8859, #9830, #849, #5577, #4783 ),
 .UNSPECIFIED., .F., .F. ) 
 B_SPLINE_CURVE_WITH_KNOTS ( ( 4, 1, 1, 1, 1, 1, 1, 1, 1, 1, 1, 1, 1, 1, 1, 1, 1, 1, 1, 1, 1, 1, 1, 1, 1, 1, 1, 1, 1, 1, 1, 1, 1, 1, 1, 1, 1, 1, 1, 1, 1, 1, 1, 1, 1, 4 ),
 ( 0.000000000000000000, 0.01696016684112893608, 0.03526043942249617452, 0.05280277254187633329, 0.06993090526874494450, 0.08694163804313655153, 0.1040119350351718791, 0.1210139405588612077, 0.1379792171159073266, 0.1553986424958141432, 0.1736039501722523581, 0.1924119339504005155, 0.2116998327295476212, 0.2316504953696777447, 0.2523434511079294396, 0.2735071578860148178, 0.2951461022590913807, 0.3179819391660331784, 0.3428270683969385502, 0.3704763703089109517, 0.4013842106079446026, 0.4356267894623514492, 0.4731822280981956563, 0.5126799690798770071, 0.5516183454030081368, 0.5879427231221452388, 0.6209690717414464434, 0.6502633940987107009, 0.6759717312850140880, 0.6991685419836423110, 0.7210175260783883155, 0.7426211155567139510, 0.7640811388048154296, 0.7847659435495429880, 0.8046277674085309251, 0.8239473966552023354, 0.8426767883169220541, 0.8606205966378887018, 0.8779797588928680563, 0.8951189492511467671, 0.9121717320952801300, 0.9291919606104407370, 0.9463734364297033963, 0.9639783248497096890, 0.9823161612921426089, 1.000000000000000000 ),
 .UNSPECIFIED. ) 
 CURVE ( )  GEOMETRIC_REPRESENTATION_ITEM ( )  RATIONAL_B_SPLINE_CURVE ( ( 1.171573005652621013, 1.171573005652621235, 1.171573005652621235, 1.171573005652621235, 1.171573005652621235, 1.171573005652621235, 1.171573005652621235, 1.171573005652621235, 1.171573005652621235, 1.171573005652621235, 1.171573005652621235, 1.171573005652621235, 1.171573005652621235, 1.171573005652621235, 1.171573005652621235, 1.171573005652621235, 1.171573005652621235, 1.171573005652621235, 1.171573005652621235, 1.171573005652621235, 1.171573005652621235, 1.171573005652621235, 1.171573005652621235, 1.171573005652621235, 1.171573005652621235, 1.171573005652621235, 1.171573005652621235, 1.171573005652621235, 1.171573005652621235, 1.171573005652621235, 1.171573005652621235, 1.171573005652621235, 1.171573005652621235, 1.171573005652621235, 1.171573005652621235, 1.171573005652621235, 1.171573005652621235, 1.171573005652621235, 1.171573005652621235, 1.171573005652621235, 1.171573005652621235, 1.171573005652621235, 1.171573005652621235, 1.171573005652621235, 1.171573005652621235, 1.171573005652621235, 1.171573005652621235, 1.171573005652621235 ) ) 
 REPRESENTATION_ITEM ( '' )  );
#5863=CARTESIAN_POINT ( 'NONE',  ( 4.669917308725584526, -9.131001784561973977, -315.0000000000000000 ) ) ;
#5865=CARTESIAN_POINT ( 'NONE',  ( -17.50000000000125056, -1.380497925828168986E-12, -315.0000000000001705 ) ) ;
#5869=CARTESIAN_POINT ( 'NONE',  ( -13.88537659940002023, -9.003549035645995957, -303.6197174156509391 ) ) ;
#5870=B_SPLINE_CURVE_WITH_KNOTS ( 'NONE', 3,
 ( #3727, #9529, #1412, #5491, #3776, #10283, #8770, #7807, #1357, #4639, #5280, #2922, #3673 ),
 .UNSPECIFIED., .F., .F.,
 ( 4, 1, 1, 1, 1, 1, 1, 1, 1, 1, 4 ),
 ( 0.000000000000000000, 0.08333333333333001192, 0.1666666666667000196, 0.2500000000000000000, 0.3333333333333000081, 0.5000000000000000000, 0.6666666666667000474, 0.7500000000000000000, 0.8333333333333000637, 0.9166666666667000474, 1.000000000000000000 ),
 .UNSPECIFIED. ) ;
#5872=CARTESIAN_POINT ( 'NONE',  ( -18.90056365643000547, -0.3167749459464000994, -317.4928077629770087 ) ) ;
#5873=CARTESIAN_POINT ( 'NONE',  ( -16.76545246634000108, 2.037063237379999947, -314.8616023057000461 ) ) ;
#5875=CARTESIAN_POINT ( 'NONE',  ( 19.97256092624000701, -0.5562539513971997973, -303.6197174156509391 ) ) ;
#5876=CARTESIAN_POINT ( 'NONE',  ( -17.49999996772987743, -5.857864456328762515, 314.9999999999999432 ) ) ;
#5879=EDGE_CURVE ( 'NONE', #3758, #6759, #5172, .T. ) ;
#5882=CARTESIAN_POINT ( 'NONE',  ( 17.06589079541999965, -6.642208448352997507, 190.4207385301700128 ) ) ;
#5883=CARTESIAN_POINT ( 'NONE',  ( 15.67978886374999803, -4.575336738469999887, -315.0000000000001137 ) ) ;
#5884=CARTESIAN_POINT ( 'NONE',  ( 16.35767260765813447, 2.566771890333039874, -315.0000000000000000 ) ) ;
#5887=CARTESIAN_POINT ( 'NONE',  ( 8.858368459239001069, 11.29793033041000250, 190.4207385301700128 ) ) ;
#5889=CARTESIAN_POINT ( 'NONE',  ( 14.57772014836000096, -5.380605385836000565, 314.6383426456000052 ) ) ;
#5892=CARTESIAN_POINT ( 'NONE',  ( 12.76583521038999613, -9.157751700393998107, 320.0770942683900557 ) ) ;
#5894=CARTESIAN_POINT ( 'NONE',  ( 0.1638132020714604398, 12.51773231663031716, -303.4999999999990905 ) ) ;
#5895=CARTESIAN_POINT ( 'NONE',  ( 8.655660348039997842, 8.816209662726999241, 314.4150829855000211 ) ) ;
#5896=EDGE_LOOP ( 'NONE', ( #1700, #2391 ) ) ;
#5897=CARTESIAN_POINT ( 'NONE',  ( 6.404755722164563458, -11.85477825286778319, 190.9999999999995737 ) ) ;
#5898=CARTESIAN_POINT ( 'NONE',  ( 19.58476356052999279, 2.818858455686998887, 319.5792614743400009 ) ) ;
#5905=CARTESIAN_POINT ( 'NONE',  ( -1.962900534989000745, 9.435972684515721909, 314.9999999999999432 ) ) ;
#5906=VECTOR ( 'NONE', #747, 1000.000000000000000 ) ;
#5907=CARTESIAN_POINT ( 'NONE',  ( -15.00000000000325784, 8.632726818195413123E-17, 315.0000000000001705 ) ) ;
#5910=CARTESIAN_POINT ( 'NONE',  ( 4.912752152484999968, -11.11695209346000013, -302.5000000000000000 ) ) ;
#5913=CARTESIAN_POINT ( 'NONE',  ( 5.950428891765999317, 10.92854977363000124, 190.0000000000000000 ) ) ;
#5922=CARTESIAN_POINT ( 'NONE',  ( 10.00000000000000000, 2.500000000000000000, -315.0000000000000000 ) ) ;
#5923=CARTESIAN_POINT ( 'NONE',  ( 9.142617743994909674, -7.997268146336696581, -315.0000000000000568 ) ) ;
#5928=CARTESIAN_POINT ( 'NONE',  ( -18.87000901094000227, 1.611639242563999819, -317.5000000000470095 ) ) ;
#5930=CARTESIAN_POINT ( 'NONE',  ( 16.06911929583999310, 5.954958506906000260, -317.4928077629770087 ) ) ;
#5933=CARTESIAN_POINT ( 'NONE',  ( -17.60469080286000931, -4.126100741655001514, -317.4928077629770087 ) ) ;
#5934=CARTESIAN_POINT ( 'NONE',  ( -17.59298685096999648, 0.02218567204014999794, -314.4150829855000211 ) ) ;
#5939=CARTESIAN_POINT ( 'NONE',  ( 15.91674550148000122, 7.581266318323002906, -303.6197174156520759 ) ) ;
#5940=CARTESIAN_POINT ( 'NONE',  ( -17.44863594367627613, -0.8973220716409442410, 314.4999502393482089 ) ) ;
#5942=CARTESIAN_POINT ( 'NONE',  ( -17.11849373668000140, -0.6181952683021000317, -314.8616023057000461 ) ) ;
#5946=CARTESIAN_POINT ( 'NONE',  ( 19.85617711436999144, -1.942822351932998792, 190.4207385301700128 ) ) ;
#5949=CARTESIAN_POINT ( 'NONE',  ( -19.77421425755001039, 1.922351829117000976, 191.1197171614399792 ) ) ;
#5950=CARTESIAN_POINT ( 'NONE',  ( 15.27200851150000105, -4.387263554753999983, 314.8616023057000461 ) ) ;
#5953=CARTESIAN_POINT ( 'NONE',  ( 18.32873049326003212, -4.258249849688001909, 320.0770942683900557 ) ) ;
#5955=CARTESIAN_POINT ( 'NONE',  ( 17.71378747801019315, 5.838323448755804002, -303.5000000000000000 ) ) ;
#5956=CARTESIAN_POINT ( 'NONE',  ( 16.78232460783999969, 3.056336161456999712, 314.4150829855000211 ) ) ;
#5959=CARTESIAN_POINT ( 'NONE',  ( 7.868470208275999411, 11.58296045169998401, 319.5792614743400009 ) ) ;
#5960=DIRECTION ( 'NONE',  ( 3.596898303937126455E-07, 0.9999999999999354960, -1.203273141451894460E-22 ) ) ;
#5962=CARTESIAN_POINT ( 'NONE',  ( 11.28384026436728327, 7.096146896414363248, 315.0000000000000000 ) ) ;
#5966=CARTESIAN_POINT ( 'NONE',  ( 15.00000000000326139, -5.136019918588313243E-17, 315.0000000000001137 ) ) ;
#5968=CARTESIAN_POINT ( 'NONE',  ( 16.24773438692637839, -3.756014664266052350, 314.4999406160053468 ) ) ;
#5969=CARTESIAN_POINT ( 'NONE',  ( 18.45932313982999062, 2.405278989253002209, 190.0071920248299477 ) ) ;
#5975=EDGE_LOOP ( 'NONE', ( #300, #10291, #5226, #6483 ) ) ;
#5976=CARTESIAN_POINT ( 'NONE',  ( 16.80239380511999059, 5.162410948549997158, 319.9928079742500131 ) ) ;
#5981=CARTESIAN_POINT ( 'NONE',  ( -15.24853452200002302, 6.688806263293003873, -317.4928077629770087 ) ) ;
#5982=CARTESIAN_POINT ( 'NONE',  ( 15.24853452200002302, -6.688806263293003873, -317.4928077629770087 ) ) ;
#5983=CARTESIAN_POINT ( 'NONE',  ( -17.56954514911999965, -0.4333932196220000033, -314.4150829855000211 ) ) ;
#5987=CARTESIAN_POINT ( 'NONE',  ( 3.134365345935000047, -11.35765845234000082, 190.0000000000000000 ) ) ;
#5990=DIRECTION ( 'NONE',  ( 5.235554895604999868E-10, 4.130578887848000029E-10, 1.000000000000000000 ) ) ;
#5995=CARTESIAN_POINT ( 'NONE',  ( 4.866278641173998665, -11.00354869785000211, -302.5071922382879279 ) ) ;
#5996=CARTESIAN_POINT ( 'NONE',  ( -16.34052447997000357, 7.211013068275999416, 191.1197171614399792 ) ) ;
#6000=CARTESIAN_POINT ( 'NONE',  ( 4.404324556173000005, -12.28809208595000335, 319.5792614743400009 ) ) ;
#6002=CARTESIAN_POINT ( 'NONE',  ( 17.14577796628000073, -0.02050488658304999712, -314.8616023057000461 ) ) ;
#6003=CARTESIAN_POINT ( 'NONE',  ( 15.07109120124999890, 4.275483045295999318, 315.0848619657999734 ) ) ;
#6004=EDGE_LOOP ( 'NONE', ( #9156, #3997, #6373, #2289, #3314 ) ) ;
#6006=CARTESIAN_POINT ( 'NONE',  ( 17.10170768143997932, 6.605950023609995725, 319.5792614743400009 ) ) ;
#6008=EDGE_CURVE ( 'NONE', #10392, #1085, #4692, .T. ) ;
#6011=CARTESIAN_POINT ( 'NONE',  ( -8.096811247556559010, 8.344189070382460827, 315.0000000000001137 ) ) ;
#6015=FACE_BOUND ( 'NONE', #5975, .T. ) ;
#6016=CARTESIAN_POINT ( 'NONE',  ( 18.99997815069999874, 0.3119984768183999835, 190.0000000000100044 ) ) ;
#6018=CARTESIAN_POINT ( 'NONE',  ( 6.176507221981585971, -9.366274586590517259, 314.4999436549671259 ) ) ;
#6019=CARTESIAN_POINT ( 'NONE',  ( 16.23266328071998643, 5.782092517776998619, 190.0071920248299477 ) ) ;
#6028=CARTESIAN_POINT ( 'NONE',  ( 18.86318716375000193, -0.4770217013004998119, 319.9928079742500131 ) ) ;
#6032=CARTESIAN_POINT ( 'NONE',  ( -1.983867121666000877, 11.33269556189999960, -317.4928077629770087 ) ) ;
#6033=CARTESIAN_POINT ( 'NONE',  ( 2.028805552265000589, -12.03060078454999449, -317.5770954168139610 ) ) ;
#6037=CARTESIAN_POINT ( 'NONE',  ( -15.43693218238999876, 4.538485726840999490, -314.6383426456000052 ) ) ;
#6038=CARTESIAN_POINT ( 'NONE',  ( 11.52006393673606865, 7.476351274249532608, -314.5677505184611391 ) ) ;
#6039=CARTESIAN_POINT ( 'NONE',  ( 17.49922277440664686, -0.09424638433143421590, 314.4999507458385892 ) ) ;
#6041=CARTESIAN_POINT ( 'NONE',  ( 17.80781204382000027, -3.997739559166000323, 190.0000000000000000 ) ) ;
#6044=CARTESIAN_POINT ( 'NONE',  ( -20.00478054794001537, -0.07382975964156003601, 191.1197171614399792 ) ) ;
#6045=EDGE_LOOP ( 'NONE', ( #3358, #3085 ) ) ;
#6048=CARTESIAN_POINT ( 'NONE',  ( 19.97288175887001316, -0.5556452136295997324, 191.1197171614399792 ) ) ;
#6055=CARTESIAN_POINT ( 'NONE',  ( -17.71262672283002360, -5.941112223585997221, 319.5792614743400009 ) ) ;
#6056=FACE_OUTER_BOUND ( 'NONE', #1471, .T. ) ;
#6057=CARTESIAN_POINT ( 'NONE',  ( -15.74033075358999945, 3.452242816619000010, 315.0848619657999734 ) ) ;
#6061=CARTESIAN_POINT ( 'NONE',  ( -10.97158218462999457, 10.45285060525999121, 318.8802828394900644 ) ) ;
#6062=B_SPLINE_SURFACE_WITH_KNOTS ( 'NONE', 3, 3, ( 
 ( #5071, #7497, #9165, #5983 ),
 ( #139, #1043, #9327, #4329 ),
 ( #10024, #9380, #7656, #5934 ),
 ( #8352, #9277, #8508, #296 ),
 ( #3414, #9224, #7704, #7602 ),
 ( #4278, #5873, #2014, #5182 ),
 ( #2611, #249, #3526, #6803 ),
 ( #990, #348, #10076, #8455 ),
 ( #1095, #10124, #6037, #1961 ),
 ( #1296, #3662, #10165, #6952 ),
 ( #1347, #6131, #6898, #4576 ),
 ( #5319, #5269, #2808, #7004 ),
 ( #10226, #7850, #10276, #2861 ),
 ( #497, #7901, #3765, #2161 ),
 ( #8761, #7058, #546, #7960 ),
 ( #10322, #1242, #2913, #3616 ),
 ( #1401, #6081, #3822, #2964 ),
 ( #4685, #2212, #6181, #6235 ),
 ( #2106, #2005, #9371, #8544 ),
 ( #4518, #7797, #1187, #8653 ),
 ( #10376, #9465, #7745, #9522 ),
 ( #4630, #3016, #4466, #9418 ),
 ( #7107, #388, #2054, #8593 ),
 ( #443, #5427, #8703, #6290 ),
 ( #9574, #5481, #3718, #5372 ),
 ( #4844, #6400, #10589, #8014 ),
 ( #6561, #9843, #2265, #7264 ),
 ( #756, #3981, #6, #5749 ),
 ( #2321, #5532, #7157, #10536 ),
 ( #2480, #710, #8815, #8983 ),
 ( #3179, #6453, #1623, #10478 ),
 ( #9034, #8118, #4894, #4945 ),
 ( #4041, #8872, #9733, #607 ),
 ( #1672, #3068, #808, #7319 ) ),
 .UNSPECIFIED., .F., .F., .F.,
 ( 4, 1, 1, 1, 1, 1, 1, 1, 1, 1, 1, 1, 1, 1, 1, 1, 1, 1, 1, 1, 1, 1, 1, 1, 1, 1, 1, 1, 1, 1, 1, 4 ),
 ( 4, 4 ),
 ( -0.01402646298304000005, 0.000000000000000000, 0.03448275862069000164, 0.06896551724138000328, 0.1034482758621000087, 0.1379310344828000023, 0.1724137931033999926, 0.2068965517240999863, 0.2413793103448000077, 0.2758620689655000291, 0.3103448275861999672, 0.3448275862069000164, 0.3793103448276000100, 0.4137931034483000037, 0.4482758620689999973, 0.4827586206897000465, 0.5172413793103000090, 0.5517241379310000582, 0.5862068965516999963, 0.6206896551723999345, 0.6551724137930999836, 0.6896551724138000328, 0.7241379310344999709, 0.7586206896552000201, 0.7931034482758999582, 0.8275862068966000074, 0.8620689655171999144, 0.8965517241379000746, 0.9310344827586000127, 0.9655172413793000619, 1.000000000000000000, 1.015741306098000063 ),
 ( -0.1697239316932999953, 1.169834029081999960 ),
 .UNSPECIFIED. ) ;
#6065=CARTESIAN_POINT ( 'NONE',  ( -16.25530297147532721, 2.761162301196854685, 315.0000000000000000 ) ) ;
#6066=CARTESIAN_POINT ( 'NONE',  ( 15.00000000000072120, -0.4945770392355430256, 315.0000000000001705 ) ) ;
#6067=CARTESIAN_POINT ( 'NONE',  ( 17.50000000000000000, 0.000000000000000000, -315.0000000000000000 ) ) ;
#6068=ADVANCED_FACE ( 'NONE', ( #9548 ), #6628, .T. ) ;
#6073=CARTESIAN_POINT ( 'NONE',  ( -16.91992689674541950, 1.077645906677548115, -315.0000000000000000 ) ) ;
#6074=CARTESIAN_POINT ( 'NONE',  ( 0.6878067384150999830, 11.39249343872000075, 190.0071920248299477 ) ) ;
#6077=CARTESIAN_POINT ( 'NONE',  ( 13.36995595564000006, -8.154012700520999246, -317.5000000000000000 ) ) ;
#6080=CARTESIAN_POINT ( 'NONE',  ( 5.334308159457383347, -9.025045582129868293, 314.9999999999999432 ) ) ;
#6081=CARTESIAN_POINT ( 'NONE',  ( -1.399029207469000058, 9.644928263550999858, -314.8616023057000461 ) ) ;
#6083=ORIENTED_EDGE ( 'NONE', *, *, #7787, .F. ) ;
#6084=CARTESIAN_POINT ( 'NONE',  ( 18.87181153733000016, -0.3572136203155001355, 319.9928079742500131 ) ) ;
#6085=CARTESIAN_POINT ( 'NONE',  ( 17.74479464825532204, -5.801447790587960895, -316.5000000000004547 ) ) ;
#6089=STYLED_ITEM ( 'NONE', ( #6605 ), #5170 ) ;
#6092=CARTESIAN_POINT ( 'NONE',  ( 10.62478234909000285, -10.68521885564000051, -317.0792622552969533 ) ) ;
#6099=CARTESIAN_POINT ( 'NONE',  ( -9.971838575284008854, -10.83713921150001447, 191.1197171614399792 ) ) ;
#6101=CARTESIAN_POINT ( 'NONE',  ( -16.37177374402162400, -2.538919766875962658, 314.9999999999999432 ) ) ;
#6102=CARTESIAN_POINT ( 'NONE',  ( -12.29914730983998972, -8.615864166288998760, -302.5071922382879279 ) ) ;
#6103=CARTESIAN_POINT ( 'NONE',  ( 19.98293839508998104, -0.4162045188173000287, 191.1197171614399792 ) ) ;
#6106=CARTESIAN_POINT ( 'NONE',  ( 13.31171245337000819, 8.049428572247000702, -302.5071922382879279 ) ) ;
#6107=CARTESIAN_POINT ( 'NONE',  ( 20.04253597850999569, -0.9484392003694999129, 319.5792614743400009 ) ) ;
#6108=CARTESIAN_POINT ( 'NONE',  ( 17.21448334449999962, -1.351716521078000222, -314.6383426456000052 ) ) ;
#6109=CARTESIAN_POINT ( 'NONE',  ( -16.76545246634000108, 2.037063237379999947, 314.8616023057000461 ) ) ;
#6111=CARTESIAN_POINT ( 'NONE',  ( 16.21588929933999523, -5.798404451932999137, 190.0071920248299477 ) ) ;
#6112=CARTESIAN_POINT ( 'NONE',  ( -7.493827757249003518, 11.59400354817999457, 318.8802828394900644 ) ) ;
#6113=CARTESIAN_POINT ( 'NONE',  ( -15.00000000000000000, 0.000000000000000000, -285.0000000000000000 ) ) ;
#6117=CARTESIAN_POINT ( 'NONE',  ( -2.814980436929585108E-10, -12.50000000000000000, 319.0000000000000000 ) ) ;
#6118=CARTESIAN_POINT ( 'NONE',  ( 19.51225877040622692, 2.792229942217316463, 319.0000000000005116 ) ) ;
#6122=CARTESIAN_POINT ( 'NONE',  ( -5.242074483217283642, 9.033702059254421712, -315.0000000000000000 ) ) ;
#6123=CARTESIAN_POINT ( 'NONE',  ( 4.308829118669001979, 11.09213725138999962, 190.0071920248299477 ) ) ;
#6130=CARTESIAN_POINT ( 'NONE',  ( 1.962900534989000745, -9.435972684515721909, 314.9999999999999432 ) ) ;
#6131=CARTESIAN_POINT ( 'NONE',  ( -13.37260572687999982, 6.041714840053000302, -314.8616023057000461 ) ) ;
#6134=CARTESIAN_POINT ( 'NONE',  ( 18.89057790499001754, 0.06397434778252002185, 319.9928079742500131 ) ) ;
#6135=CARTESIAN_POINT ( 'NONE',  ( -17.71658133615935427, -5.834976589818515080, -316.5000000000004547 ) ) ;
#6137=ORIENTED_EDGE ( 'NONE', *, *, #7510, .F. ) ;
#6138=CARTESIAN_POINT ( 'NONE',  ( 17.49999999954662044, -9.625715914672042649E-06, 190.0000000000000000 ) ) ;
#6139=CARTESIAN_POINT ( 'NONE',  ( 8.115185848843001537, -11.51636271397001465, -317.0792622552969533 ) ) ;
#6141=EDGE_CURVE ( 'NONE', #9430, #2509, #1482, .T. ) ;
#6144=CARTESIAN_POINT ( 'NONE',  ( 17.34597251029000375, -4.674348096672999553, 190.0000000000000000 ) ) ;
#6145=CARTESIAN_POINT ( 'NONE',  ( -10.23467949917770525, -9.999999999493892844, 189.9999999999997726 ) ) ;
#6147=CARTESIAN_POINT ( 'NONE',  ( 1.248913580286000302, -12.48838264809999643, 191.1197171614399792 ) ) ;
#6150=CARTESIAN_POINT ( 'NONE',  ( 3.306880204566999382, -11.21686954173999951, -302.5071922382879279 ) ) ;
#6155=CARTESIAN_POINT ( 'NONE',  ( 14.79708307774000353, -8.514882941861998233, 319.5792614743400009 ) ) ;
#6156=CARTESIAN_POINT ( 'NONE',  ( 16.28527389671999970, -3.844447514156999812, -314.4150829855000211 ) ) ;
#6157=CARTESIAN_POINT ( 'NONE',  ( -17.12243801299000268, 0.5826713957640000663, 314.8616023057000461 ) ) ;
#6158=ORIENTED_EDGE ( 'NONE', *, *, #2869, .T. ) ;
#6159=CARTESIAN_POINT ( 'NONE',  ( 15.60334176867001688, -6.376785739494004623, 190.0071920248299477 ) ) ;
#6166=CARTESIAN_POINT ( 'NONE',  ( 0.000000000000000000, -7.937240849781000307, 315.0000000000001705 ) ) ;
#6169=CARTESIAN_POINT ( 'NONE',  ( -20.00000000000000000, -7.771159141713679452E-11, 319.0000000000000000 ) ) ;
#6171=PLANE ( 'NONE',  #719 ) ;
#6172=CARTESIAN_POINT ( 'NONE',  ( -8.666289393444031930, 8.161235200486094854, -315.0000000000000000 ) ) ;
#6175=VECTOR ( 'NONE', #7353, 1000.000000000000000 ) ;
#6178=CARTESIAN_POINT ( 'NONE',  ( 11.32071836301000012, -9.223563301002998926, -317.5000000000000000 ) ) ;
#6180=CARTESIAN_POINT ( 'NONE',  ( 16.34899991413091414, -2.583752171356570759, 315.0000000000000000 ) ) ;
#6181=CARTESIAN_POINT ( 'NONE',  ( 1.276003512426000075, 9.874146089817999794, -314.6383426456000052 ) ) ;
#6182=CARTESIAN_POINT ( 'NONE',  ( -17.50000000000125056, -1.380497925828168986E-12, -314.4963898845654171 ) ) ;
#6186=CARTESIAN_POINT ( 'NONE',  ( -16.58827648083000028, 6.426222433883002516, -317.5770954168139610 ) ) ;
#6187=( BOUNDED_SURFACE ( )  B_SPLINE_SURFACE ( 3, 3, ( 
 ( #1693, #8243, #2503, #3301, #7496, #5769, #5179, #7548, #5982, #9276, #5016, #3363, #3467, #193, #28, #6639, #9057, #4968, #84, #5819, #7599, #4220, #935, #2553, #8294, #9112, #4381, #137, #1092, #3413, #6749, #9968, #10023, #4166, #2665, #5933, #2716, #2609, #5872, #9223, #1855 ),
 ( #10075, #9163, #1908, #247, #5125, #1746, #8402, #1042, #1802, #5070, #8453, #3525, #8351, #6583, #989, #4276, #4328, #6802, #9866, #6033, #7703, #5435, #7805, #2062, #9325, #9426, #4525, #1147, #9528, #8712, #2114, #347, #6188, #7065, #3773, #1959, #5230, #10123, #294, #4473, #2764 ),
 ( #2971, #6242, #2012, #3625, #450, #3725, #7654, #6905, #8506, #4426, #10173, #2816, #4583, #6092, #7859, #6139, #9378, #5326, #5278, #8552, #1249, #9473, #7011, #1355, #2168, #3572, #1196, #10330, #504, #10282, #7752, #2920, #395, #3668, #6961, #10235, #6853, #5380, #2868, #8601, #8661 ),
 ( #1304, #8824, #1409, #6297, #4750, #717, #1469, #4854, #5539, #8129, #2273, #8020, #614, #2221, #6515, #8879, #10543, #10597, #663, #3939, #3990, #4693, #7164, #3888, #10435, #553, #6460, #7115, #9798, #3187, #10383, #9582, #4638, #7220, #7968, #5490, #10487, #7272, #3129, #766, #6407 ) ),
 .UNSPECIFIED., .F., .F., .F. ) 
 B_SPLINE_SURFACE_WITH_KNOTS ( ( 4, 4 ),
 ( 4, 1, 1, 1, 1, 1, 1, 1, 1, 1, 1, 1, 1, 1, 1, 1, 1, 1, 1, 1, 1, 1, 1, 1, 1, 1, 1, 1, 1, 1, 1, 1, 1, 1, 1, 1, 1, 1, 4 ),
 ( 0.000000000000000000, 1.000000000000000000 ),
 ( -0.007738640450445999699, 0.000000000000000000, 0.03414709649185000001, 0.06696605908318999101, 0.09596079224771000837, 0.1211002772268999911, 0.1443783404606999998, 0.1680876537897000034, 0.1921286104184000143, 0.2160216200219000071, 0.2397245863996999848, 0.2634813019505999887, 0.2879188160025000220, 0.3133917475886000004, 0.3395543376315999784, 0.3663618195672999622, 0.3946229251345000355, 0.4252536485549999745, 0.4591139563344999730, 0.4956048897295999844, 0.5324779435423999674, 0.5674158629142000976, 0.5992726300609999557, 0.6287198090143000240, 0.6565915576515000129, 0.6836661054489000522, 0.7100337132233999204, 0.7353920520230999847, 0.7598724402797999433, 0.7838392479475999597, 0.8076909583479000565, 0.8317349054331000247, 0.8555088018188000687, 0.8788217029082999732, 0.9039691640437000908, 0.9329692239710999369, 0.9658153655582000230, 1.000000000000000000, 1.008464120473999914 ),
 .UNSPECIFIED. ) 
 GEOMETRIC_REPRESENTATION_ITEM ( )  RATIONAL_B_SPLINE_SURFACE ( (
 ( 1.236577356246000070, 1.236577356246000070, 1.236577356246000070, 1.236577356246000070, 1.236577356246000070, 1.236577356246000070, 1.236577356246000070, 1.236577356246000070, 1.236577356246000070, 1.236577356246000070, 1.236577356246000070, 1.236577356246000070, 1.236577356246000070, 1.236577356246000070, 1.236577356246000070, 1.236577356246000070, 1.236577356246000070, 1.236577356246000070, 1.236577356246000070, 1.236577356246000070, 1.236577356246000070, 1.236577356246000070, 1.236577356246000070, 1.236577356246000070, 1.236577356246000070, 1.236577356246000070, 1.236577356246000070, 1.236577356246000070, 1.236577356246000070, 1.236577356246000070, 1.236577356246000070, 1.236577356246000070, 1.236577356246000070, 1.236577356246000070, 1.236577356246000070, 1.236577356246000070, 1.236577356246000070, 1.236577356246000070, 1.236577356246000070, 1.236577356246000070, 1.236577356246000070),
 ( 0.9211408812511999722, 0.9211408812511999722, 0.9211408812511999722, 0.9211408812511999722, 0.9211408812511999722, 0.9211408812511999722, 0.9211408812511999722, 0.9211408812511999722, 0.9211408812511999722, 0.9211408812511999722, 0.9211408812511999722, 0.9211408812511999722, 0.9211408812511999722, 0.9211408812511999722, 0.9211408812511999722, 0.9211408812511999722, 0.9211408812511999722, 0.9211408812511999722, 0.9211408812511999722, 0.9211408812511999722, 0.9211408812511999722, 0.9211408812511999722, 0.9211408812511999722, 0.9211408812511999722, 0.9211408812511999722, 0.9211408812511999722, 0.9211408812511999722, 0.9211408812511999722, 0.9211408812511999722, 0.9211408812511999722, 0.9211408812511999722, 0.9211408812511999722, 0.9211408812511999722, 0.9211408812511999722, 0.9211408812511999722, 0.9211408812511999722, 0.9211408812511999722, 0.9211408812511999722, 0.9211408812511999722, 0.9211408812511999722, 0.9211408812511999722),
 ( 0.9211408812511999722, 0.9211408812511999722, 0.9211408812511999722, 0.9211408812511999722, 0.9211408812511999722, 0.9211408812511999722, 0.9211408812511999722, 0.9211408812511999722, 0.9211408812511999722, 0.9211408812511999722, 0.9211408812511999722, 0.9211408812511999722, 0.9211408812511999722, 0.9211408812511999722, 0.9211408812511999722, 0.9211408812511999722, 0.9211408812511999722, 0.9211408812511999722, 0.9211408812511999722, 0.9211408812511999722, 0.9211408812511999722, 0.9211408812511999722, 0.9211408812511999722, 0.9211408812511999722, 0.9211408812511999722, 0.9211408812511999722, 0.9211408812511999722, 0.9211408812511999722, 0.9211408812511999722, 0.9211408812511999722, 0.9211408812511999722, 0.9211408812511999722, 0.9211408812511999722, 0.9211408812511999722, 0.9211408812511999722, 0.9211408812511999722, 0.9211408812511999722, 0.9211408812511999722, 0.9211408812511999722, 0.9211408812511999722, 0.9211408812511999722),
 ( 1.236577356246000070, 1.236577356246000070, 1.236577356246000070, 1.236577356246000070, 1.236577356246000070, 1.236577356246000070, 1.236577356246000070, 1.236577356246000070, 1.236577356246000070, 1.236577356246000070, 1.236577356246000070, 1.236577356246000070, 1.236577356246000070, 1.236577356246000070, 1.236577356246000070, 1.236577356246000070, 1.236577356246000070, 1.236577356246000070, 1.236577356246000070, 1.236577356246000070, 1.236577356246000070, 1.236577356246000070, 1.236577356246000070, 1.236577356246000070, 1.236577356246000070, 1.236577356246000070, 1.236577356246000070, 1.236577356246000070, 1.236577356246000070, 1.236577356246000070, 1.236577356246000070, 1.236577356246000070, 1.236577356246000070, 1.236577356246000070, 1.236577356246000070, 1.236577356246000070, 1.236577356246000070, 1.236577356246000070, 1.236577356246000070, 1.236577356246000070, 1.236577356246000070) ) ) 
 REPRESENTATION_ITEM ( '' )  SURFACE ( )  );
#6188=CARTESIAN_POINT ( 'NONE',  ( -15.65816392223999820, -7.257913545763996055, -317.5770954168139610 ) ) ;
#6189=B_SPLINE_CURVE_WITH_KNOTS ( 'NONE', 3,
 ( #9640, #3837, #10388, #9750, #6302, #9586, #3892, #5495, #8774, #10441, #1417, #5656, #10556, #4699, #3082, #6358, #2282, #5546, #8835, #4215, #7333, #7438, #3357, #8345, #5713, #9107, #76, #1638, #1794, #7491, #9859, #4270, #7540, #2548, #6577, #6683, #10016, #2443, #6634, #8237, #5065, #8190, #4160, #9910, #983, #5119 ),
 .UNSPECIFIED., .F., .F.,
 ( 4, 2, 2, 2, 2, 2, 2, 2, 2, 2, 2, 2, 2, 2, 2, 2, 2, 2, 2, 2, 2, 2, 4 ),
 ( 0.000000000000000000, 0.001362852592701297230, 0.002044278889051945412, 0.002725705185402593159, 0.004088557778103890823, 0.005451410370805188921, 0.006814262963506486151, 0.008177115556207781646, 0.01090282074161037437, 0.01635423111241555635, 0.01907993629781814388, 0.02180564148322073487, 0.02453134666862332586, 0.02725705185402591685, 0.02998275703942850437, 0.03270846222483109189, 0.03543416741023368288, 0.03815987259563628081, 0.03952272518833757631, 0.04088557778103886486, 0.04224843037374016036, 0.04292985667009080464, 0.04361128296644144198 ),
 .UNSPECIFIED. ) ;
#6195=CARTESIAN_POINT ( 'NONE',  ( -19.79155829785255349, -1.881978406165077500, 319.0000000000003979 ) ) ;
#6197=CARTESIAN_POINT ( 'NONE',  ( -19.97288175887001316, 0.5556452136296999855, 191.1197171614399792 ) ) ;
#6199=CARTESIAN_POINT ( 'NONE',  ( -15.75886148104574325, -3.542954957252464343, 315.0000000000000000 ) ) ;
#6201=CARTESIAN_POINT ( 'NONE',  ( 18.20422786544000715, 5.185156308378004120, 191.1197171614399792 ) ) ;
#6203=LINE ( 'NONE', #3638, #1331 ) ;
#6206=CARTESIAN_POINT ( 'NONE',  ( -4.866278641173998665, 11.00354869785000211, -302.5071922382879279 ) ) ;
#6207=CARTESIAN_POINT ( 'NONE',  ( -18.77791317464001608, -4.479224074632002228, 319.5792614743400009 ) ) ;
#6210=CARTESIAN_POINT ( 'NONE',  ( -6.488017178959999853, 9.182784307579000327, 314.6383426456000052 ) ) ;
#6212=ORIENTED_EDGE ( 'NONE', *, *, #9764, .F. ) ;
#6213=CARTESIAN_POINT ( 'NONE',  ( -11.56561186376999295, -8.976555918559004255, 190.0071920248299477 ) ) ;
#6215=CARTESIAN_POINT ( 'NONE',  ( -18.17597206675998223, 5.223702392620001689, 318.8802828394900644 ) ) ;
#6216=PLANE ( 'NONE',  #845 ) ;
#6218=CARTESIAN_POINT ( 'NONE',  ( -17.34710322845000263, 0.4172063223308000168, 314.6383426456000052 ) ) ;
#6220=CARTESIAN_POINT ( 'NONE',  ( -15.40286302630929427, 3.995001727760178145, 315.0000000000000568 ) ) ;
#6221=CARTESIAN_POINT ( 'NONE',  ( -7.006889269069000115, -6.844138725329000472, 315.0000000000001705 ) ) ;
#6222=CARTESIAN_POINT ( 'NONE',  ( -15.42284054825286610, -3.971008657351323468, -314.9999999999998863 ) ) ;
#6226=CARTESIAN_POINT ( 'NONE',  ( -5.850354798305519743, 8.918567588720486938, -315.0000000000000568 ) ) ;
#6227=CARTESIAN_POINT ( 'NONE',  ( 19.38229133873998222, 1.780473529460998128, 189.9229057364800042 ) ) ;
#6228=CARTESIAN_POINT ( 'NONE',  ( -17.50000000000001776, 8.653894624238266756E-10, 189.9999999999998863 ) ) ;
#6230=CARTESIAN_POINT ( 'NONE',  ( 16.90341843474000072, -5.241942252742000541, -317.4999999999989768 ) ) ;
#6234=CARTESIAN_POINT ( 'NONE',  ( 11.65165375873240450, -6.897932327036405020, 315.0000000000000568 ) ) ;
#6235=CARTESIAN_POINT ( 'NONE',  ( 1.285290206351000108, 10.09749793447999977, -314.4150829855000211 ) ) ;
#6236=CARTESIAN_POINT ( 'NONE',  ( 17.49922277440664686, -0.09424638433143421590, 315.0000000000000000 ) ) ;
#6237=CARTESIAN_POINT ( 'NONE',  ( 12.95511329522999233, 9.055231460430995583, 320.0770942683900557 ) ) ;
#6241=CARTESIAN_POINT ( 'NONE',  ( -2.028805552265000589, 12.03060078454999449, -317.5770954168139610 ) ) ;
#6242=CARTESIAN_POINT ( 'NONE',  ( 20.06704520635998179, 0.4211730678688000440, -317.0792622552969533 ) ) ;
#6255=CARTESIAN_POINT ( 'NONE',  ( -11.75848697160781064, 10.12394145745024510, -316.5000000000004547 ) ) ;
#6257=CARTESIAN_POINT ( 'NONE',  ( 19.99999721801999897, 7.771189452710000131E-11, 191.0000000000000000 ) ) ;
#6258=CARTESIAN_POINT ( 'NONE',  ( -17.39204038057999924, -5.566020924881995846, -302.4229045757450081 ) ) ;
#6259=CARTESIAN_POINT ( 'NONE',  ( 19.96348645057001647, 0.8966426439394996617, 191.1197171614399792 ) ) ;
#6260=EDGE_CURVE ( 'NONE', #7297, #3286, #8120, .T. ) ;
#6263=EDGE_CURVE ( 'NONE', #4067, #10485, #8399, .T. ) ;
#6266=CARTESIAN_POINT ( 'NONE',  ( -12.10743226551000085, -7.094093637544000686, -314.6383426456000052 ) ) ;
#6267=CARTESIAN_POINT ( 'NONE',  ( -8.690073206612000334, 8.569658446474999636, 314.6383426456000052 ) ) ;
#6276=CARTESIAN_POINT ( 'NONE',  ( -16.95014751240671913, 0.8318069206872661381, 315.0000000000000000 ) ) ;
#6277=CARTESIAN_POINT ( 'NONE',  ( -18.45919443845001950, -2.405475664342000996, 319.9928079742500131 ) ) ;
#6279=CARTESIAN_POINT ( 'NONE',  ( 19.99999721132999753, -3.518697978483000342E-10, 319.0000000000000000 ) ) ;
#6283=CARTESIAN_POINT ( 'NONE',  ( -1.574054099965566111, 9.469115279523554918, -315.0000000000001705 ) ) ;
#6284=CARTESIAN_POINT ( 'NONE',  ( -3.087789584922997932, 11.94493704178999671, 189.9229057364800042 ) ) ;
#6289=CARTESIAN_POINT ( 'NONE',  ( 16.47320456655591059, -2.338720490045835820, 314.9999999999999432 ) ) ;
#6290=CARTESIAN_POINT ( 'NONE',  ( 13.56771446467999986, 6.451120369226999607, -314.4150829855000211 ) ) ;
#6291=CARTESIAN_POINT ( 'NONE',  ( 17.40348243411531826, -5.898854857574459487, 315.0000000000000000 ) ) ;
#6292=CARTESIAN_POINT ( 'NONE',  ( -19.54690800120000205, 0.8885403386512999990, 320.0770942683900557 ) ) ;
#6296=CARTESIAN_POINT ( 'NONE',  ( -13.97631948628000309, 9.047145764649998867, -317.0792622552969533 ) ) ;
#6297=CARTESIAN_POINT ( 'NONE',  ( 19.87640215697998158, -1.702148751976998442, -316.3802825947000201 ) ) ;
#6301=ORIENTED_EDGE ( 'NONE', *, *, #10494, .T. ) ;
#6302=CARTESIAN_POINT ( 'NONE',  ( -17.20152651095805041, -1.793788947124295374, -314.5180462286797365 ) ) ;
#6304=CARTESIAN_POINT ( 'NONE',  ( 7.865580335751168661, 11.50505378538359125, -316.5000000000004547 ) ) ;
#6306=CARTESIAN_POINT ( 'NONE',  ( -15.52919946924948569, -3.840693445095582081, 314.9999999999999432 ) ) ;
#6307=CARTESIAN_POINT ( 'NONE',  ( -12.85183647427999176, -9.678193536939003749, -302.9207377450070453 ) ) ;
#6308=DIRECTION ( 'NONE',  ( 0.000000000000000000, 1.000000000000000000, 0.000000000000000000 ) ) ;
#6309=CARTESIAN_POINT ( 'NONE',  ( 17.39204038057999924, 5.566020924881995846, -302.4229045757450081 ) ) ;
#6312=CARTESIAN_POINT ( 'NONE',  ( -15.56325459994999960, -4.731967449628999844, -314.4150829855000211 ) ) ;
#6313=CARTESIAN_POINT ( 'NONE',  ( 12.33444409538000031, 8.732262621622000509, -302.5000000000000000 ) ) ;
#6314=EDGE_LOOP ( 'NONE', ( #8882, #3787, #2171, #6083 ) ) ;
#6315=CARTESIAN_POINT ( 'NONE',  ( -16.06942734036999454, -6.898991720969999797, 189.9229057364800042 ) ) ;
#6316=CARTESIAN_POINT ( 'NONE',  ( 14.79888371878075048, 8.420183212156704400, 190.9999999999996589 ) ) ;
#6319=CARTESIAN_POINT ( 'NONE',  ( -13.18712987686000027, -5.898505050745000311, 315.0848619657999734 ) ) ;
#6320=CARTESIAN_POINT ( 'NONE',  ( 17.49922277440664686, -0.09424638433143421590, 315.0000000000000000 ) ) ;
#6321=CARTESIAN_POINT ( 'NONE',  ( 12.63876572971000023, 8.567575428377999458, 320.0000000000000000 ) ) ;
#6322=CARTESIAN_POINT ( 'NONE',  ( -6.240232637630001911, -10.74449313720999832, 319.9928079742500131 ) ) ;
#6323=CARTESIAN_POINT ( 'NONE',  ( -13.82248977823974734, -5.505663031471445201, -315.0000000000000000 ) ) ;
#6332=CARTESIAN_POINT ( 'NONE',  ( -19.19804233804001115, 3.716674010855997690, 190.4207385301700128 ) ) ;
#6333=CARTESIAN_POINT ( 'NONE',  ( 5.118368704603114087E-10, 10.00000000003099210, 314.4999681336588537 ) ) ;
#6339=CARTESIAN_POINT ( 'NONE',  ( -8.032401884333960851, -11.45915766226284482, -303.4999999999996589 ) ) ;
#6342=CARTESIAN_POINT ( 'NONE',  ( 10.19111349739211292, -9.999999999041103038, 314.4999507458385324 ) ) ;
#6344=CARTESIAN_POINT ( 'NONE',  ( -15.30440697208000600, 7.531500302410004011, 320.0770942683900557 ) ) ;
#6348=CARTESIAN_POINT ( 'NONE',  ( 17.39473599676002635, 5.562790558317003864, -317.5770954168139610 ) ) ;
#6358=CARTESIAN_POINT ( 'NONE',  ( -12.32755932899231688, -7.043638358067994432, -314.5741798689286384 ) ) ;
#6361=CARTESIAN_POINT ( 'NONE',  ( 17.71658133615935782, 5.834976589818514192, -316.5000000000004547 ) ) ;
#6363=CARTESIAN_POINT ( 'NONE',  ( -15.24035984457677628, -4.192874667847209302, 315.0000000000000000 ) ) ;
#6364=CARTESIAN_POINT ( 'NONE',  ( -6.704579698891996564, -11.86746000475999452, -302.9207377450070453 ) ) ;
#6368=CARTESIAN_POINT ( 'NONE',  ( -17.42451203059000520, 5.527343733032997974, -302.4229045757450081 ) ) ;
#6369=CARTESIAN_POINT ( 'NONE',  ( 9.912528015309003848, -10.85837313990000474, 318.8802828394900644 ) ) ;
#6371=CARTESIAN_POINT ( 'NONE',  ( 6.488017178959999853, -9.182784307579000327, -314.6383426456000052 ) ) ;
#6373=ORIENTED_EDGE ( 'NONE', *, *, #4443, .T. ) ;
#6374=CARTESIAN_POINT ( 'NONE',  ( 11.98038374875001111, -9.553300872651998787, 189.9229057364800042 ) ) ;
#6375=CARTESIAN_POINT ( 'NONE',  ( -14.83495203015046116, 8.394818437327874250, 190.9999999999996589 ) ) ;
#6376=LINE ( 'NONE', #2462, #6175 ) ;
#6377=ORIENTED_EDGE ( 'NONE', *, *, #7985, .T. ) ;
#6379=CARTESIAN_POINT ( 'NONE',  ( -8.519003879469000395, -8.390442916014999142, 314.8616023057000461 ) ) ;
#6383=CARTESIAN_POINT ( 'NONE',  ( 13.15646768860627169, 9.424872508248352432, 319.0000000000005116 ) ) ;
#6390=CARTESIAN_POINT ( 'NONE',  ( -18.75098855781002882, 3.495875360606998772, 189.9229057364800042 ) ) ;
#6391=CARTESIAN_POINT ( 'NONE',  ( 10.23467949917770525, 9.999999999493887515, -302.4999999999997158 ) ) ;
#6396=CARTESIAN_POINT ( 'NONE',  ( 16.99996037728000076, -1.352915776343000118E-09, 314.9999801883000146 ) ) ;
#6398=CARTESIAN_POINT ( 'NONE',  ( -6.687916194383508817, -11.79215677264876838, -303.4999999999996589 ) ) ;
#6400=CARTESIAN_POINT ( 'NONE',  ( 15.23514566747999943, 4.427644513407000382, -314.8616023057000461 ) ) ;
#6402=CARTESIAN_POINT ( 'NONE',  ( 13.82465948680000878, 8.551125454139995696, 320.0770942683900557 ) ) ;
#6405=ORIENTED_EDGE ( 'NONE', *, *, #6008, .T. ) ;
#6406=CARTESIAN_POINT ( 'NONE',  ( -19.46922894822000316, 1.611824300579999925, -317.5770954168139610 ) ) ;
#6407=CARTESIAN_POINT ( 'NONE',  ( -19.97262988322000865, 0.5553097472237004117, -316.3802825947000201 ) ) ;
#6409=CARTESIAN_POINT ( 'NONE',  ( -1.295798468764000066, -11.49282963429000048, 320.0000000000000000 ) ) ;
#6417=CARTESIAN_POINT ( 'NONE',  ( -13.97618761079829142, -5.383201530108604693, 314.9999999999999432 ) ) ;
#6418=CARTESIAN_POINT ( 'NONE',  ( -3.702588368219998927, -12.37624192652999966, -302.9207377450070453 ) ) ;
#6425=CARTESIAN_POINT ( 'NONE',  ( -18.93783568409002172, 3.175510411809001177, -302.4229045757450081 ) ) ;
#6426=CARTESIAN_POINT ( 'NONE',  ( 8.771473555299991176, -11.23637119458999223, 318.8802828394900644 ) ) ;
#6428=CARTESIAN_POINT ( 'NONE',  ( -13.18712987686000027, -5.898505050745000311, -315.0848619657999734 ) ) ;
#6429=CARTESIAN_POINT ( 'NONE',  ( -17.35381917807999841, -0.3185724951638000402, 314.6383426456000052 ) ) ;
#6431=CARTESIAN_POINT ( 'NONE',  ( 18.75098855781002882, -3.495875360606998772, 189.9229057364800042 ) ) ;
#6432=CARTESIAN_POINT ( 'NONE',  ( -7.783073706837757122, 11.52583533951409933, 190.9999999999996589 ) ) ;
#6435=MECHANICAL_DESIGN_GEOMETRIC_PRESENTATION_REPRESENTATION('',(#6089),#9695);
#6436=CARTESIAN_POINT ( 'NONE',  ( -6.370857846455999507, -9.209451711050000711, 314.6383426456000052 ) ) ;
#6437=CARTESIAN_POINT ( 'NONE',  ( 16.99996037728000076, -1.352915776343000118E-09, 314.9999801883000146 ) ) ;
#6438=CARTESIAN_POINT ( 'NONE',  ( -18.20355969383999906, 3.293069710501999925, 320.0000000000000000 ) ) ;
#6440=CARTESIAN_POINT ( 'NONE',  ( 14.04520818109275737, 8.909665382566956282, 319.0000000000005116 ) ) ;
#6442=CARTESIAN_POINT ( 'NONE',  ( -15.00000000000000000, 0.4945770392355999800, 315.0000000000000000 ) ) ;
#6446=CARTESIAN_POINT ( 'NONE',  ( -17.06589079541999965, 6.642208448352997507, 190.4207385301700128 ) ) ;
#6450=CARTESIAN_POINT ( 'NONE',  ( 15.46063250253144972, 3.925225575964395919, 315.0000000000000568 ) ) ;
#6452=CARTESIAN_POINT ( 'NONE',  ( 17.74743742734688112, -5.798256014711219208, -303.4999999999996589 ) ) ;
#6453=CARTESIAN_POINT ( 'NONE',  ( 17.11849373668000140, 0.6181952683021999517, -314.8616023057000461 ) ) ;
#6454=DIRECTION ( 'NONE',  ( 0.000000000000000000, 0.000000000000000000, 1.000000000000000000 ) ) ;
#6455=CARTESIAN_POINT ( 'NONE',  ( -18.20429351259000228, 3.291556992836000006, 190.0000000000000000 ) ) ;
#6456=CARTESIAN_POINT ( 'NONE',  ( 7.740399053647997185, 11.10168159160000201, 320.0770942683900557 ) ) ;
#6459=CARTESIAN_POINT ( 'NONE',  ( 16.84537440012000786, 6.754000406595005224, -316.3802825947000201 ) ) ;
#6460=CARTESIAN_POINT ( 'NONE',  ( -9.192918156740001123, -11.10629030388999894, -316.3802825947000201 ) ) ;
#6462=CARTESIAN_POINT ( 'NONE',  ( 14.93129073739000034, -7.087303338045999546, 320.0000000000000000 ) ) ;
#6472=CARTESIAN_POINT ( 'NONE',  ( -0.7882946689300455168, -9.499899501988618766, 315.0000000000000000 ) ) ;
#6473=CARTESIAN_POINT ( 'NONE',  ( -15.65461689722998706, -7.260828390490999595, -302.4229045757450081 ) ) ;
#6479=PRESENTATION_STYLE_ASSIGNMENT (( #7290 ) ) ;
#6480=ORIENTED_EDGE ( 'NONE', *, *, #7655, .F. ) ;
#6481=CARTESIAN_POINT ( 'NONE',  ( 20.06799914428001941, -0.4075895895062001673, -302.9207377450070453 ) ) ;
#6483=ORIENTED_EDGE ( 'NONE', *, *, #6986, .T. ) ;
#6484=CARTESIAN_POINT ( 'NONE',  ( 8.690073206612000334, -8.569658446474999636, -314.6383426456000052 ) ) ;
#6485=ADVANCED_FACE ( 'NONE', ( #10071 ), #1956, .F. ) ;
#6486=CARTESIAN_POINT ( 'NONE',  ( 19.99999721801999897, 7.771189452710000131E-11, 191.0000000000000000 ) ) ;
#6488=CARTESIAN_POINT ( 'NONE',  ( 19.57080534385999471, 0.3817780055853002841, 189.9229057364800042 ) ) ;
#6489=CIRCLE ( 'NONE', #9237, 0.9999999999999755751 ) ;
#6490=CARTESIAN_POINT ( 'NONE',  ( 19.51240441859934194, 2.792009854621256171, 190.9999999999996589 ) ) ;
#6491=CARTESIAN_POINT ( 'NONE',  ( 4.578722611353294170, 9.145541810471781830, -315.0000000000000568 ) ) ;
#6493=CARTESIAN_POINT ( 'NONE',  ( -16.19514236092000203, -2.730451569713999938, 315.0848619657999734 ) ) ;
#6495=CARTESIAN_POINT ( 'NONE',  ( -10.58225433500999912, 9.538747186136999900, 320.0000000000000000 ) ) ;
#6497=CARTESIAN_POINT ( 'NONE',  ( -18.68762439754708637, 4.478870766961970062, 319.0000000000005116 ) ) ;
#6499=CARTESIAN_POINT ( 'NONE',  ( 15.00000000000326139, -5.136019918588313243E-17, 315.0000000000001137 ) ) ;
#6500=ORIENTED_EDGE ( 'NONE', *, *, #9162, .T. ) ;
#6504=CARTESIAN_POINT ( 'NONE',  ( 3.131429216827940247E-09, -12.50000000000000000, -303.5000000000000000 ) ) ;
#6505=CARTESIAN_POINT ( 'NONE',  ( -16.99996037728000076, 1.352916535802999941E-09, -314.9999801883000146 ) ) ;
#6507=CARTESIAN_POINT ( 'NONE',  ( -17.19853431800999743, 2.231396706187000145, -315.0000000000000000 ) ) ;
#6510=CARTESIAN_POINT ( 'NONE',  ( 14.87617152917998631, 8.357511890987989744, 318.8802828394900644 ) ) ;
#6512=CARTESIAN_POINT ( 'NONE',  ( 7.006889269069000115, 6.844138725329000472, 315.0000000000001705 ) ) ;
#6514=CARTESIAN_POINT ( 'NONE',  ( 19.37639879579000635, 3.420933338561999548, -317.0792622552969533 ) ) ;
#6515=CARTESIAN_POINT ( 'NONE',  ( 9.372233899709991434, -11.04684900435999495, -316.3802825947000201 ) ) ;
#6518=CARTESIAN_POINT ( 'NONE',  ( -19.00000000000000000, 0.000000000000000000, 319.9999999999899956 ) ) ;
#6520=CARTESIAN_POINT ( 'NONE',  ( -18.99997865338999858, 1.260542274312000007E-06, -316.5000000000000000 ) ) ;
#6521=CARTESIAN_POINT ( 'NONE',  ( 11.76997148278789673, -6.834709328092291258, -315.0000000000000568 ) ) ;
#6524=CARTESIAN_POINT ( 'NONE',  ( -12.98706127646999953, 6.788989183774999603, -314.4963898845653603 ) ) ;
#6526=CARTESIAN_POINT ( 'NONE',  ( 13.35645252658000004, 8.162105094466999944, -317.5000000000000000 ) ) ;
#6528=CARTESIAN_POINT ( 'NONE',  ( 5.044863629634003921, -12.10215170741999557, -303.6197174156509391 ) ) ;
#6530=CARTESIAN_POINT ( 'NONE',  ( 19.00000000000000000, 0.000000000000000000, 190.0000000000100044 ) ) ;
#6535=CARTESIAN_POINT ( 'NONE',  ( -12.66297984401999166, 9.215363186789998551, -302.4229045757450081 ) ) ;
#6538=CARTESIAN_POINT ( 'NONE',  ( -17.20518503178000103, -1.389427005613000032, -314.6383426456000052 ) ) ;
#6540=ORIENTED_EDGE ( 'NONE', *, *, #6263, .F. ) ;
#6541=CARTESIAN_POINT ( 'NONE',  ( -17.30501060709000072, -4.528037784100006569, 190.0071920248299477 ) ) ;
#6542=CARTESIAN_POINT ( 'NONE',  ( -15.61921319513150230, 7.819487029138878498, 190.9999999999996589 ) ) ;
#6543=CARTESIAN_POINT ( 'NONE',  ( 12.16683899257771806, 6.621314373557692257, -315.0000000000001137 ) ) ;
#6546=CARTESIAN_POINT ( 'NONE',  ( -15.39920013370999996, -4.579805981517999669, 314.6383426456000052 ) ) ;
#6548=CARTESIAN_POINT ( 'NONE',  ( 17.35388116884000098, 4.663644590058999562, 320.0000000000000000 ) ) ;
#6549=CARTESIAN_POINT ( 'NONE',  ( 11.81011838702999484, -9.634252844421009598, 320.0770942683900557 ) ) ;
#6550=CARTESIAN_POINT ( 'NONE',  ( 10.19008647966648873, 10.76511244458322558, 319.0000000000005116 ) ) ;
#6551=FACE_OUTER_BOUND ( 'NONE', #9372, .T. ) ;
#6560=CARTESIAN_POINT ( 'NONE',  ( -19.86375996897344010, -1.775925728142829341, -303.4999999999996589 ) ) ;
#6561=CARTESIAN_POINT ( 'NONE',  ( 15.71297435277999810, 3.490404421959999670, -315.0848619657999734 ) ) ;
#6563=CARTESIAN_POINT ( 'NONE',  ( -19.00000000000000000, 0.000000000000000000, 190.0000000000100044 ) ) ;
#6566=CARTESIAN_POINT ( 'NONE',  ( 13.57573464316000056, 3.225916527208000151, -284.9999999999999432 ) ) ;
#6568=CARTESIAN_POINT ( 'NONE',  ( 16.90418428017002839, 6.814536637555997700, -317.0792622552969533 ) ) ;
#6570=CARTESIAN_POINT ( 'NONE',  ( -11.73784133842000088, -9.026952533543999735, 320.0000000000000000 ) ) ;
#6575=CARTESIAN_POINT ( 'NONE',  ( 14.08970834377950965, -5.290460773273633954, -315.0000000000000568 ) ) ;
#6577=CARTESIAN_POINT ( 'NONE',  ( 14.57677553938589554, -5.476482737502805342, -314.5817494731896886 ) ) ;
#6579=CARTESIAN_POINT ( 'NONE',  ( -0.2188334844706000260, 11.51755598686999882, -317.5000000000000000 ) ) ;
#6581=CARTESIAN_POINT ( 'NONE',  ( 12.89386942443999295, -9.656754267509002787, -302.9207377450070453 ) ) ;
#6583=CARTESIAN_POINT ( 'NONE',  ( 10.44399617086000021, -10.22112142899999476, -317.5770954168139610 ) ) ;
#6586=CARTESIAN_POINT ( 'NONE',  ( 13.88537659940002023, 9.003549035645995957, -303.6197174156520759 ) ) ;
#6588=CARTESIAN_POINT ( 'NONE',  ( -10.25126261553517537, 10.00000004282989785, 314.4997059534069308 ) ) ;
#6589=ORIENTED_EDGE ( 'NONE', *, *, #5029, .F. ) ;
#6594=CARTESIAN_POINT ( 'NONE',  ( -17.70739197152998656, -5.947706840970997888, 190.4207385301700128 ) ) ;
#6595=CARTESIAN_POINT ( 'NONE',  ( -17.19853431800999743, -2.231396706187000145, -314.4944826805095772 ) ) ;
#6601=CARTESIAN_POINT ( 'NONE',  ( 16.77957632114000219, -1.244976636274000015, 315.0848619657999734 ) ) ;
#6603=CARTESIAN_POINT ( 'NONE',  ( 17.84276444133998041, -4.978015457891998174, 320.0770942683900557 ) ) ;
#6605=PRESENTATION_STYLE_ASSIGNMENT (( #9025 ) ) ;
#6606=CARTESIAN_POINT ( 'NONE',  ( 16.89608781496000134, 0.5923740909019999945, 315.0848619657999734 ) ) ;
#6608=CARTESIAN_POINT ( 'NONE',  ( 15.61921319513150053, -7.819487029138875833, 190.9999999999995737 ) ) ;
#6613=AXIS2_PLACEMENT_3D ( 'NONE', #625, #5501, #6308 ) ;
#6616=CARTESIAN_POINT ( 'NONE',  ( 16.91975252613927694, 1.077737682115706086, 314.9999999999999432 ) ) ;
#6622=CARTESIAN_POINT ( 'NONE',  ( -18.78737820286000115, 1.762683282930000095, 190.0000000000000000 ) ) ;
#6625=CARTESIAN_POINT ( 'NONE',  ( 10.23467085909357976, -10.00000000050611781, 190.0000000000003695 ) ) ;
#6626=CARTESIAN_POINT ( 'NONE',  ( -19.87640215697998158, 1.702148751976998442, -316.3802825947000201 ) ) ;
#6627=CARTESIAN_POINT ( 'NONE',  ( -10.79636471171000167, -9.449795599854001082, 320.0000000000000000 ) ) ;
#6628=( BOUNDED_SURFACE ( )  B_SPLINE_SURFACE ( 3, 3, ( 
 ( #8625, #1272, #3800, #8682, #8574, #7677, #10305, #472, #7090, #1120, #6111, #6159, #4402, #321, #6983, #5252, #3595, #8526, #3744, #7728, #1219, #3645, #6928, #7033, #9398, #2033, #5300, #9447, #4496, #2941, #7773, #417, #10254, #6213, #8903, #1494, #8154, #3263, #8852, #2297, #792, #6541, #1604, #8735, #9714, #10571, #4771, #9601, #4071, #3213 ),
 ( #1546, #6488, #9767, #5511, #1377, #2242, #6431, #2405, #4662, #8041, #5673, #689, #10457, #7996, #7349, #8097, #6374, #3908, #2356, #8791, #7936, #1433, #740, #8958, #634, #578, #5622, #4720, #4876, #3858, #3044, #4826, #3961, #7188, #3098, #4016, #7241, #9657, #6315, #7298, #10621, #9819, #2459, #10512, #7137, #10405, #5566, #3156, #841, #9978 ),
 ( #5777, #5080, #3533, #8203, #5946, #2620, #9233, #6811, #4337, #9122, #5882, #40, #4231, #4125, #7401, #9175, #4286, #1815, #10084, #1053, #7609, #892, #5134, #1865, #8360, #4178, #2562, #998, #3479, #258, #3315, #1651, #9925, #5727, #9016, #3372, #8413, #4927, #5830, #1756, #6594, #9876, #2513, #9068, #6700, #7558, #5026, #1704, #4977, #203 ),
 ( #6760, #10032, #8253, #8306, #947, #7505, #7451, #95, #6649, #147, #3421, #2676, #3786, #7866, #6914, #2773, #4593, #6969, #459, #1258, #2929, #9386, #10186, #10242, #6147, #8560, #7760, #9434, #4437, #4390, #9285, #6099, #4535, #1312, #2830, #7664, #3733, #402, #2020, #5287, #7020, #1970, #1206, #6863, #10292, #515, #1104, #6044, #7073, #6197 ) ),
 .UNSPECIFIED., .F., .F., .T. ) 
 B_SPLINE_SURFACE_WITH_KNOTS ( ( 4, 4 ),
 ( 4, 1, 1, 1, 1, 1, 1, 1, 1, 1, 1, 1, 1, 1, 1, 1, 1, 1, 1, 1, 1, 1, 1, 1, 1, 1, 1, 1, 1, 1, 1, 1, 1, 1, 1, 1, 1, 1, 1, 1, 1, 1, 1, 1, 1, 1, 1, 4 ),
 ( 0.000000000000000000, 1.000000000000000000 ),
 ( -0.008478179454678999930, 0.000000000000000000, 0.01942502340896999982, 0.03767429839031000149, 0.05516856733836000143, 0.07225070737889999206, 0.08921661857028999332, 0.1062419522249000020, 0.1231986756591000043, 0.1401197909732000146, 0.1574955775699000138, 0.1756558812635999889, 0.1944176066207999876, 0.2136589569993999904, 0.2335613621991999844, 0.2542018781120999882, 0.2753083038155999529, 0.2968879296931000167, 0.3196642413612000300, 0.3444503751709999673, 0.3720414184181000117, 0.4028839481288000179, 0.4370422198952000348, 0.4744802605176999810, 0.5138140658555000462, 0.5525504936030000147, 0.5886556970966999591, 0.6214671571023999697, 0.6505675624772999655, 0.6761140898808000177, 0.6991730762615999684, 0.7208971548058999979, 0.7423774111579999335, 0.7637103432859999597, 0.7842694365818000390, 0.8040102150915000578, 0.8232128915810998926, 0.8418292181656999995, 0.8596651317910000145, 0.8769212066234000069, 0.8939598742608000359, 0.9109129999441000214, 0.9278339763510999871, 0.9449158864711000305, 0.9624195949295000219, 0.9806529035300000086, 1.000000000000000000, 1.007725586608000157 ),
 .UNSPECIFIED. ) 
 GEOMETRIC_REPRESENTATION_ITEM ( )  RATIONAL_B_SPLINE_SURFACE ( (
 ( 1.236576749365999817, 1.236576749365999817, 1.236576749365999817, 1.236576749365999817, 1.236576749365999817, 1.236576749365999817, 1.236576749365999817, 1.236576749365999817, 1.236576749365999817, 1.236576749365999817, 1.236576749365999817, 1.236576749365999817, 1.236576749365999817, 1.236576749365999817, 1.236576749365999817, 1.236576749365999817, 1.236576749365999817, 1.236576749365999817, 1.236576749365999817, 1.236576749365999817, 1.236576749365999817, 1.236576749365999817, 1.236576749365999817, 1.236576749365999817, 1.236576749365999817, 1.236576749365999817, 1.236576749365999817, 1.236576749365999817, 1.236576749365999817, 1.236576749365999817, 1.236576749365999817, 1.236576749365999817, 1.236576749365999817, 1.236576749365999817, 1.236576749365999817, 1.236576749365999817, 1.236576749365999817, 1.236576749365999817, 1.236576749365999817, 1.236576749365999817, 1.236576749365999817, 1.236576749365999817, 1.236576749365999817, 1.236576749365999817, 1.236576749365999817, 1.236576749365999817, 1.236576749365999817, 1.236576749365999817, 1.236576749365999817, 1.236576749365999817),
 ( 0.9211410835446999235, 0.9211410835446999235, 0.9211410835446999235, 0.9211410835446999235, 0.9211410835446999235, 0.9211410835446999235, 0.9211410835446999235, 0.9211410835446999235, 0.9211410835446999235, 0.9211410835446999235, 0.9211410835446999235, 0.9211410835446999235, 0.9211410835446999235, 0.9211410835446999235, 0.9211410835446999235, 0.9211410835446999235, 0.9211410835446999235, 0.9211410835446999235, 0.9211410835446999235, 0.9211410835446999235, 0.9211410835446999235, 0.9211410835446999235, 0.9211410835446999235, 0.9211410835446999235, 0.9211410835446999235, 0.9211410835446999235, 0.9211410835446999235, 0.9211410835446999235, 0.9211410835446999235, 0.9211410835446999235, 0.9211410835446999235, 0.9211410835446999235, 0.9211410835446999235, 0.9211410835446999235, 0.9211410835446999235, 0.9211410835446999235, 0.9211410835446999235, 0.9211410835446999235, 0.9211410835446999235, 0.9211410835446999235, 0.9211410835446999235, 0.9211410835446999235, 0.9211410835446999235, 0.9211410835446999235, 0.9211410835446999235, 0.9211410835446999235, 0.9211410835446999235, 0.9211410835446999235, 0.9211410835446999235, 0.9211410835446999235),
 ( 0.9211410835446999235, 0.9211410835446999235, 0.9211410835446999235, 0.9211410835446999235, 0.9211410835446999235, 0.9211410835446999235, 0.9211410835446999235, 0.9211410835446999235, 0.9211410835446999235, 0.9211410835446999235, 0.9211410835446999235, 0.9211410835446999235, 0.9211410835446999235, 0.9211410835446999235, 0.9211410835446999235, 0.9211410835446999235, 0.9211410835446999235, 0.9211410835446999235, 0.9211410835446999235, 0.9211410835446999235, 0.9211410835446999235, 0.9211410835446999235, 0.9211410835446999235, 0.9211410835446999235, 0.9211410835446999235, 0.9211410835446999235, 0.9211410835446999235, 0.9211410835446999235, 0.9211410835446999235, 0.9211410835446999235, 0.9211410835446999235, 0.9211410835446999235, 0.9211410835446999235, 0.9211410835446999235, 0.9211410835446999235, 0.9211410835446999235, 0.9211410835446999235, 0.9211410835446999235, 0.9211410835446999235, 0.9211410835446999235, 0.9211410835446999235, 0.9211410835446999235, 0.9211410835446999235, 0.9211410835446999235, 0.9211410835446999235, 0.9211410835446999235, 0.9211410835446999235, 0.9211410835446999235, 0.9211410835446999235, 0.9211410835446999235),
 ( 1.236576749365999817, 1.236576749365999817, 1.236576749365999817, 1.236576749365999817, 1.236576749365999817, 1.236576749365999817, 1.236576749365999817, 1.236576749365999817, 1.236576749365999817, 1.236576749365999817, 1.236576749365999817, 1.236576749365999817, 1.236576749365999817, 1.236576749365999817, 1.236576749365999817, 1.236576749365999817, 1.236576749365999817, 1.236576749365999817, 1.236576749365999817, 1.236576749365999817, 1.236576749365999817, 1.236576749365999817, 1.236576749365999817, 1.236576749365999817, 1.236576749365999817, 1.236576749365999817, 1.236576749365999817, 1.236576749365999817, 1.236576749365999817, 1.236576749365999817, 1.236576749365999817, 1.236576749365999817, 1.236576749365999817, 1.236576749365999817, 1.236576749365999817, 1.236576749365999817, 1.236576749365999817, 1.236576749365999817, 1.236576749365999817, 1.236576749365999817, 1.236576749365999817, 1.236576749365999817, 1.236576749365999817, 1.236576749365999817, 1.236576749365999817, 1.236576749365999817, 1.236576749365999817, 1.236576749365999817, 1.236576749365999817, 1.236576749365999817) ) ) 
 REPRESENTATION_ITEM ( '' )  SURFACE ( )  );
#6631=CARTESIAN_POINT ( 'NONE',  ( 1.574054099965567444, -9.469115279523553141, -315.0000000000000568 ) ) ;
#6633=COLOUR_RGB ( '', 0.40784314, 0.44705882, 0.49803922) ;
#6634=CARTESIAN_POINT ( 'NONE',  ( 16.63862268811587697, -3.034640078201989777, -314.5459747968307056 ) ) ;
#6635=EDGE_LOOP ( 'NONE', ( #5496, #458, #6500, #7374 ) ) ;
#6638=CARTESIAN_POINT ( 'NONE',  ( 1.673754838359998498, -12.46646309164999522, -303.6197174156509391 ) ) ;
#6639=CARTESIAN_POINT ( 'NONE',  ( 7.796607451809997258, -10.36222334076000529, -317.4928077629770087 ) ) ;
#6642=FILL_AREA_STYLE ('',( #8296 ) ) ;
#6646=CARTESIAN_POINT ( 'NONE',  ( -17.36972170382999892, -0.04551883977364000466, -314.6383426456000052 ) ) ;
#6649=CARTESIAN_POINT ( 'NONE',  ( 18.17619403612001250, -5.223318733890998544, 191.1197171614399792 ) ) ;
#6650=CARTESIAN_POINT ( 'NONE',  ( -17.19853431800999743, -2.231396706187000145, -315.0000000000001137 ) ) ;
#6653=CARTESIAN_POINT ( 'NONE',  ( 4.478082317681002955, 12.27758592791000147, 190.4207385301700128 ) ) ;
#6654=CARTESIAN_POINT ( 'NONE',  ( 17.35381917807999841, 0.3185724951638000402, 314.6383426456000052 ) ) ;
#6656=CARTESIAN_POINT ( 'NONE',  ( 18.86319819242002183, 0.4765179085981003926, 319.9928079742500131 ) ) ;
#6658=CARTESIAN_POINT ( 'NONE',  ( -17.49966312145123482, 0.4461383192961264621, 314.4999388432775049 ) ) ;
#6659=CARTESIAN_POINT ( 'NONE',  ( 12.81623431846864136, 9.609762277177448908, -303.4999999999990905 ) ) ;
#6661=CARTESIAN_POINT ( 'NONE',  ( 16.19514236092000203, 2.730451569713999938, 315.0848619657999734 ) ) ;
#6663=CARTESIAN_POINT ( 'NONE',  ( -2.649465170253727297, -12.40913386102118210, 190.9999999999995737 ) ) ;
#6666=CARTESIAN_POINT ( 'NONE',  ( 5.850395566949658566, 8.918560297860793185, 315.0000000000000000 ) ) ;
#6668=EDGE_LOOP ( 'NONE', ( #4835, #291 ) ) ;
#6672=CARTESIAN_POINT ( 'NONE',  ( 11.56195786956000049, 9.110631795823000090, 190.0000000000000000 ) ) ;
#6673=CARTESIAN_POINT ( 'NONE',  ( -11.28781796570999951, 4.951468039558000633, 315.0000000000001705 ) ) ;
#6675=CARTESIAN_POINT ( 'NONE',  ( 6.467159262072997628, 11.83367582535999141, -316.3802825947000201 ) ) ;
#6679=CARTESIAN_POINT ( 'NONE',  ( 16.99996037728000076, -1.352915083302999933E-09, -314.9999801883000146 ) ) ;
#6681=CARTESIAN_POINT ( 'NONE',  ( 10.54249803899487503, -7.451732067202642362, -315.0000000000000568 ) ) ;
#6683=CARTESIAN_POINT ( 'NONE',  ( 15.54345086749722427, -4.503564883714266998, -314.5712070352258820 ) ) ;
#6685=CARTESIAN_POINT ( 'NONE',  ( 18.86945318303000008, 1.615078380336999908, -317.5000000000470095 ) ) ;
#6687=CARTESIAN_POINT ( 'NONE',  ( 12.85477847496998827, -9.582024189157998251, -303.6197174156520759 ) ) ;
#6693=CARTESIAN_POINT ( 'NONE',  ( -13.97988708520999701, 9.045087908074000538, -302.9207377450070453 ) ) ;
#6695=CARTESIAN_POINT ( 'NONE',  ( 2.381287022736665303E-07, -10.00000000000000000, 314.4997059534069308 ) ) ;
#6698=CARTESIAN_POINT ( 'NONE',  ( -17.63021146919999893, 4.299866645372000029, -302.4999999999969873 ) ) ;
#6700=CARTESIAN_POINT ( 'NONE',  ( -19.58491037614999897, -2.818636756334000903, 190.4207385301700128 ) ) ;
#6703=B_SPLINE_CURVE_WITH_KNOTS ( 'NONE', 3,
 ( #4503, #7780, #2090, #5357, #4077, #3967, #798, #6548, #8799, #3105, #5517, #4561, #1440, #4728, #6321, #642, #8857, #4024, #8967, #10576, #847, #9022, #7248, #8001, #7355, #3218, #1499, #3270, #9773, #5575, #7304, #6495, #5627, #4831, #2414, #4781, #3918, #9609, #3163, #1610, #1658, #8102, #6438, #9662, #7195, #744, #9827, #5680 ),
 .UNSPECIFIED., .F., .F.,
 ( 4, 1, 1, 1, 1, 1, 1, 1, 1, 1, 1, 1, 1, 1, 1, 1, 1, 1, 1, 1, 1, 1, 1, 1, 1, 1, 1, 1, 1, 1, 1, 1, 1, 1, 1, 1, 1, 1, 1, 1, 1, 1, 1, 1, 1, 4 ),
 ( 0.000000000000000000, 0.02222222222221999915, 0.04444444444443999831, 0.06666666666666999641, 0.08888888888889000250, 0.1111111111111000027, 0.1333333333332999970, 0.1555555555555999947, 0.1777777777777999890, 0.2000000000000000111, 0.2222222222222000054, 0.2444444444443999997, 0.2666666666666999697, 0.2888888888889000195, 0.3111111111111000138, 0.3333333333333000081, 0.3555555555556000336, 0.3777777777777999724, 0.4000000000000000222, 0.4222222222221999610, 0.4444444444444000109, 0.4666666666666999808, 0.4888888888889000306, 0.5111111111110999694, 0.5333333333333000192, 0.5555555555555999891, 0.5777777777778000390, 0.5999999999999999778, 0.6222222222222000276, 0.6444444444443999664, 0.6666666666667000474, 0.6888888888888999862, 0.7111111111111000360, 0.7333333333333000859, 0.7555555555556000558, 0.7777777777777999946, 0.8000000000000000444, 0.8222222222221999832, 0.8444444444443999220, 0.8666666666667000030, 0.8888888888888999418, 0.9111111111110999916, 0.9333333333333000414, 0.9555555555556000114, 0.9777777777778000612, 1.000000000000000000 ),
 .UNSPECIFIED. ) ;
#6705=CARTESIAN_POINT ( 'NONE',  ( -12.19509678855998835, 10.00267306739999640, 190.4207385301700128 ) ) ;
#6707=CARTESIAN_POINT ( 'NONE',  ( 12.17979804859000126, -7.053762231097000068, 314.6383426456000052 ) ) ;
#6709=CARTESIAN_POINT ( 'NONE',  ( -18.35207017878000357, -4.220106527025000887, 320.0770942683900557 ) ) ;
#6711=CARTESIAN_POINT ( 'NONE',  ( 9.314945463565894812, 11.07333627012143573, -303.4999999999990905 ) ) ;
#6712=CARTESIAN_POINT ( 'NONE',  ( 10.32396869588999877, 7.471487098147999717, 315.0848619657999734 ) ) ;
#6715=CARTESIAN_POINT ( 'NONE',  ( -13.93599793909949369, -8.976999749472309276, 190.9999999999995737 ) ) ;
#6717=CARTESIAN_POINT ( 'NONE',  ( 19.78455541125000750, 1.880268586931002073, 318.8802828394900644 ) ) ;
#6719=ORIENTED_EDGE ( 'NONE', *, *, #2398, .F. ) ;
#6721=CARTESIAN_POINT ( 'NONE',  ( -13.67632236045006167, 5.618997091738346050, 315.0000000000000000 ) ) ;
#6723=CARTESIAN_POINT ( 'NONE',  ( -13.57573464316000056, -3.225916527208000151, -285.0000000000000000 ) ) ;
#6725=CARTESIAN_POINT ( 'NONE',  ( 14.35075321877000043, -7.519064610420000072, -302.5000000000000000 ) ) ;
#6728=CARTESIAN_POINT ( 'NONE',  ( 10.60011422839999895, 9.531420659438001763, 190.0000000000000000 ) ) ;
#6729=CARTESIAN_POINT ( 'NONE',  ( 9.425149342036858613, -8.435515065082231700, 314.4999430218500720 ) ) ;
#6735=CARTESIAN_POINT ( 'NONE',  ( 18.99998145310000197, -0.3132853329045000024, 319.9999999999899956 ) ) ;
#6739=CARTESIAN_POINT ( 'NONE',  ( 17.50000000000000000, 0.7437989020623000380, -315.0000000000000000 ) ) ;
#6740=CARTESIAN_POINT ( 'NONE',  ( 15.46045765806406891, -3.925441769934805869, -315.0000000000001137 ) ) ;
#6743=CARTESIAN_POINT ( 'NONE',  ( 17.50000000000107292, 0.7437989020622546299, -315.0000000000001137 ) ) ;
#6747=VERTEX_POINT ( 'NONE', #4950 ) ;
#6748=CARTESIAN_POINT ( 'NONE',  ( 18.63306024686997375, -4.746768565380000027, -302.9207377450070453 ) ) ;
#6749=CARTESIAN_POINT ( 'NONE',  ( -13.31532601970998897, -8.047348965112000485, -317.4928077629770087 ) ) ;
#6750=ADVANCED_FACE ( 'NONE', ( #2485 ), #8540, .F. ) ;
#6751=VECTOR ( 'NONE', #7808, 1000.000000000000000 ) ;
#6752=CARTESIAN_POINT ( 'NONE',  ( 17.50000000000000000, 0.000000000000000000, -314.4999343908002629 ) ) ;
#6754=CARTESIAN_POINT ( 'NONE',  ( -12.85477847496998827, 9.582024189157998251, -303.6197174156520759 ) ) ;
#6759=VERTEX_POINT ( 'NONE', #6113 ) ;
#6760=CARTESIAN_POINT ( 'NONE',  ( 19.97280825118999914, 0.5561396363675005228, 191.1197171614399792 ) ) ;
#6763=CARTESIAN_POINT ( 'NONE',  ( -20.00511239988002998, 0.1020359997562000631, 191.1197171614399792 ) ) ;
#6765=CARTESIAN_POINT ( 'NONE',  ( 16.97404422732000029, -2.118410180888999683, 314.6383426456000052 ) ) ;
#6768=CARTESIAN_POINT ( 'NONE',  ( 10.81481884307000207, -10.07000335707000538, 320.0770942683900557 ) ) ;
#6770=CARTESIAN_POINT ( 'NONE',  ( -5.046018101664360600, 12.10925368423180437, -303.5000000000000000 ) ) ;
#6771=CARTESIAN_POINT ( 'NONE',  ( 16.98808798087999961, 1.334629195702000004, 314.8616023057000461 ) ) ;
#6774=CARTESIAN_POINT ( 'NONE',  ( -2.578726422179000721, 12.49238522902999726, 319.5792614743400009 ) ) ;
#6778=CARTESIAN_POINT ( 'NONE',  ( 8.666088325696231109, 8.161304309888411268, 315.0000000000000568 ) ) ;
#6784=CARTESIAN_POINT ( 'NONE',  ( 13.37992741786000117, -8.147955808703001068, -302.5000000000000000 ) ) ;
#6785=CARTESIAN_POINT ( 'NONE',  ( 0.000000000000000000, 0.000000000000000000, -285.0000000000000000 ) ) ;
#6786=CARTESIAN_POINT ( 'NONE',  ( 18.95710617844000012, 0.9155000425601000913, 190.0000000000000000 ) ) ;
#6787=CARTESIAN_POINT ( 'NONE',  ( -15.60727917143683463, 3.742131089528406118, -315.0000000000000568 ) ) ;
#6788=CARTESIAN_POINT ( 'NONE',  ( -14.79012398734008293, 1.483731117706880154, 315.0000000000001705 ) ) ;
#6792=CARTESIAN_POINT ( 'NONE',  ( 18.53283357168000123, -2.549981878952999992, 320.0000000000000000 ) ) ;
#6796=CARTESIAN_POINT ( 'NONE',  ( 18.85507443398999428, 0.7700411122678003650, 319.9928079742500131 ) ) ;
#6797=CARTESIAN_POINT ( 'NONE',  ( 12.86685525668169561, -9.583295652123236863, -316.5000000000004547 ) ) ;
#6801=CARTESIAN_POINT ( 'NONE',  ( -12.34703828426001770, 8.590819132751997600, -317.4928077629770087 ) ) ;
#6802=CARTESIAN_POINT ( 'NONE',  ( 5.251781279335003383, -11.64703610505998910, -317.5770954168139610 ) ) ;
#6803=CARTESIAN_POINT ( 'NONE',  ( -16.80445917461999983, 3.015803745947999825, -314.4150829855000211 ) ) ;
#6805=CARTESIAN_POINT ( 'NONE',  ( -17.74191744551998795, 5.793625128177000150, -303.6197174156520759 ) ) ;
#6807=CARTESIAN_POINT ( 'NONE',  ( 18.95640219669000004, -0.9217981998336000071, 190.0000000000000000 ) ) ;
#6811=CARTESIAN_POINT ( 'NONE',  ( 18.75323799499002675, -4.519634888734000100, 190.4207385301700128 ) ) ;
#6813=CARTESIAN_POINT ( 'NONE',  ( 17.62731894649998665, -4.091366980619998373, -302.5071922382879279 ) ) ;
#6815=CARTESIAN_POINT ( 'NONE',  ( -14.87873868498998498, 8.458320990069003287, 190.4207385301700128 ) ) ;
#6817=CARTESIAN_POINT ( 'NONE',  ( 13.62823431091000081, -6.408810695481999886, 314.4150829855000211 ) ) ;
#6821=CARTESIAN_POINT ( 'NONE',  ( -9.099181536070998888, -11.22222323403999766, 319.5792614743400009 ) ) ;
#6822=CARTESIAN_POINT ( 'NONE',  ( -16.24773437005479693, 3.756014688789979683, 314.4999406160052331 ) ) ;
#6825=CARTESIAN_POINT ( 'NONE',  ( 16.25556153634000367, 3.885850782616000032, 314.4150829855000211 ) ) ;
#6827=CARTESIAN_POINT ( 'NONE',  ( 9.013443235573840084, -11.16848941897282899, 190.9999999999995737 ) ) ;
#6828=CARTESIAN_POINT ( 'NONE',  ( 20.08924610253000509, 0.07535283344304002928, 319.5792614743400009 ) ) ;
#6831=CARTESIAN_POINT ( 'NONE',  ( 4.252796533868254514, 9.197585063050969012, 315.0000000000000568 ) ) ;
#6832=CARTESIAN_POINT ( 'NONE',  ( -15.00000000000071587, -0.4945770392355663403, -284.9999999999999432 ) ) ;
#6834=DIRECTION ( 'NONE',  ( 1.000000000000000000, 0.000000000000000000, 0.000000000000000000 ) ) ;
#6837=CARTESIAN_POINT ( 'NONE',  ( 12.50247260085999912, 8.641513563414997989, 190.0000000000000000 ) ) ;
#6839=CARTESIAN_POINT ( 'NONE',  ( -14.93050028969001808, 6.935770771621001529, 190.0071920248299477 ) ) ;
#6845=EDGE_LOOP ( 'NONE', ( #4973, #2979, #6719, #3249 ) ) ;
#6847=CARTESIAN_POINT ( 'NONE',  ( -18.54292857607040901, -4.743390938996658868, -316.5000000000004547 ) ) ;
#6852=CARTESIAN_POINT ( 'NONE',  ( -5.133129775586001031, 10.95790389472999316, -317.4928077629770087 ) ) ;
#6853=CARTESIAN_POINT ( 'NONE',  ( -19.37639879579000635, -3.420933338561999548, -317.0792622552969533 ) ) ;
#6854=CARTESIAN_POINT ( 'NONE',  ( -19.00000000000000000, 0.000000000000000000, 319.9999999999899956 ) ) ;
#6855=DIRECTION ( 'NONE',  ( 0.000000000000000000, 0.000000000000000000, -1.000000000000000000 ) ) ;
#6858=CARTESIAN_POINT ( 'NONE',  ( -4.353497780899999725, -11.20674699699000065, 190.0000000000000000 ) ) ;
#6860=CARTESIAN_POINT ( 'NONE',  ( 2.381287040813000348E-07, -10.00000001404999850, 190.0000000000000000 ) ) ;
#6863=CARTESIAN_POINT ( 'NONE',  ( -19.14223954934999483, -3.638712114223002558, 191.1197171614399792 ) ) ;
#6865=CARTESIAN_POINT ( 'NONE',  ( -16.40981772118269788, -2.462276419762760682, 314.9999999999999432 ) ) ;
#6866=CARTESIAN_POINT ( 'NONE',  ( -7.736889024074004695, -10.37866566675000435, -302.5071922382879279 ) ) ;
#6867=CARTESIAN_POINT ( 'NONE',  ( -19.98387668437998954, -0.4031290841194005714, 191.1197171614399792 ) ) ;
#6868=AXIS2_PLACEMENT_3D ( 'NONE', #7435, #10601, #72 ) ;
#6869=ADVANCED_FACE ( 'NONE', ( #3699, #9550 ), #6216, .T. ) ;
#6873=CARTESIAN_POINT ( 'NONE',  ( 18.87259549714001139, -0.3457787829170000937, -302.5071922382879279 ) ) ;
#6874=CARTESIAN_POINT ( 'NONE',  ( -4.941041030666997180, -12.20591504665998350, 319.5792614743400009 ) ) ;
#6876=CARTESIAN_POINT ( 'NONE',  ( -1.399029207469000058, 9.644928263550999858, 314.8616023057000461 ) ) ;
#6878=CARTESIAN_POINT ( 'NONE',  ( -17.64879272652969888, -5.897502810282468921, 190.9999999999995737 ) ) ;
#6880=CARTESIAN_POINT ( 'NONE',  ( 18.27279225368999249, 5.234253896328004529, 319.5792614743400009 ) ) ;
#6882=EDGE_CURVE ( 'NONE', #4012, #8127, #2845, .T. ) ;
#6885=CARTESIAN_POINT ( 'NONE',  ( -1.669669261120717341, 9.454727574740482865, 315.0000000000000568 ) ) ;
#6886=CARTESIAN_POINT ( 'NONE',  ( 0.000000000000000000, -10.00000000000000000, 315.0000000000000000 ) ) ;
#6890=CARTESIAN_POINT ( 'NONE',  ( 18.20814976352000158, 3.283820199526999772, 190.0000000000000000 ) ) ;
#6891=CARTESIAN_POINT ( 'NONE',  ( 14.91207369124052740, -5.270756709766473591, 314.4999413757460047 ) ) ;
#6892=CARTESIAN_POINT ( 'NONE',  ( -11.67891759455000056, 8.922363378240000031, 190.0071920248299477 ) ) ;
#6894=( BOUNDED_CURVE ( )  B_SPLINE_CURVE ( 3, ( #6934, #1333, #5206, #8636, #4612, #8580, #6886 ),
 .UNSPECIFIED., .F., .T. ) 
 B_SPLINE_CURVE_WITH_KNOTS ( ( 4, 3, 4 ),
 ( 0.000000000000000000, 0.5000000000000000000, 1.000000000000000000 ),
 .UNSPECIFIED. ) 
 CURVE ( )  GEOMETRIC_REPRESENTATION_ITEM ( )  RATIONAL_B_SPLINE_CURVE ( ( 1.000000000000000000, 0.8047378516590519837, 0.8047378516590519837, 1.000000000000000000, 0.8047378516590519837, 0.8047378516590519837, 1.000000000000000000 ) ) 
 REPRESENTATION_ITEM ( '' )  );
#6895=CARTESIAN_POINT ( 'NONE',  ( -18.32252861763999974, -3.123808493131999597, -317.4999999999870397 ) ) ;
#6897=CARTESIAN_POINT ( 'NONE',  ( 13.95695539824072640, -5.398716172439862682, 315.0000000000000568 ) ) ;
#6898=CARTESIAN_POINT ( 'NONE',  ( -13.50042001888999899, 6.225262767767000049, -314.6383426456000052 ) ) ;
#6901=CARTESIAN_POINT ( 'NONE',  ( 15.96117728870900088, -7.554047240424474730, -316.5000000000004547 ) ) ;
#6905=CARTESIAN_POINT ( 'NONE',  ( 16.93681971163998057, -6.782628217974004059, -317.0792622552969533 ) ) ;
#6909=CARTESIAN_POINT ( 'NONE',  ( 4.557748955467384455, 9.652551271539412170, -314.5171779026347281 ) ) ;
#6911=CARTESIAN_POINT ( 'NONE',  ( 18.99998114578000141, -0.3144692935366000253, 190.0000000000100044 ) ) ;
#6914=CARTESIAN_POINT ( 'NONE',  ( 13.99304003883001180, -8.933243331610997373, 191.1197171614399792 ) ) ;
#6916=CARTESIAN_POINT ( 'NONE',  ( -16.99953299605537183, -0.4334412736564766666, 315.0000000000000568 ) ) ;
#6917=CARTESIAN_POINT ( 'NONE',  ( -14.28705177277001148, -7.417718350405998251, -302.5071922382879279 ) ) ;
#6924=CARTESIAN_POINT ( 'NONE',  ( -19.97284365803998796, 0.5561741493802002667, 318.8802828394900644 ) ) ;
#6925=CARTESIAN_POINT ( 'NONE',  ( 17.56758064089999749, -0.6313722887073999201, -314.4150829855000211 ) ) ;
#6926=CARTESIAN_POINT ( 'NONE',  ( -15.27200851150000105, 4.387263554753999983, 314.8616023057000461 ) ) ;
#6927=ORIENTED_EDGE ( 'NONE', *, *, #9496, .T. ) ;
#6928=CARTESIAN_POINT ( 'NONE',  ( 4.683335428805002643, -11.03437642965999288, 190.0071920248299477 ) ) ;
#6933=CARTESIAN_POINT ( 'NONE',  ( -14.65007096172560708, 4.807726778454477490, 314.9999999999998863 ) ) ;
#6934=CARTESIAN_POINT ( 'NONE',  ( 0.000000000000000000, 10.00000000000000000, 315.0000000000000000 ) ) ;
#6935=CARTESIAN_POINT ( 'NONE',  ( -12.75178873474799168, -6.273979344207467612, -314.9999999999999432 ) ) ;
#6941=CARTESIAN_POINT ( 'NONE',  ( -11.76997148278789673, 6.834709328092291258, -315.0000000000000000 ) ) ;
#6942=CARTESIAN_POINT ( 'NONE',  ( -4.683335428805002643, 11.03437642965999288, 190.0071920248299477 ) ) ;
#6951=CARTESIAN_POINT ( 'NONE',  ( 4.298491262593391760, -9.188587546143761386, 314.9999999999999432 ) ) ;
#6952=CARTESIAN_POINT ( 'NONE',  ( -14.72449281369000040, 5.549439731021000632, -314.4150829855000211 ) ) ;
#6955=CARTESIAN_POINT ( 'NONE',  ( -14.12295497348999440, 7.525186449763000773, 319.9928079742500131 ) ) ;
#6961=CARTESIAN_POINT ( 'NONE',  ( -17.77555462084998794, -5.884850558328997394, -317.0792622552969533 ) ) ;
#6963=CARTESIAN_POINT ( 'NONE',  ( 13.47608353327720643, 6.291341891605557457, -314.5797986957608714 ) ) ;
#6965=CARTESIAN_POINT ( 'NONE',  ( 7.592156631695000435, -10.54118908926000131, 190.0000000000000000 ) ) ;
#6966=CARTESIAN_POINT ( 'NONE',  ( -19.14895805910627757, -3.641352296147344791, 319.0000000000003979 ) ) ;
#6969=CARTESIAN_POINT ( 'NONE',  ( 11.16929996816999804, -10.37059603288001419, 191.1197171614399792 ) ) ;
#6972=CARTESIAN_POINT ( 'NONE',  ( -16.06615879071999231, -5.957812395457000143, -302.5071922382879279 ) ) ;
#6977=( BOUNDED_CURVE ( )  B_SPLINE_CURVE ( 3, ( #6860, #6145, #9432, #8668 ),
 .UNSPECIFIED., .F., .T. ) 
 B_SPLINE_CURVE_WITH_KNOTS ( ( 4, 4 ),
 ( 0.000000000000000000, 1.000000000000000000 ),
 .UNSPECIFIED. ) 
 CURVE ( )  GEOMETRIC_REPRESENTATION_ITEM ( )  RATIONAL_B_SPLINE_CURVE ( ( 1.000000000000000000, 0.8029010325775971513, 0.8003084355045908538, 0.9922222087809807745 ) ) 
 REPRESENTATION_ITEM ( '' )  );
#6978=CARTESIAN_POINT ( 'NONE',  ( -17.62731894649998665, 4.091366980619998373, -302.5071922382879279 ) ) ;
#6979=CARTESIAN_POINT ( 'NONE',  ( 9.940815099545000422, -10.93780185275999983, 319.5792614743400009 ) ) ;
#6980=CARTESIAN_POINT ( 'NONE',  ( 16.80445917461999983, -3.015803745947999825, -314.4150829855000211 ) ) ;
#6981=CARTESIAN_POINT ( 'NONE',  ( -3.971626792229000280, 9.186906450543000702, 315.0848619657999734 ) ) ;
#6983=CARTESIAN_POINT ( 'NONE',  ( 13.41272981818000432, -7.983430642947998201, 190.0071920248299477 ) ) ;
#6984=CARTESIAN_POINT ( 'NONE',  ( -16.30476707551000359, 7.243228625700997902, 318.8802828394900644 ) ) ;
#6986=EDGE_CURVE ( 'NONE', #10485, #1864, #6376, .T. ) ;
#6990=CARTESIAN_POINT ( 'NONE',  ( -11.69624556101560664, -6.874206995516637164, -315.0000000000000000 ) ) ;
#6991=CARTESIAN_POINT ( 'NONE',  ( 20.00000000000000000, 0.000000000000000000, 319.0000000000000000 ) ) ;
#6993=CARTESIAN_POINT ( 'NONE',  ( -3.713614856666575144E-09, 12.50000000000000000, -303.5000000000000000 ) ) ;
#6994=CARTESIAN_POINT ( 'NONE',  ( -8.778856717165009371, 8.123403389731517876, -315.0000000000001137 ) ) ;
#6996=CARTESIAN_POINT ( 'NONE',  ( -3.019104878445999063, 11.24894423506000152, 190.0071920248299477 ) ) ;
#7003=CARTESIAN_POINT ( 'NONE',  ( 3.309867371927075919, -9.320876041153052682, 315.0000000000000568 ) ) ;
#7004=CARTESIAN_POINT ( 'NONE',  ( -12.28828818102000042, 7.249309191407999897, -314.4150829855000211 ) ) ;
#7010=CARTESIAN_POINT ( 'NONE',  ( -14.32792941690000177, 7.389020440446000926, -317.4928077629770087 ) ) ;
#7011=CARTESIAN_POINT ( 'NONE',  ( -3.365463313584999838, -12.41489380075000604, -317.0792622552969533 ) ) ;
#7015=CARTESIAN_POINT ( 'NONE',  ( -10.00000000000000000, 2.500000000000000000, -317.5000000000000000 ) ) ;
#7017=CARTESIAN_POINT ( 'NONE',  ( -17.81342281586000098, -3.988456401492999959, 190.0000000000000000 ) ) ;
#7018=LINE ( 'NONE', #5333, #2140 ) ;
#7020=CARTESIAN_POINT ( 'NONE',  ( -17.64332610462000872, -5.892819363352002959, 191.1197171614399792 ) ) ;
#7021=EDGE_LOOP ( 'NONE', ( #9713, #633, #6480, #3493 ) ) ;
#7022=CARTESIAN_POINT ( 'NONE',  ( -17.50000000088854435, -5.867334121986941042, -302.5000000000002842 ) ) ;
#7023=CARTESIAN_POINT ( 'NONE',  ( -15.21156667173000621, -6.719223644262998008, -302.5071922382879279 ) ) ;
#7028=CARTESIAN_POINT ( 'NONE',  ( -15.25170542629001602, 6.686182281419003282, -302.5071922382879279 ) ) ;
#7029=CARTESIAN_POINT ( 'NONE',  ( -15.65693014362998348, -7.780815921226000853, 318.8802828394900644 ) ) ;
#7030=CARTESIAN_POINT ( 'NONE',  ( 15.60185585328000002, -4.689707898928999974, -314.4150829855000211 ) ) ;
#7031=CARTESIAN_POINT ( 'NONE',  ( -16.77957632114000219, 1.244976636274000015, 315.0848619657999734 ) ) ;
#7033=CARTESIAN_POINT ( 'NONE',  ( 3.019104878445999063, -11.24894423506000152, 190.0071920248299477 ) ) ;
#7038=CARTESIAN_POINT ( 'NONE',  ( -16.90189876424999937, 0.3838616842170000099, 315.0848619657999734 ) ) ;
#7043=CARTESIAN_POINT ( 'NONE',  ( -11.54764063961475351, -6.952680983979390383, -315.0000000000000000 ) ) ;
#7045=CARTESIAN_POINT ( 'NONE',  ( 17.16661504264608951, -5.088157148453773714E-08, 314.8332817084516364 ) ) ;
#7047=CARTESIAN_POINT ( 'NONE',  ( 6.369817261971415512, 8.818538635844451079, -315.0000000000000000 ) ) ;
#7048=CARTESIAN_POINT ( 'NONE',  ( 12.81613682183999536, 9.130924732858002102, 189.9229057364800042 ) ) ;
#7057=CARTESIAN_POINT ( 'NONE',  ( 8.096811247556559010, -8.344189070382460827, 315.0000000000001137 ) ) ;
#7058=CARTESIAN_POINT ( 'NONE',  ( -6.438474686349000997, 8.964777275824999947, -314.8616023057000461 ) ) ;
#7060=CARTESIAN_POINT ( 'NONE',  ( 16.74680747859001784, 6.256295688540001620, 320.0770942683900557 ) ) ;
#7064=CARTESIAN_POINT ( 'NONE',  ( 3.312898553962003056, 11.91959439673999199, -317.5770954168139610 ) ) ;
#7065=CARTESIAN_POINT ( 'NONE',  ( -16.55682536756000545, -6.456981081556999236, -317.5770954168139610 ) ) ;
#7071=CARTESIAN_POINT ( 'NONE',  ( 6.040317665795909008, -11.93081507280030884, 319.0000000000003979 ) ) ;
#7073=CARTESIAN_POINT ( 'NONE',  ( -19.98293839508998104, 0.4162045188174002819, 191.1197171614399792 ) ) ;
#7075=CARTESIAN_POINT ( 'NONE',  ( -16.99996037728000076, 1.352916227065999958E-09, 314.9999801883000146 ) ) ;
#7076=CARTESIAN_POINT ( 'NONE',  ( -14.68756396110000395, -7.991310926523999214, -302.4229045757450081 ) ) ;
#7082=CARTESIAN_POINT ( 'NONE',  ( 18.91993355959997558, 3.215835268190998075, -302.4229045757450081 ) ) ;
#7085=VECTOR ( 'NONE', #1640, 1000.000000000000000 ) ;
#7086=CARTESIAN_POINT ( 'NONE',  ( -8.450675645183000739, -8.177559542660000957, -315.0848619657999734 ) ) ;
#7087=CARTESIAN_POINT ( 'NONE',  ( -12.07130791617000121, 6.858215270785999351, 314.8616023057000461 ) ) ;
#7090=CARTESIAN_POINT ( 'NONE',  ( 17.27977314787002427, -4.562413721234999109, 190.0071920248299477 ) ) ;
#7096=CARTESIAN_POINT ( 'NONE',  ( 13.57573464316000056, -3.225916527208000151, 315.0000000000001705 ) ) ;
#7097=CARTESIAN_POINT ( 'NONE',  ( -15.06645494800451068, -4.378519400638149150, -315.0000000000000568 ) ) ;
#7100=CARTESIAN_POINT ( 'NONE',  ( -11.78094678683302376, 6.828785851005065410, -315.0000000000000000 ) ) ;
#7101=CARTESIAN_POINT ( 'NONE',  ( -16.71231899867997583, 6.291214601299001785, 189.9229057364800042 ) ) ;
#7102=CARTESIAN_POINT ( 'NONE',  ( 5.453091995311539542, 9.512452488116691640, 314.4999455543127738 ) ) ;
#7103=CARTESIAN_POINT ( 'NONE',  ( 6.537962633339999385, -10.80030782989000038, -317.5000000000000000 ) ) ;
#7106=CARTESIAN_POINT ( 'NONE',  ( 15.35630118782766651, -4.050343336346089451, 315.0000000000000000 ) ) ;
#7107=CARTESIAN_POINT ( 'NONE',  ( 11.89238025184999792, 6.701939844102000166, -315.0848619657999734 ) ) ;
#7108=FACE_OUTER_BOUND ( 'NONE', #10386, .T. ) ;
#7109=CARTESIAN_POINT ( 'NONE',  ( -17.84276444133998041, 4.978015457891998174, 320.0770942683900557 ) ) ;
#7114=CARTESIAN_POINT ( 'NONE',  ( -15.69339834701000136, 7.228928788388996551, -317.5770954168139610 ) ) ;
#7115=CARTESIAN_POINT ( 'NONE',  ( -10.46141074968000062, -10.65879569097000079, -316.3802825947000201 ) ) ;
#7117=CARTESIAN_POINT ( 'NONE',  ( 19.99999035944999903, -7.277437094418000096E-10, -303.5000000000000000 ) ) ;
#7124=CARTESIAN_POINT ( 'NONE',  ( -19.00000000000000000, 0.000000000000000000, -317.4999999998989892 ) ) ;
#7126=CARTESIAN_POINT ( 'NONE',  ( -11.77008734995756178, -6.834641529527616832, 315.0000000000000568 ) ) ;
#7127=CARTESIAN_POINT ( 'NONE',  ( 19.60208457603997090, -0.3236162399036999759, -302.4229045757450081 ) ) ;
#7128=CARTESIAN_POINT ( 'NONE',  ( 9.971838575284008854, 10.83713921150001447, 191.1197171614399792 ) ) ;
#7130=CARTESIAN_POINT ( 'NONE',  ( -14.73495828939998731, 7.957952820716998055, -302.4229045757450081 ) ) ;
#7131=CARTESIAN_POINT ( 'NONE',  ( 0.6337574957234999307, -12.50712592802002021, 318.8802828394900644 ) ) ;
#7133=CARTESIAN_POINT ( 'NONE',  ( -14.52969073417999901, -5.422537850045999974, -314.6383426456000052 ) ) ;
#7136=ORIENTED_EDGE ( 'NONE', *, *, #5162, .F. ) ;
#7137=CARTESIAN_POINT ( 'NONE',  ( -19.11670425725001010, -2.646693943201001264, 189.9229057364800042 ) ) ;
#7138=CARTESIAN_POINT ( 'NONE',  ( -11.17208682466014302, 10.37722895585535809, 190.9999999999996589 ) ) ;
#7139=CARTESIAN_POINT ( 'NONE',  ( 10.00000000000000000, -2.500000000000000000, -285.0000000000000000 ) ) ;
#7141=CARTESIAN_POINT ( 'NONE',  ( -16.07469914181999826, -3.754035329064000059, 314.6383426456000052 ) ) ;
#7143=CARTESIAN_POINT ( 'NONE',  ( -16.47320456655591059, 2.338720490045835820, 314.9999999999999432 ) ) ;
#7144=CARTESIAN_POINT ( 'NONE',  ( -17.42228208267999889, -1.444224815522999972, 314.4150829855000211 ) ) ;
#7145=CARTESIAN_POINT ( 'NONE',  ( -16.13978190921855216, -2.966266463780214302, -315.0000000000000000 ) ) ;
#7150=CARTESIAN_POINT ( 'NONE',  ( -8.717693564518029348, 8.144027366771089405, -314.9999999999999432 ) ) ;
#7151=CARTESIAN_POINT ( 'NONE',  ( -18.24410766404003326, 5.273389473771006308, 190.4207385301700128 ) ) ;
#7152=CARTESIAN_POINT ( 'NONE',  ( 8.203499347305186262, 8.842483610386494775, 314.4999460608030404 ) ) ;
#7153=CARTESIAN_POINT ( 'NONE',  ( -11.71572875140193837, -12.50000000114647847, -316.5000000000000000 ) ) ;
#7157=CARTESIAN_POINT ( 'NONE',  ( 16.95904175860000151, 2.156867278632000229, -314.6383426456000052 ) ) ;
#7159=CARTESIAN_POINT ( 'NONE',  ( -8.650961417647998530, 10.84061383582999838, 320.0770942683900557 ) ) ;
#7163=CARTESIAN_POINT ( 'NONE',  ( -12.67153153313999070, 9.210367834107003659, -317.5770954168139610 ) ) ;
#7164=CARTESIAN_POINT ( 'NONE',  ( -3.356563794682998925, -12.33103673683000423, -316.3802825947000201 ) ) ;
#7169=CARTESIAN_POINT ( 'NONE',  ( -11.51453371961019556, 7.479120141997829485, -314.5676927934668470 ) ) ;
#7174=CARTESIAN_POINT ( 'NONE',  ( -6.752884998590674925, 11.77766676623698139, -316.5000000000004547 ) ) ;
#7176=CARTESIAN_POINT ( 'NONE',  ( -5.850395566949658566, -8.918560297860793185, 315.0000000000000000 ) ) ;
#7177=CARTESIAN_POINT ( 'NONE',  ( -9.338997116452000924, -11.14661793222000519, -302.9207377450070453 ) ) ;
#7181=EDGE_CURVE ( 'NONE', #4512, #1396, #5676, .T. ) ;
#7182=CARTESIAN_POINT ( 'NONE',  ( 6.596975511883001353, 11.38119116100000028, -302.4229045757450081 ) ) ;
#7183=CARTESIAN_POINT ( 'NONE',  ( -7.846787046322997838, -11.50147725199999371, 318.8802828394900644 ) ) ;
#7185=CARTESIAN_POINT ( 'NONE',  ( -3.874983216044999956, -9.425407904674999671, -314.8616023057000461 ) ) ;
#7186=CARTESIAN_POINT ( 'NONE',  ( 16.89041368998000081, 5.257268626091000208, -302.5000000000009663 ) ) ;
#7188=CARTESIAN_POINT ( 'NONE',  ( -11.86325706386000434, -9.609314883874001012, 189.9229057364800042 ) ) ;
#7189=CARTESIAN_POINT ( 'NONE',  ( -9.013443235573840084, 11.16848941897283076, 190.9999999999996589 ) ) ;
#7194=CARTESIAN_POINT ( 'NONE',  ( -10.58801790939999954, -8.088125079530000150, 314.4150829855000211 ) ) ;
#7195=CARTESIAN_POINT ( 'NONE',  ( -18.78787853991000034, 1.761062637770999917, 320.0000000000000000 ) ) ;
#7196=CARTESIAN_POINT ( 'NONE',  ( 4.237945188771000460, -11.10223611999999704, 319.9928079742500131 ) ) ;
#7197=CARTESIAN_POINT ( 'NONE',  ( -17.61684826078804988, 5.934684944789588634, 319.0000000000005116 ) ) ;
#7198=CARTESIAN_POINT ( 'NONE',  ( 10.23467949614886763, -10.00000000050611781, -302.4999999999996021 ) ) ;
#7200=ORIENTED_EDGE ( 'NONE', *, *, #9836, .T. ) ;
#7202=VECTOR ( 'NONE', #923, 1000.000000000000000 ) ;
#7204=CARTESIAN_POINT ( 'NONE',  ( 15.34534221234999585, 7.499749350177997265, 189.9229057364800042 ) ) ;
#7209=CARTESIAN_POINT ( 'NONE',  ( 15.60753896450557221, 3.741771784933492828, 315.0000000000000568 ) ) ;
#7212=CARTESIAN_POINT ( 'NONE',  ( -19.00000000000000000, 0.000000000000000000, -302.5000000001010108 ) ) ;
#7214=CARTESIAN_POINT ( 'NONE',  ( 1.310287062331999319, 12.07175205226999815, 320.0770942683900557 ) ) ;
#7217=EDGE_LOOP ( 'NONE', ( #448, #5621, #6212, #455 ) ) ;
#7218=CARTESIAN_POINT ( 'NONE',  ( 6.380917221297004005, 11.42904134337998734, -317.5770954168139610 ) ) ;
#7220=CARTESIAN_POINT ( 'NONE',  ( -16.84537440012000786, -6.754000406595005224, -316.3802825947000201 ) ) ;
#7222=CARTESIAN_POINT ( 'NONE',  ( 10.58225433500999912, -9.538747186136999900, 320.0000000000000000 ) ) ;
#7225=CARTESIAN_POINT ( 'NONE',  ( -7.237892782308162687, 9.087442202657104673, -314.5335583295244533 ) ) ;
#7227=CARTESIAN_POINT ( 'NONE',  ( 11.98824862436842409, -10.01561519341996132, 319.0000000000003979 ) ) ;
#7231=CARTESIAN_POINT ( 'NONE',  ( -11.84516230667378345, -6.793967159201454997, 315.0000000000000568 ) ) ;
#7232=CARTESIAN_POINT ( 'NONE',  ( 3.382256884648001893, -11.91212135210998824, -302.4229045757450081 ) ) ;
#7234=CARTESIAN_POINT ( 'NONE',  ( 7.006889269069000115, -6.844138725329000472, 315.0000000000000000 ) ) ;
#7235=CARTESIAN_POINT ( 'NONE',  ( -7.947966332010000023, 11.56278913298000077, -302.9207377450070453 ) ) ;
#7236=CARTESIAN_POINT ( 'NONE',  ( 16.30476707551000359, -7.243228625700997902, 318.8802828394900644 ) ) ;
#7238=CARTESIAN_POINT ( 'NONE',  ( 1.399029207469000058, -9.644928263550999858, -314.8616023057000461 ) ) ;
#7241=CARTESIAN_POINT ( 'NONE',  ( -14.56080423438999993, -8.072998568875000558, 189.9229057364800042 ) ) ;
#7242=CARTESIAN_POINT ( 'NONE',  ( -1.249193831065315452, 12.49557363514548491, 190.9999999999996589 ) ) ;
#7246=CARTESIAN_POINT ( 'NONE',  ( -16.25556153634000367, -3.885850782616000032, 314.4150829855000211 ) ) ;
#7248=CARTESIAN_POINT ( 'NONE',  ( 3.142739053800999827, 11.35686622240999810, 320.0000000000000000 ) ) ;
#7249=CARTESIAN_POINT ( 'NONE',  ( 13.31009360926000085, -8.046300872832002682, 319.9928079742500131 ) ) ;
#7255=CARTESIAN_POINT ( 'NONE',  ( 7.006889269069000115, 6.844138725329000472, -285.0000000000000000 ) ) ;
#7257=CARTESIAN_POINT ( 'NONE',  ( -11.00905209676000140, 9.989194338198000622, 189.9229057364800042 ) ) ;
#7260=CARTESIAN_POINT ( 'NONE',  ( -11.71572875140193837, -12.50000000114647847, -303.4999999999999432 ) ) ;
#7261=CARTESIAN_POINT ( 'NONE',  ( 16.39045651208371979, 2.501479531468998818, 315.0000000000000000 ) ) ;
#7263=CARTESIAN_POINT ( 'NONE',  ( -19.30523607465251956, -3.390426274888738156, -303.5000000000006253 ) ) ;
#7264=CARTESIAN_POINT ( 'NONE',  ( 16.25556153634000367, 3.885850782616000032, -314.4150829855000211 ) ) ;
#7266=CARTESIAN_POINT ( 'NONE',  ( -10.81481884307000207, 10.07000335707000538, 320.0770942683900557 ) ) ;
#7267=CARTESIAN_POINT ( 'NONE',  ( 10.00000000000000000, 2.500000000000000000, -285.0000000000000000 ) ) ;
#7271=CARTESIAN_POINT ( 'NONE',  ( 11.66516470684000772, 10.15894662545001381, -316.3802825947000201 ) ) ;
#7272=CARTESIAN_POINT ( 'NONE',  ( -19.86719273998999213, -1.743644188460999667, -316.3802825947000201 ) ) ;
#7274=CARTESIAN_POINT ( 'NONE',  ( -15.00000000000000000, 0.000000000000000000, -285.0000000000000000 ) ) ;
#7280=CARTESIAN_POINT ( 'NONE',  ( -1.327715439883788706, -12.49239253839650843, 319.0000000000003979 ) ) ;
#7284=CARTESIAN_POINT ( 'NONE',  ( -8.778709539581399213, -8.123450746681353252, 315.0000000000000000 ) ) ;
#7285=CARTESIAN_POINT ( 'NONE',  ( 18.21470573400001669, -4.474143576597000127, -302.4229045757450081 ) ) ;
#7290=SURFACE_STYLE_USAGE ( .BOTH. , #8089 ) ;
#7291=CARTESIAN_POINT ( 'NONE',  ( -13.72185241754999652, 8.618935511841003816, -302.4229045757450081 ) ) ;
#7294=ORIENTED_EDGE ( 'NONE', *, *, #1550, .T. ) ;
#7295=CARTESIAN_POINT ( 'NONE',  ( 10.40890489166000066, -7.434429060800999522, -315.0848619657999734 ) ) ;
#7297=VERTEX_POINT ( 'NONE', #4908 ) ;
#7298=CARTESIAN_POINT ( 'NONE',  ( -16.73002466287002576, -6.274001814427998980, 189.9229057364800042 ) ) ;
#7299=CARTESIAN_POINT ( 'NONE',  ( 17.02940347669788324, 6.570098831661549177, 190.9999999999996589 ) ) ;
#7303=CARTESIAN_POINT ( 'NONE',  ( -14.38384290288000145, -5.252906928686999599, 314.8616023057000461 ) ) ;
#7304=CARTESIAN_POINT ( 'NONE',  ( -9.597846547914999249, 9.915773017694000657, 320.0000000000000000 ) ) ;
#7307=CARTESIAN_POINT ( 'NONE',  ( 17.49999999911143433, -5.867334123717693473, -302.4999999999996021 ) ) ;
#7316=CARTESIAN_POINT ( 'NONE',  ( 11.80673610560780240, 6.814824988023822527, 315.0000000000000000 ) ) ;
#7318=CARTESIAN_POINT ( 'NONE',  ( -19.99984324442397465, -0.5882482212486090933, -303.4999999999997158 ) ) ;
#7319=CARTESIAN_POINT ( 'NONE',  ( 17.56970546055000071, -0.4338786413876999926, -314.4150829855000211 ) ) ;
#7321=CARTESIAN_POINT ( 'NONE',  ( 15.65693014362998348, 7.780815921226000853, 318.8802828394900644 ) ) ;
#7322=DIRECTION ( 'NONE',  ( 0.000000000000000000, -1.000000000000000000, 0.000000000000000000 ) ) ;
#7325=CARTESIAN_POINT ( 'NONE',  ( 14.92964316144998627, 8.327009966606000901, -316.3802825947000201 ) ) ;
#7328=LINE ( 'NONE', #7274, #10088 ) ;
#7331=CARTESIAN_POINT ( 'NONE',  ( -16.63862268811586986, 3.034640078201995994, -314.5459747968306488 ) ) ;
#7333=CARTESIAN_POINT ( 'NONE',  ( -3.650011388878885210, -9.782272988550902326, -314.5118284007355669 ) ) ;
#7335=CARTESIAN_POINT ( 'NONE',  ( -7.807700195763000117, 10.48319479899000051, -317.5000000000000000 ) ) ;
#7336=ORIENTED_EDGE ( 'NONE', *, *, #2869, .F. ) ;
#7337=CARTESIAN_POINT ( 'NONE',  ( 14.97309261602000419, -8.296494983500004139, -303.6197174156509391 ) ) ;
#7338=CARTESIAN_POINT ( 'NONE',  ( 19.99999721132999753, -3.518697978483000342E-10, 319.0000000000000000 ) ) ;
#7342=SHAPE_REPRESENTATION_RELATIONSHIP ( 'NONE' , 'NONE' ,  #1806, #453 ) ;
#7343=CARTESIAN_POINT ( 'NONE',  ( 9.183684135703998663, 10.67340332910999834, -302.4229045757450081 ) ) ;
#7344=CARTESIAN_POINT ( 'NONE',  ( -10.25126250535807770, -10.00000007971003058, 314.9999999999999432 ) ) ;
#7346=CARTESIAN_POINT ( 'NONE',  ( -17.57772697299999720, 0.3191603157329000462, -314.4150829855000211 ) ) ;
#7349=CARTESIAN_POINT ( 'NONE',  ( 13.77732760571000092, -8.580179748050001720, 189.9229057364800042 ) ) ;
#7352=CARTESIAN_POINT ( 'NONE',  ( 14.65054575295525119, 4.807282645526345100, -315.0000000000001137 ) ) ;
#7353=DIRECTION ( 'NONE',  ( 1.000000000000000000, 0.000000000000000000, 0.000000000000000000 ) ) ;
#7354=CARTESIAN_POINT ( 'NONE',  ( -15.23514566747999943, -4.427644513407000382, 314.8616023057000461 ) ) ;
#7355=CARTESIAN_POINT ( 'NONE',  ( -0.6600210488075000104, 11.51366633668999917, 320.0000000000000000 ) ) ;
#7357=CARTESIAN_POINT ( 'NONE',  ( -14.75365836417945431, 8.451130538707893436, 319.0000000000005116 ) ) ;
#7360=ORIENTED_EDGE ( 'NONE', *, *, #9425, .F. ) ;
#7361=CARTESIAN_POINT ( 'NONE',  ( -13.57573464316000056, 3.225916527208000151, -285.0000000000000000 ) ) ;
#7366=CARTESIAN_POINT ( 'NONE',  ( 7.927914882803702490, -11.48831374418035089, -303.4999999999996589 ) ) ;
#7374=ORIENTED_EDGE ( 'NONE', *, *, #6882, .F. ) ;
#7375=CARTESIAN_POINT ( 'NONE',  ( 4.990336260259995882, 12.19640393417999036, -317.0792622552969533 ) ) ;
#7380=CARTESIAN_POINT ( 'NONE',  ( -3.142739053800999827, -11.35686622240999810, 320.0000000000000000 ) ) ;
#7384=CARTESIAN_POINT ( 'NONE',  ( 15.48916725177958398, -3.890278845006962083, -315.0000000000000000 ) ) ;
#7385=ORIENTED_EDGE ( 'NONE', *, *, #4237, .F. ) ;
#7386=CARTESIAN_POINT ( 'NONE',  ( -15.67978886374999803, 4.575336738469999887, -315.0000000000001137 ) ) ;
#7388=CARTESIAN_POINT ( 'NONE',  ( -10.00000000000000000, 2.500000000000000000, -315.0000000000000000 ) ) ;
#7390=CARTESIAN_POINT ( 'NONE',  ( -15.91674550148000122, -7.581266318323002906, -303.6197174156509391 ) ) ;
#7396=CARTESIAN_POINT ( 'NONE',  ( -11.71875184657000091, 10.13482718352000944, -303.6197174156509391 ) ) ;
#7398=CARTESIAN_POINT ( 'NONE',  ( -16.39086977655999888, -2.839079766962000040, -314.8616023057000461 ) ) ;
#7401=CARTESIAN_POINT ( 'NONE',  ( 14.03700484701000484, -9.005201968871000773, 190.4207385301700128 ) ) ;
#7402=CARTESIAN_POINT ( 'NONE',  ( -17.50000000000107292, -0.7437989020622546299, -314.4944826805095772 ) ) ;
#7403=CARTESIAN_POINT ( 'NONE',  ( 15.63394123731325358, 3.714777356940325070, -314.9999999999999432 ) ) ;
#7405=VECTOR ( 'NONE', #7322, 1000.000000000000000 ) ;
#7406=CARTESIAN_POINT ( 'NONE',  ( 8.620760283086999820, -8.357092890497000326, 314.8616023057000461 ) ) ;
#7408=CARTESIAN_POINT ( 'NONE',  ( 2.538616493050997569, -11.99586634586999523, 320.0770942683900557 ) ) ;
#7409=CARTESIAN_POINT ( 'NONE',  ( 19.14895805910628468, 3.641352296147347012, 319.0000000000005116 ) ) ;
#7410=CARTESIAN_POINT ( 'NONE',  ( 15.92130416703352580, 7.586839038430810866, -303.5000000000000000 ) ) ;
#7411=CARTESIAN_POINT ( 'NONE',  ( 17.34089965840999881, 0.6440164457022999889, 314.6383426456000052 ) ) ;
#7417=CARTESIAN_POINT ( 'NONE',  ( -19.00000000000000000, 0.000000000000000000, -302.5000000001010108 ) ) ;
#7428=CARTESIAN_POINT ( 'NONE',  ( -14.79012398734008293, 1.483731117706880154, -284.9999999999999432 ) ) ;
#7430=CARTESIAN_POINT ( 'NONE',  ( -20.01697452336999561, 0.3413909698088000710, -316.3802825947000201 ) ) ;
#7435=CARTESIAN_POINT ( 'NONE',  ( 18.99997865338999858, -1.260542273207000211E-06, -316.5000000000000000 ) ) ;
#7436=CARTESIAN_POINT ( 'NONE',  ( 11.78094678683302554, -6.828785851005064522, -315.0000000000000568 ) ) ;
#7438=CARTESIAN_POINT ( 'NONE',  ( -1.831806507035719234, -9.955740905498862148, -314.5031779949863449 ) ) ;
#7439=ORIENTED_EDGE ( 'NONE', *, *, #4899, .F. ) ;
#7440=CARTESIAN_POINT ( 'NONE',  ( -2.034678270035999770, 11.44985799554000039, -317.5000000000000000 ) ) ;
#7442=CARTESIAN_POINT ( 'NONE',  ( -8.030503796230000546, -11.45221762926000153, -303.6197174156509391 ) ) ;
#7444=CARTESIAN_POINT ( 'NONE',  ( 15.00000000000000000, -0.4945770392355999800, 315.0000000000000000 ) ) ;
#7445=CARTESIAN_POINT ( 'NONE',  ( -16.88084019735002173, 6.719348373024005561, -303.6197174156509391 ) ) ;
#7446=CARTESIAN_POINT ( 'NONE',  ( -17.50000000000000000, -3.147917160613439321E-08, 314.4997059534069308 ) ) ;
#7451=CARTESIAN_POINT ( 'NONE',  ( 19.12235363464000670, -3.679291565416002108, 191.1197171614399792 ) ) ;
#7455=CARTESIAN_POINT ( 'NONE',  ( 16.39938580555998726, 7.272241081627004000, 190.4207385301700128 ) ) ;
#7459=CARTESIAN_POINT ( 'NONE',  ( 17.56954514911999965, 0.4333932196220000033, 314.4150829855000211 ) ) ;
#7461=CARTESIAN_POINT ( 'NONE',  ( 15.00000000000000000, 0.000000000000000000, -285.0000000000000000 ) ) ;
#7462=CARTESIAN_POINT ( 'NONE',  ( 15.57034186525998543, -6.406527364046002759, 319.9928079742500131 ) ) ;
#7463=CARTESIAN_POINT ( 'NONE',  ( -12.89381003144900184, 6.798165335629914097, 314.4999421354863216 ) ) ;
#7464=CARTESIAN_POINT ( 'NONE',  ( 17.57772697299999720, -0.3191603157329000462, 314.4150829855000211 ) ) ;
#7466=CARTESIAN_POINT ( 'NONE',  ( 17.62182611535273935, -5.928443937941890063, 190.9999999999995737 ) ) ;
#7468=ORIENTED_EDGE ( 'NONE', *, *, #8088, .T. ) ;
#7470=ADVANCED_FACE ( 'NONE', ( #10490, #4103 ), #3192, .T. ) ;
#7473=CARTESIAN_POINT ( 'NONE',  ( -11.69610966801475449, 6.874282731906364852, 315.0000000000000000 ) ) ;
#7477=CARTESIAN_POINT ( 'NONE',  ( 7.649658656166000270, -10.52693506402999901, -302.5000000000000000 ) ) ;
#7479=CARTESIAN_POINT ( 'NONE',  ( 0.6643694614233000006, 11.51357945830000062, 190.0000000000000000 ) ) ;
#7482=CARTESIAN_POINT ( 'NONE',  ( 17.49999012170142620, -5.867339742191236773, 190.0000000000003695 ) ) ;
#7483=CARTESIAN_POINT ( 'NONE',  ( -2.060812052271002059, 12.52766984582000021, -317.0792622552969533 ) ) ;
#7488=LINE ( 'NONE', #5922, #796 ) ;
#7489=CARTESIAN_POINT ( 'NONE',  ( 16.37160231057345428, -2.539265572400264404, -315.0000000000000000 ) ) ;
#7491=CARTESIAN_POINT ( 'NONE',  ( 8.988119689606872242, -8.550792887852699309, -314.5455502384735951 ) ) ;
#7493=CARTESIAN_POINT ( 'NONE',  ( 3.336936413097000287, 11.33398029193999967, -317.5000000000000000 ) ) ;
#7495=CARTESIAN_POINT ( 'NONE',  ( -9.312701725069002734, -11.06649994634999246, -303.6197174156509391 ) ) ;
#7496=CARTESIAN_POINT ( 'NONE',  ( 18.29581373626999508, -2.889895519923001643, -317.4928077629770087 ) ) ;
#7497=CARTESIAN_POINT ( 'NONE',  ( -17.12432750374000179, -0.4000877216259000058, -314.8616023057000461 ) ) ;
#7499=CARTESIAN_POINT ( 'NONE',  ( 19.29864983862999850, 3.387441872937999143, -303.6197174156509391 ) ) ;
#7504=ORIENTED_EDGE ( 'NONE', *, *, #1909, .F. ) ;
#7505=CARTESIAN_POINT ( 'NONE',  ( 19.49006540358000805, -2.831553480999998929, 191.1197171614399792 ) ) ;
#7506=CARTESIAN_POINT ( 'NONE',  ( 8.037373804805000077, -9.179324345868998591, -314.4944826805095772 ) ) ;
#7507=CARTESIAN_POINT ( 'NONE',  ( 15.40306756913855146, 3.994766537461135858, -314.9999999999998863 ) ) ;
#7509=CARTESIAN_POINT ( 'NONE',  ( -10.15702342499999844, 10.85948264422000165, 190.4207385301700128 ) ) ;
#7510=EDGE_CURVE ( 'NONE', #7297, #9430, #8221, .T. ) ;
#7511=CARTESIAN_POINT ( 'NONE',  ( 16.90171868104999930, 0.3834349726278000192, 315.0848619657999734 ) ) ;
#7513=CARTESIAN_POINT ( 'NONE',  ( -19.56036306585002293, 0.5267516669946002983, 320.0770942683900557 ) ) ;
#7515=CARTESIAN_POINT ( 'NONE',  ( 16.07469914181999826, 3.754035329064000059, 314.6383426456000052 ) ) ;
#7518=CARTESIAN_POINT ( 'NONE',  ( -11.00353245304999739, 10.53087951318999593, 319.5792614743400009 ) ) ;
#7521=EDGE_CURVE ( 'NONE', #3286, #2509, #10122, .T. ) ;
#7523=CARTESIAN_POINT ( 'NONE',  ( -12.16656789651012005, 6.621481216618937182, 314.9999999999999432 ) ) ;
#7527=CARTESIAN_POINT ( 'NONE',  ( 19.00000000000000000, 0.000000000000000000, -302.5000000001010108 ) ) ;
#7530=CARTESIAN_POINT ( 'NONE',  ( 17.50000000000002487, 1.995060298004523415E-08, 314.4999385900306947 ) ) ;
#7538=CARTESIAN_POINT ( 'NONE',  ( 11.80659750965543608, -6.814906413124091067, -314.9999999999999432 ) ) ;
#7540=CARTESIAN_POINT ( 'NONE',  ( 12.32405526929588113, -7.045528031251313550, -314.5741454722275421 ) ) ;
#7545=CARTESIAN_POINT ( 'NONE',  ( 3.435942420224999072, -12.40730057411998821, -302.9207377450070453 ) ) ;
#7548=CARTESIAN_POINT ( 'NONE',  ( 16.09890757810000750, -5.925814185855000638, -317.4928077629770087 ) ) ;
#7552=CARTESIAN_POINT ( 'NONE',  ( 19.86714287764001696, 1.744094218545000352, -303.6197174156520759 ) ) ;
#7555=CARTESIAN_POINT ( 'NONE',  ( -17.14610219660000112, -0.04370646908745000336, -314.8616023057000461 ) ) ;
#7556=CARTESIAN_POINT ( 'NONE',  ( -18.99984306468000028, 0.5551939808346000316, -302.5000000001010108 ) ) ;
#7557=ORIENTED_EDGE ( 'NONE', *, *, #5245, .T. ) ;
#7558=CARTESIAN_POINT ( 'NONE',  ( -19.86706274963002983, -1.898735342979001484, 190.4207385301700128 ) ) ;
#7559=CARTESIAN_POINT ( 'NONE',  ( -8.037373804805000077, -9.179324345868998591, -315.0000000000001137 ) ) ;
#7561=CARTESIAN_POINT ( 'NONE',  ( 18.27235334878999851, 5.234940180598000481, 190.4207385301700128 ) ) ;
#7564=CARTESIAN_POINT ( 'NONE',  ( 16.60805916514000202, -2.908391789136000050, 314.6383426456000052 ) ) ;
#7566=CARTESIAN_POINT ( 'NONE',  ( -3.163121738623003054, -11.93735872977999968, 320.0770942683900557 ) ) ;
#7568=CARTESIAN_POINT ( 'NONE',  ( -15.96459840556375376, 7.551217265629138531, -303.5000000000000000 ) ) ;
#7569=CARTESIAN_POINT ( 'NONE',  ( 13.44085293541000148, 6.266915263066000108, 314.6383426456000052 ) ) ;
#7570=EDGE_LOOP ( 'NONE', ( #5283, #4230, #67, #7504 ) ) ;
#7572=CARTESIAN_POINT ( 'NONE',  ( 16.37943014210002346, 7.176468652514003566, 318.8802828394900644 ) ) ;
#7574=CARTESIAN_POINT ( 'NONE',  ( -8.616673968646825443, 8.177724119443702477, 315.0000000000000000 ) ) ;
#7580=CARTESIAN_POINT ( 'NONE',  ( 4.353497780899999725, 11.20674699699000065, 190.0000000000000000 ) ) ;
#7581=CARTESIAN_POINT ( 'NONE',  ( -16.24410010525431503, 2.791089382272745834, -315.0000000000000000 ) ) ;
#7584=CARTESIAN_POINT ( 'NONE',  ( -12.57201637590000942, 8.467554047266999007, 190.0071920248299477 ) ) ;
#7590=CARTESIAN_POINT ( 'NONE',  ( -4.298300662841374020, -9.188610398197571527, -315.0000000000000568 ) ) ;
#7599=CARTESIAN_POINT ( 'NONE',  ( 0.2281161656705998908, -11.39695712172000164, -317.4928077629770087 ) ) ;
#7602=CARTESIAN_POINT ( 'NONE',  ( -17.43193685618000188, 1.405086463480999859, -314.4150829855000211 ) ) ;
#7603=CARTESIAN_POINT ( 'NONE',  ( -19.97270637197000909, -0.5553832019671004483, -303.6197174156509391 ) ) ;
#7604=CARTESIAN_POINT ( 'NONE',  ( 2.881524480432390771E-09, -9.999999999999998224, 315.0000000000000000 ) ) ;
#7606=CARTESIAN_POINT ( 'NONE',  ( -0.6643694614234000317, -11.51357945830000062, 190.0000000000000000 ) ) ;
#7607=CARTESIAN_POINT ( 'NONE',  ( -16.15280651819000113, 6.039793344733999980, -302.5000000000000000 ) ) ;
#7609=CARTESIAN_POINT ( 'NONE',  ( 7.802724030307999215, -11.60041405728999919, 190.4207385301700128 ) ) ;
#7610=B_SPLINE_CURVE_WITH_KNOTS ( 'NONE', 1,
 ( #10509, #2240 ),
 .UNSPECIFIED., .F., .F.,
 ( 2, 2 ),
 ( 0.01907785912498438652, 0.8020667992272817459 ),
 .UNSPECIFIED. ) ;
#7611=CARTESIAN_POINT ( 'NONE',  ( 17.50000000000125056, 1.380497925828168986E-12, -315.0000000000001705 ) ) ;
#7612=CARTESIAN_POINT ( 'NONE',  ( 15.25170542629001602, -6.686182281419003282, -302.5071922382879279 ) ) ;
#7613=CARTESIAN_POINT ( 'NONE',  ( -13.14174346518001535, 9.520659322650999457, 190.4207385301700128 ) ) ;
#7616=CARTESIAN_POINT ( 'NONE',  ( 10.67587555525000020, -8.049811041411000900, 314.4150829855000211 ) ) ;
#7619=CARTESIAN_POINT ( 'NONE',  ( 18.69275906597000869, -1.650694058049998469, 319.9928079742500131 ) ) ;
#7620=CARTESIAN_POINT ( 'NONE',  ( -7.551446853019275984, 9.031194155076960328, 314.4999434017205431 ) ) ;
#7621=CARTESIAN_POINT ( 'NONE',  ( -12.85811403544582454, 9.588400772462147614, -303.5000000000000000 ) ) ;
#7622=CARTESIAN_POINT ( 'NONE',  ( 17.35477687787999912, -0.3068793820639000303, 314.6383426456000052 ) ) ;
#7624=CARTESIAN_POINT ( 'NONE',  ( 14.83495203015046648, -8.394818437327874250, 190.9999999999995737 ) ) ;
#7625=CARTESIAN_POINT ( 'NONE',  ( 17.71262672283002360, 5.941112223585997221, 319.5792614743400009 ) ) ;
#7628=CARTESIAN_POINT ( 'NONE',  ( 8.021995032228604217, 8.375907102466543463, 315.0000000000000568 ) ) ;
#7632=CARTESIAN_POINT ( 'NONE',  ( -5.145495120689000501, -11.07694361959999974, -302.5000000000000000 ) ) ;
#7637=CARTESIAN_POINT ( 'NONE',  ( -16.21588929933999523, 5.798404451932999137, 190.0071920248299477 ) ) ;
#7639=( BOUNDED_SURFACE ( )  B_SPLINE_SURFACE ( 3, 3, ( 
 ( #5399, #6873, #8521, #5343, #3691, #1165, #4444, #8677, #2182, #7723, #6106, #5451, #4545, #9442, #9393, #7820, #466, #2028, #9543, #8729, #2885, #3739, #5295, #6206, #523, #8568, #1213, #4490, #7672, #7768, #411, #4397, #7028, #10350, #2988, #6978, #10249, #7875, #10300, #314, #4601 ),
 ( #3794, #2936, #9492, #2132, #7082, #3590, #6309, #7927, #2236, #10451, #5615, #10565, #1540, #2452, #7343, #3256, #7182, #785, #1597, #8897, #3092, #734, #8783, #3901, #7990, #3851, #572, #5560, #10614, #6535, #7291, #7130, #3037, #2399, #6368, #5503, #6425, #8951, #8090, #9812, #1371 ),
 ( #4065, #6481, #4820, #4010, #3207, #9760, #5667, #1427, #4655, #4713, #9708, #4869, #10398, #4765, #8148, #8035, #9648, #628, #9595, #2290, #8845, #1487, #5720, #683, #3955, #7235, #10505, #3148, #2349, #1645, #6693, #4971, #10025, #835, #3308, #9972, #8298, #9870, #9061, #2613, #5019 ),
 ( #5875, #2670, #9167, #7552, #7499, #4920, #1808, #8246, #5939, #4118, #6586, #5074, #941, #2507, #1698, #8354, #4225, #884, #5771, #992, #9227, #4280, #196, #141, #3527, #3472, #1859, #2718, #7396, #6754, #4170, #5128, #3416, #7445, #6805, #31, #8407, #1046, #4330, #10077, #7603 ) ),
 .UNSPECIFIED., .F., .F., .T. ) 
 B_SPLINE_SURFACE_WITH_KNOTS ( ( 4, 4 ),
 ( 4, 1, 1, 1, 1, 1, 1, 1, 1, 1, 1, 1, 1, 1, 1, 1, 1, 1, 1, 1, 1, 1, 1, 1, 1, 1, 1, 1, 1, 1, 1, 1, 1, 1, 1, 1, 1, 1, 4 ),
 ( 0.000000000000000000, 1.000000000000000000 ),
 ( -0.008481365240538999567, 0.000000000000000000, 0.03418499052141999589, 0.06705543243986999968, 0.09609225505224000541, 0.1212689627326999919, 0.1445858237144000136, 0.1683350686350000014, 0.1924153997444999764, 0.2163475385441999965, 0.2400901845063000140, 0.2638872993326000227, 0.2883641926465000394, 0.3138739111173999841, 0.3400736664824999811, 0.3669224033080000225, 0.3952263667259999780, 0.4258975072560999831, 0.4597904367344000098, 0.4962938553987999990, 0.5331571951194999937, 0.5680640359449000698, 0.5998794348263000176, 0.6292819723868000592, 0.6571102200006999627, 0.6841458463841999516, 0.7104758728877998974, 0.7357936615436999617, 0.7602320418247999756, 0.7841586104491999887, 0.8079717864086000123, 0.8319769714029000562, 0.8557114603086999338, 0.8789861807339000022, 0.9040973669459999584, 0.9330567862467999962, 0.9658526712421000582, 1.000000000000000000, 1.007721702948999987 ),
 .UNSPECIFIED. ) 
 GEOMETRIC_REPRESENTATION_ITEM ( )  RATIONAL_B_SPLINE_SURFACE ( (
 ( 1.236577362560999926, 1.236577362560999926, 1.236577362560999926, 1.236577362560999926, 1.236577362560999926, 1.236577362560999926, 1.236577362560999926, 1.236577362560999926, 1.236577362560999926, 1.236577362560999926, 1.236577362560999926, 1.236577362560999926, 1.236577362560999926, 1.236577362560999926, 1.236577362560999926, 1.236577362560999926, 1.236577362560999926, 1.236577362560999926, 1.236577362560999926, 1.236577362560999926, 1.236577362560999926, 1.236577362560999926, 1.236577362560999926, 1.236577362560999926, 1.236577362560999926, 1.236577362560999926, 1.236577362560999926, 1.236577362560999926, 1.236577362560999926, 1.236577362560999926, 1.236577362560999926, 1.236577362560999926, 1.236577362560999926, 1.236577362560999926, 1.236577362560999926, 1.236577362560999926, 1.236577362560999926, 1.236577362560999926, 1.236577362560999926, 1.236577362560999926, 1.236577362560999926),
 ( 0.9211408791463999712, 0.9211408791463999712, 0.9211408791463999712, 0.9211408791463999712, 0.9211408791463999712, 0.9211408791463999712, 0.9211408791463999712, 0.9211408791463999712, 0.9211408791463999712, 0.9211408791463999712, 0.9211408791463999712, 0.9211408791463999712, 0.9211408791463999712, 0.9211408791463999712, 0.9211408791463999712, 0.9211408791463999712, 0.9211408791463999712, 0.9211408791463999712, 0.9211408791463999712, 0.9211408791463999712, 0.9211408791463999712, 0.9211408791463999712, 0.9211408791463999712, 0.9211408791463999712, 0.9211408791463999712, 0.9211408791463999712, 0.9211408791463999712, 0.9211408791463999712, 0.9211408791463999712, 0.9211408791463999712, 0.9211408791463999712, 0.9211408791463999712, 0.9211408791463999712, 0.9211408791463999712, 0.9211408791463999712, 0.9211408791463999712, 0.9211408791463999712, 0.9211408791463999712, 0.9211408791463999712, 0.9211408791463999712, 0.9211408791463999712),
 ( 0.9211408791463999712, 0.9211408791463999712, 0.9211408791463999712, 0.9211408791463999712, 0.9211408791463999712, 0.9211408791463999712, 0.9211408791463999712, 0.9211408791463999712, 0.9211408791463999712, 0.9211408791463999712, 0.9211408791463999712, 0.9211408791463999712, 0.9211408791463999712, 0.9211408791463999712, 0.9211408791463999712, 0.9211408791463999712, 0.9211408791463999712, 0.9211408791463999712, 0.9211408791463999712, 0.9211408791463999712, 0.9211408791463999712, 0.9211408791463999712, 0.9211408791463999712, 0.9211408791463999712, 0.9211408791463999712, 0.9211408791463999712, 0.9211408791463999712, 0.9211408791463999712, 0.9211408791463999712, 0.9211408791463999712, 0.9211408791463999712, 0.9211408791463999712, 0.9211408791463999712, 0.9211408791463999712, 0.9211408791463999712, 0.9211408791463999712, 0.9211408791463999712, 0.9211408791463999712, 0.9211408791463999712, 0.9211408791463999712, 0.9211408791463999712),
 ( 1.236577362560999926, 1.236577362560999926, 1.236577362560999926, 1.236577362560999926, 1.236577362560999926, 1.236577362560999926, 1.236577362560999926, 1.236577362560999926, 1.236577362560999926, 1.236577362560999926, 1.236577362560999926, 1.236577362560999926, 1.236577362560999926, 1.236577362560999926, 1.236577362560999926, 1.236577362560999926, 1.236577362560999926, 1.236577362560999926, 1.236577362560999926, 1.236577362560999926, 1.236577362560999926, 1.236577362560999926, 1.236577362560999926, 1.236577362560999926, 1.236577362560999926, 1.236577362560999926, 1.236577362560999926, 1.236577362560999926, 1.236577362560999926, 1.236577362560999926, 1.236577362560999926, 1.236577362560999926, 1.236577362560999926, 1.236577362560999926, 1.236577362560999926, 1.236577362560999926, 1.236577362560999926, 1.236577362560999926, 1.236577362560999926, 1.236577362560999926, 1.236577362560999926) ) ) 
 REPRESENTATION_ITEM ( '' )  SURFACE ( )  );
#7640=CARTESIAN_POINT ( 'NONE',  ( 19.00000000000000000, 0.000000000000000000, 319.9999999999899956 ) ) ;
#7646=CARTESIAN_POINT ( 'NONE',  ( 17.30539973653000629, 4.527429531397997309, 319.9928079742500131 ) ) ;
#7647=CARTESIAN_POINT ( 'NONE',  ( 10.59678593799237944, -10.61334907845371411, -316.5000000000004547 ) ) ;
#7651=CARTESIAN_POINT ( 'NONE',  ( -7.796607451809997258, 10.36222334076000529, -317.4928077629770087 ) ) ;
#7654=CARTESIAN_POINT ( 'NONE',  ( 17.80394872498997927, -5.851108818846995518, -317.0792622552969533 ) ) ;
#7655=EDGE_CURVE ( 'NONE', #4786, #6747, #10288, .T. ) ;
#7656=CARTESIAN_POINT ( 'NONE',  ( -17.36938240862999905, 0.02134527931159000205, -314.6383426456000052 ) ) ;
#7659=CARTESIAN_POINT ( 'NONE',  ( -5.453091809460914874, -9.512452523087866041, 314.4999455543127169 ) ) ;
#7662=PLANE ( 'NONE',  #3175 ) ;
#7664=CARTESIAN_POINT ( 'NONE',  ( -13.93226991011998450, -8.970845217077998868, 191.1197171614399792 ) ) ;
#7669=CARTESIAN_POINT ( 'NONE',  ( -3.136708848033998187, 12.44064353863999983, 190.4207385301700128 ) ) ;
#7672=CARTESIAN_POINT ( 'NONE',  ( -11.26120837094999594, 9.120087085473000954, -302.5071922382879279 ) ) ;
#7673=CARTESIAN_POINT ( 'NONE',  ( 20.06808111288002294, 0.4071096865243998830, 319.5792614743400009 ) ) ;
#7674=CARTESIAN_POINT ( 'NONE',  ( -10.23467948400018912, 10.00000000050611959, 189.9999999999997442 ) ) ;
#7675=CARTESIAN_POINT ( 'NONE',  ( -14.28417481768999941, 5.042936695466000430, 315.0848619657999734 ) ) ;
#7676=VERTEX_POINT ( 'NONE', #6679 ) ;
#7677=CARTESIAN_POINT ( 'NONE',  ( 18.44574565965998758, -2.441956922350000614, 190.0071920248299477 ) ) ;
#7679=CARTESIAN_POINT ( 'NONE',  ( 12.24957049234000728, 9.976523051824997879, 319.5792614743400009 ) ) ;
#7680=FACE_OUTER_BOUND ( 'NONE', #4047, .T. ) ;
#7682=CARTESIAN_POINT ( 'NONE',  ( -4.462202093987085227, 9.163742891420229242, 315.0000000000000000 ) ) ;
#7683=CARTESIAN_POINT ( 'NONE',  ( 15.00000000000325961, 7.547804830080786473E-15, -284.9999999999999432 ) ) ;
#7684=LINE ( 'NONE', #6067, #4712 ) ;
#7687=CARTESIAN_POINT ( 'NONE',  ( 7.551447009212327366, -9.031194112208083880, 314.4999434017202589 ) ) ;
#7688=CARTESIAN_POINT ( 'NONE',  ( -16.77317840633001467, 5.196478383294000025, 190.0071920248299477 ) ) ;
#7691=B_SPLINE_SURFACE_WITH_KNOTS ( 'NONE', 3, 3, ( 
 ( #7725, #10095, #7770, #5297 ),
 ( #2030, #317, #9444, #10302 ),
 ( #3642, #6002, #5346, #3693 ),
 ( #2840, #8622, #5401, #6925 ),
 ( #4548, #413, #6108, #9395 ),
 ( #9345, #8570, #3592, #7822 ),
 ( #5199, #5249, #7877, #6980 ),
 ( #10251, #469, #2887, #6156 ),
 ( #9297, #2081, #1268, #7030 ),
 ( #2938, #8472, #4399, #1928 ),
 ( #9494, #8679, #8954, #686 ),
 ( #8848, #10568, #9653, #7932 ),
 ( #7295, #737, #631, #10352 ),
 ( #3958, #3210, #6484, #2239 ),
 ( #1543, #5670, #6371, #9545 ),
 ( #1374, #4768, #2402, #3905 ),
 ( #8093, #7238, #5507, #9763 ),
 ( #9598, #2185, #1600, #4873 ),
 ( #10454, #7185, #10508, #3095 ),
 ( #8151, #2294, #7993, #3797 ),
 ( #7086, #2990, #8038, #5618 ),
 ( #1430, #5563, #10401, #4659 ),
 ( #3153, #9711, #6266, #1490 ),
 ( #6428, #5454, #8732, #575 ),
 ( #3854, #2352, #7133, #3041 ),
 ( #4716, #8787, #8900, #6312 ),
 ( #4823, #4013, #9171, #3311 ),
 ( #9119, #7398, #1811, #3259 ),
 ( #9922, #4228, #4924, #2616 ),
 ( #2455, #9013, #6538, #4068 ),
 ( #9815, #5942, #4121, #2510 ),
 ( #5827, #7555, #6646, #8200 ),
 ( #4283, #8357, #8249, #7346 ),
 ( #8302, #200, #3475, #9873 ) ),
 .UNSPECIFIED., .F., .F., .F.,
 ( 4, 1, 1, 1, 1, 1, 1, 1, 1, 1, 1, 1, 1, 1, 1, 1, 1, 1, 1, 1, 1, 1, 1, 1, 1, 1, 1, 1, 1, 1, 1, 4 ),
 ( 4, 4 ),
 ( -0.01402646298304000005, 0.000000000000000000, 0.03448275862069000164, 0.06896551724138000328, 0.1034482758621000087, 0.1379310344828000023, 0.1724137931033999926, 0.2068965517240999863, 0.2413793103448000077, 0.2758620689655000291, 0.3103448275861999672, 0.3448275862069000164, 0.3793103448276000100, 0.4137931034483000037, 0.4482758620689999973, 0.4827586206897000465, 0.5172413793103000090, 0.5517241379310000582, 0.5862068965516999963, 0.6206896551723999345, 0.6551724137930999836, 0.6896551724138000328, 0.7241379310344999709, 0.7586206896552000201, 0.7931034482758999582, 0.8275862068966000074, 0.8620689655171999144, 0.8965517241379000746, 0.9310344827586000127, 0.9655172413793000619, 1.000000000000000000, 1.015741306098000063 ),
 ( -0.1697239316932999953, 1.169834029081999960 ),
 .UNSPECIFIED. ) ;
#7694=CARTESIAN_POINT ( 'NONE',  ( 8.377603294184089222, -8.255708763986199017, 315.0000000000000000 ) ) ;
#7697=CARTESIAN_POINT ( 'NONE',  ( 4.753602499919002078, 11.02326831536999840, 319.9928079742500131 ) ) ;
#7698=CARTESIAN_POINT ( 'NONE',  ( -11.66810544104021474, -10.16551412172561442, -316.5000000000004547 ) ) ;
#7701=CARTESIAN_POINT ( 'NONE',  ( 3.239095488904002007, 11.22417384501999038, -317.4928077629770087 ) ) ;
#7702=EDGE_CURVE ( 'NONE', #1396, #4012, #284, .T. ) ;
#7703=CARTESIAN_POINT ( 'NONE',  ( 0.2332652941727002271, -12.09631257874000099, -317.5770954168139610 ) ) ;
#7704=CARTESIAN_POINT ( 'NONE',  ( -17.21448334449999962, 1.351716521078000222, -314.6383426456000052 ) ) ;
#7709=EDGE_CURVE ( 'NONE', #4512, #1864, #7488, .T. ) ;
#7712=CARTESIAN_POINT ( 'NONE',  ( -13.15646768860626636, -9.424872508248350655, 319.0000000000003979 ) ) ;
#7714=CARTESIAN_POINT ( 'NONE',  ( -17.74479464825531849, 5.801447790587961784, -316.5000000000004547 ) ) ;
#7716=CARTESIAN_POINT ( 'NONE',  ( -10.23467949917770525, -9.999999999493892844, -302.5000000000002842 ) ) ;
#7717=CARTESIAN_POINT ( 'NONE',  ( -18.90059280977999734, -0.3165218993500001909, -302.5071922382879279 ) ) ;
#7721=( BOUNDED_SURFACE ( )  B_SPLINE_SURFACE ( 3, 3, ( 
 ( #4236, #4884, #799, #1441, #8969, #6277, #9722, #4729, #3106, #2362, #2196, #5465, #1386, #4670, #10465, #7945, #5518, #3867, #9610, #10412, #3054, #6322, #8800, #8002, #643, #5628, #3919, #7196, #5576, #8910, #9663, #8858, #1500, #4782, #3968, #7249, #9188, #9242, #7462, #3382, #9130, #9023, #9829, #2685, #2520, #7619, #105, #4346, #8420, #6656 ),
 ( #7513, #1006, #1823, #3489, #9933, #2571, #155, #6709, #1766, #8319, #9986, #4986, #4933, #2467, #5839, #5088, #1873, #5036, #8210, #4294, #954, #4241, #3430, #7566, #5784, #2629, #7408, #210, #1059, #1659, #3323, #3271, #6768, #6549, #5892, #5735, #8369, #50, #848, #4132, #10042, #6603, #5953, #9884, #9076, #5144, #1714, #8262, #901, #4187 ),
 ( #10141, #2783, #9344, #4491, #9443, #412, #1319, #6207, #2133, #6055, #10301, #468, #7769, #1980, #7724, #3692, #8621, #5400, #2733, #6821, #4445, #9493, #6874, #8678, #3591, #10092, #265, #6000, #4398, #5248, #7821, #6979, #4602, #3542, #10196, #10250, #6155, #9295, #8522, #8471, #1925, #2886, #2080, #5197, #365, #3640, #6107, #1116, #7673, #2937 ),
 ( #6924, #315, #1166, #2839, #9394, #2029, #5344, #1267, #4547, #3740, #5296, #8569, #7029, #1214, #3093, #2292, #684, #4821, #2184, #5561, #7183, #8730, #7929, #8846, #3903, #7131, #5452, #1488, #1541, #8036, #6426, #6369, #2400, #4766, #8091, #1598, #2989, #3956, #7236, #7876, #573, #10506, #3151, #9761, #10452, #9709, #5668, #1372, #735, #3852 ) ),
 .UNSPECIFIED., .F., .F., .T. ) 
 B_SPLINE_SURFACE_WITH_KNOTS ( ( 4, 4 ),
 ( 4, 1, 1, 1, 1, 1, 1, 1, 1, 1, 1, 1, 1, 1, 1, 1, 1, 1, 1, 1, 1, 1, 1, 1, 1, 1, 1, 1, 1, 1, 1, 1, 1, 1, 1, 1, 1, 1, 1, 1, 1, 1, 1, 1, 1, 1, 1, 4 ),
 ( 0.000000000000000000, 1.000000000000000000 ),
 ( -0.007735220065637000292, 0.000000000000000000, 0.01939640243318000237, 0.03761844488146999510, 0.05508578791268000513, 0.07214070117811000049, 0.08907871635319999926, 0.1060760411204000053, 0.1230053663521000068, 0.1398981196264000026, 0.1572430803250000064, 0.1753705638249999921, 0.1940981471027000138, 0.2133035938373999962, 0.2331689712455000119, 0.2537734685920000066, 0.2748467046084999699, 0.2963931466709999740, 0.3191313647827999644, 0.3438702858816999886, 0.3714013923646999893, 0.4021771076120999600, 0.4362733060512000161, 0.4736682024355999832, 0.5129970981982000522, 0.5517690204782000896, 0.5879381184936999238, 0.6208232858471999238, 0.6499923806306000529, 0.6755908196375000063, 0.6986884684476999396, 0.7204440523525998952, 0.7419552906557000949, 0.7633235764464999518, 0.7839199576433999450, 0.8036968760389999744, 0.8229339175995999955, 0.8415832447269999683, 0.8594503467308000078, 0.8767353019176999940, 0.8938012255453000598, 0.9107811110342000083, 0.9277285813575999462, 0.9448366096839999617, 0.9623662406040000006, 0.9806256863350999442, 1.000000000000000000, 1.008468161259999940 ),
 .UNSPECIFIED. ) 
 GEOMETRIC_REPRESENTATION_ITEM ( )  RATIONAL_B_SPLINE_SURFACE ( (
 ( 1.236576751392000073, 1.236576751392000073, 1.236576751392000073, 1.236576751392000073, 1.236576751392000073, 1.236576751392000073, 1.236576751392000073, 1.236576751392000073, 1.236576751392000073, 1.236576751392000073, 1.236576751392000073, 1.236576751392000073, 1.236576751392000073, 1.236576751392000073, 1.236576751392000073, 1.236576751392000073, 1.236576751392000073, 1.236576751392000073, 1.236576751392000073, 1.236576751392000073, 1.236576751392000073, 1.236576751392000073, 1.236576751392000073, 1.236576751392000073, 1.236576751392000073, 1.236576751392000073, 1.236576751392000073, 1.236576751392000073, 1.236576751392000073, 1.236576751392000073, 1.236576751392000073, 1.236576751392000073, 1.236576751392000073, 1.236576751392000073, 1.236576751392000073, 1.236576751392000073, 1.236576751392000073, 1.236576751392000073, 1.236576751392000073, 1.236576751392000073, 1.236576751392000073, 1.236576751392000073, 1.236576751392000073, 1.236576751392000073, 1.236576751392000073, 1.236576751392000073, 1.236576751392000073, 1.236576751392000073, 1.236576751392000073, 1.236576751392000073),
 ( 0.9211410828692999653, 0.9211410828692999653, 0.9211410828692999653, 0.9211410828692999653, 0.9211410828692999653, 0.9211410828692999653, 0.9211410828692999653, 0.9211410828692999653, 0.9211410828692999653, 0.9211410828692999653, 0.9211410828692999653, 0.9211410828692999653, 0.9211410828692999653, 0.9211410828692999653, 0.9211410828692999653, 0.9211410828692999653, 0.9211410828692999653, 0.9211410828692999653, 0.9211410828692999653, 0.9211410828692999653, 0.9211410828692999653, 0.9211410828692999653, 0.9211410828692999653, 0.9211410828692999653, 0.9211410828692999653, 0.9211410828692999653, 0.9211410828692999653, 0.9211410828692999653, 0.9211410828692999653, 0.9211410828692999653, 0.9211410828692999653, 0.9211410828692999653, 0.9211410828692999653, 0.9211410828692999653, 0.9211410828692999653, 0.9211410828692999653, 0.9211410828692999653, 0.9211410828692999653, 0.9211410828692999653, 0.9211410828692999653, 0.9211410828692999653, 0.9211410828692999653, 0.9211410828692999653, 0.9211410828692999653, 0.9211410828692999653, 0.9211410828692999653, 0.9211410828692999653, 0.9211410828692999653, 0.9211410828692999653, 0.9211410828692999653),
 ( 0.9211410828692999653, 0.9211410828692999653, 0.9211410828692999653, 0.9211410828692999653, 0.9211410828692999653, 0.9211410828692999653, 0.9211410828692999653, 0.9211410828692999653, 0.9211410828692999653, 0.9211410828692999653, 0.9211410828692999653, 0.9211410828692999653, 0.9211410828692999653, 0.9211410828692999653, 0.9211410828692999653, 0.9211410828692999653, 0.9211410828692999653, 0.9211410828692999653, 0.9211410828692999653, 0.9211410828692999653, 0.9211410828692999653, 0.9211410828692999653, 0.9211410828692999653, 0.9211410828692999653, 0.9211410828692999653, 0.9211410828692999653, 0.9211410828692999653, 0.9211410828692999653, 0.9211410828692999653, 0.9211410828692999653, 0.9211410828692999653, 0.9211410828692999653, 0.9211410828692999653, 0.9211410828692999653, 0.9211410828692999653, 0.9211410828692999653, 0.9211410828692999653, 0.9211410828692999653, 0.9211410828692999653, 0.9211410828692999653, 0.9211410828692999653, 0.9211410828692999653, 0.9211410828692999653, 0.9211410828692999653, 0.9211410828692999653, 0.9211410828692999653, 0.9211410828692999653, 0.9211410828692999653, 0.9211410828692999653, 0.9211410828692999653),
 ( 1.236576751392000073, 1.236576751392000073, 1.236576751392000073, 1.236576751392000073, 1.236576751392000073, 1.236576751392000073, 1.236576751392000073, 1.236576751392000073, 1.236576751392000073, 1.236576751392000073, 1.236576751392000073, 1.236576751392000073, 1.236576751392000073, 1.236576751392000073, 1.236576751392000073, 1.236576751392000073, 1.236576751392000073, 1.236576751392000073, 1.236576751392000073, 1.236576751392000073, 1.236576751392000073, 1.236576751392000073, 1.236576751392000073, 1.236576751392000073, 1.236576751392000073, 1.236576751392000073, 1.236576751392000073, 1.236576751392000073, 1.236576751392000073, 1.236576751392000073, 1.236576751392000073, 1.236576751392000073, 1.236576751392000073, 1.236576751392000073, 1.236576751392000073, 1.236576751392000073, 1.236576751392000073, 1.236576751392000073, 1.236576751392000073, 1.236576751392000073, 1.236576751392000073, 1.236576751392000073, 1.236576751392000073, 1.236576751392000073, 1.236576751392000073, 1.236576751392000073, 1.236576751392000073, 1.236576751392000073, 1.236576751392000073, 1.236576751392000073) ) ) 
 REPRESENTATION_ITEM ( '' )  SURFACE ( )  );
#7723=CARTESIAN_POINT ( 'NONE',  ( 14.28705177277001148, 7.417718350405998251, -302.5071922382879279 ) ) ;
#7724=CARTESIAN_POINT ( 'NONE',  ( -14.08562033053999585, -8.975362299151996126, 319.5792614743400009 ) ) ;
#7725=CARTESIAN_POINT ( 'NONE',  ( 16.90171868104999930, 0.3834349726278000192, -315.0848619657999734 ) ) ;
#7726=CARTESIAN_POINT ( 'NONE',  ( -15.10708484062000068, 4.236041382665999500, 315.0848619657999734 ) ) ;
#7728=CARTESIAN_POINT ( 'NONE',  ( 8.676965067697993916, -10.10010313590999509, 190.0071920248299477 ) ) ;
#7729=CARTESIAN_POINT ( 'NONE',  ( -19.98389199037000452, -0.4027620370101000491, 318.8802828394900644 ) ) ;
#7733=CARTESIAN_POINT ( 'NONE',  ( -15.63365740121746406, 3.715179591933191361, 315.0000000000000568 ) ) ;
#7734=CARTESIAN_POINT ( 'NONE',  ( 20.00000000000000000, 0.000000000000000000, 319.0000000000000000 ) ) ;
#7737=CARTESIAN_POINT ( 'NONE',  ( 10.23467949917769282, 9.999999999493891067, -302.4999999999996589 ) ) ;
#7739=CARTESIAN_POINT ( 'NONE',  ( -10.73820067419999980, 9.344548074503993718, 190.0071920248299477 ) ) ;
#7741=CARTESIAN_POINT ( 'NONE',  ( 19.00000000000000000, 0.000000000000000000, -317.4999999998989892 ) ) ;
#7744=CARTESIAN_POINT ( 'NONE',  ( 6.369677570987301252, -8.818560138237836910, 315.0000000000000000 ) ) ;
#7745=CARTESIAN_POINT ( 'NONE',  ( 8.587332113753999963, 8.603326289371000968, -314.6383426456000052 ) ) ;
#7747=CARTESIAN_POINT ( 'NONE',  ( 16.24851264371998738, 5.765366273007000331, 319.9928079742500131 ) ) ;
#7748=CARTESIAN_POINT ( 'NONE',  ( -6.468659092863069837, -11.84071280232868872, -316.5000000000004547 ) ) ;
#7751=FACE_OUTER_BOUND ( 'NONE', #7913, .T. ) ;
#7752=CARTESIAN_POINT ( 'NONE',  ( -13.93268562690000678, -9.073621533052005361, -317.0792622552969533 ) ) ;
#7755=CARTESIAN_POINT ( 'NONE',  ( 15.84843729815535873, 4.154783985720849948, -314.5664249374441965 ) ) ;
#7757=CARTESIAN_POINT ( 'NONE',  ( -16.27511603407000251, -5.909078865696000271, 190.0000000000000000 ) ) ;
#7758=CARTESIAN_POINT ( 'NONE',  ( -10.19008647966648695, -10.76511244458322381, 319.0000000000003979 ) ) ;
#7760=CARTESIAN_POINT ( 'NONE',  ( -2.648868200020001229, -12.40196232477001459, 191.1197171614399792 ) ) ;
#7763=CARTESIAN_POINT ( 'NONE',  ( -5.068019528653000982, -10.96907295785000080, -302.5071922382879279 ) ) ;
#7768=CARTESIAN_POINT ( 'NONE',  ( -12.33880146245001619, 8.595632119114995362, -302.5071922382879279 ) ) ;
#7769=CARTESIAN_POINT ( 'NONE',  ( -15.70899585331000559, -7.847162746392004173, 319.5792614743400009 ) ) ;
#7770=CARTESIAN_POINT ( 'NONE',  ( 17.34693632642999717, 0.4167404706239999923, -314.6383426456000052 ) ) ;
#7771=CARTESIAN_POINT ( 'NONE',  ( -4.001463906138999604, 9.408458373209999337, 314.8616023057000461 ) ) ;
#7773=CARTESIAN_POINT ( 'NONE',  ( -8.506801009283002202, -10.15345907998999486, 190.0071920248299477 ) ) ;
#7774=CARTESIAN_POINT ( 'NONE',  ( -15.55726960039999973, 7.859060843841005450, 318.8802828394900644 ) ) ;
#7779=LINE ( 'NONE', #2894, #3052 ) ;
#7780=CARTESIAN_POINT ( 'NONE',  ( 18.99997784094000153, 0.3131176371119000490, 319.9999999999899956 ) ) ;
#7781=CARTESIAN_POINT ( 'NONE',  ( -11.28781796570999951, -4.951468039558000633, 315.0000000000001705 ) ) ;
#7782=CARTESIAN_POINT ( 'NONE',  ( -13.67659370612792102, -5.618803873927792125, -315.0000000000000000 ) ) ;
#7786=CARTESIAN_POINT ( 'NONE',  ( 20.00000000000000000, 7.322330471414334241, -303.5000000000000000 ) ) ;
#7787=EDGE_CURVE ( 'NONE', #8305, #22, #9680, .T. ) ;
#7788=CARTESIAN_POINT ( 'NONE',  ( -7.042363285622345259, 8.656086706473072212, -315.0000000000000000 ) ) ;
#7789=CARTESIAN_POINT ( 'NONE',  ( 17.50000000000000000, 0.000000000000000000, -314.4999343908002629 ) ) ;
#7792=ORIENTED_EDGE ( 'NONE', *, *, #4899, .T. ) ;
#7793=CARTESIAN_POINT ( 'NONE',  ( -18.99987372849000167, -0.5562009942293000275, -317.4999999998989892 ) ) ;
#7796=CARTESIAN_POINT ( 'NONE',  ( 2.158263635479988896, -9.422507356620213770, 315.0000000000001137 ) ) ;
#7797=CARTESIAN_POINT ( 'NONE',  ( 6.322301096779000318, 8.991223814764000011, -314.8616023057000461 ) ) ;
#7804=CARTESIAN_POINT ( 'NONE',  ( 15.21494798568001627, 6.716444321683999519, -317.4928077629770087 ) ) ;
#7805=CARTESIAN_POINT ( 'NONE',  ( -3.312898553962003056, -11.91959439673999199, -317.5770954168139610 ) ) ;
#7807=CARTESIAN_POINT ( 'NONE',  ( 8.037373804805000077, -9.179324345868998591, -315.0000000000000000 ) ) ;
#7808=DIRECTION ( 'NONE',  ( 0.000000000000000000, 0.000000000000000000, 1.000000000000000000 ) ) ;
#7810=CARTESIAN_POINT ( 'NONE',  ( -13.37693598625000213, -8.145668871592000926, 190.0000000000000000 ) ) ;
#7813=CARTESIAN_POINT ( 'NONE',  ( -18.56670159326492708, 4.707099758006330958, -316.5000000000004547 ) ) ;
#7815=CARTESIAN_POINT ( 'NONE',  ( -16.91975252613927694, -1.077737682115705642, 314.9999999999999432 ) ) ;
#7816=CARTESIAN_POINT ( 'NONE',  ( 12.33880146245001619, -8.595632119114995362, -302.5071922382879279 ) ) ;
#7819=DIRECTION ( 'NONE',  ( 5.231090560719999733E-11, 3.356127988687999994E-12, 1.000000000000000000 ) ) ;
#7820=CARTESIAN_POINT ( 'NONE',  ( 7.736889024074004695, 10.37866566675000435, -302.5071922382879279 ) ) ;
#7821=CARTESIAN_POINT ( 'NONE',  ( 8.796035389134001292, -11.31703133948999707, 319.5792614743400009 ) ) ;
#7822=CARTESIAN_POINT ( 'NONE',  ( 17.18263598829999950, -2.199757124398999952, -314.4150829855000211 ) ) ;
#7823=CARTESIAN_POINT ( 'NONE',  ( -11.96281778373999849, 6.662668310474999522, 315.0848619657999734 ) ) ;
#7833=CARTESIAN_POINT ( 'NONE',  ( -13.92506561308973545, 5.424300063451886089, 315.0000000000000568 ) ) ;
#7834=CARTESIAN_POINT ( 'NONE',  ( -11.28781796570999951, -4.951468039558000633, -284.9999999999999432 ) ) ;
#7835=CARTESIAN_POINT ( 'NONE',  ( -15.63394123731325003, -3.714777356940329511, -315.0000000000000000 ) ) ;
#7839=CARTESIAN_POINT ( 'NONE',  ( -17.50000000000000000, 0.000000000000000000, -302.5000000000000000 ) ) ;
#7840=EDGE_CURVE ( 'NONE', #4467, #1953, #4775, .T. ) ;
#7841=CARTESIAN_POINT ( 'NONE',  ( -2.737251867098380309, 9.374957062059571911, -315.0000000000000000 ) ) ;
#7842=CARTESIAN_POINT ( 'NONE',  ( -1.232798796115999851, 12.07489154382001040, 189.9229057364800042 ) ) ;
#7843=CARTESIAN_POINT ( 'NONE',  ( 17.49957620161082872, 0.4465025197079524055, 314.4999504925934275 ) ) ;
#7849=CARTESIAN_POINT ( 'NONE',  ( 16.82367287970800973, -1.353209159721973309, 315.0000000000000000 ) ) ;
#7850=CARTESIAN_POINT ( 'NONE',  ( -10.49789511286000021, 7.639556387670999982, -314.8616023057000461 ) ) ;
#7854=CARTESIAN_POINT ( 'NONE',  ( 4.863072958135999713, 11.71397411138000422, 320.0770942683900557 ) ) ;
#7858=CARTESIAN_POINT ( 'NONE',  ( -19.56018822079001040, -0.5268747006259002497, -317.5770954168139610 ) ) ;
#7859=CARTESIAN_POINT ( 'NONE',  ( 9.398723296113995929, -11.12690316796998324, -317.0792622552969533 ) ) ;
#7861=CARTESIAN_POINT ( 'NONE',  ( 0.000000000000000000, 0.000000000000000000, 315.0000000000000000 ) ) ;
#7862=ORIENTED_EDGE ( 'NONE', *, *, #7181, .F. ) ;
#7864=CARTESIAN_POINT ( 'NONE',  ( 17.50000000000000711, -8.653813013134384923E-10, -302.5000000000000568 ) ) ;
#7866=CARTESIAN_POINT ( 'NONE',  ( 14.83086724907998999, -8.388894394345001615, 191.1197171614399792 ) ) ;
#7867=ORIENTED_EDGE ( 'NONE', *, *, #1113, .F. ) ;
#7869=CARTESIAN_POINT ( 'NONE',  ( -20.10115407781998442, -0.3730669878444000664, -302.9207377450070453 ) ) ;
#7875=CARTESIAN_POINT ( 'NONE',  ( -18.78105930652002087, 1.458809753444000767, -302.5071922382879279 ) ) ;
#7876=CARTESIAN_POINT ( 'NONE',  ( 16.98888588455999127, -6.600739700975996271, 318.8802828394900644 ) ) ;
#7877=CARTESIAN_POINT ( 'NONE',  ( 16.60805916514000202, -2.908391789136000050, -314.6383426456000052 ) ) ;
#7878=CARTESIAN_POINT ( 'NONE',  ( -17.18263598829999950, 2.199757124398999952, 314.4150829855000211 ) ) ;
#7880=CARTESIAN_POINT ( 'NONE',  ( -15.60370682163541467, -7.832153051853420145, 190.9999999999995737 ) ) ;
#7882=DIRECTION ( 'NONE',  ( 1.000000000000000000, 0.000000000000000000, 0.000000000000000000 ) ) ;
#7888=CARTESIAN_POINT ( 'NONE',  ( -8.096765587028130540, -8.344222180821057933, -315.0000000000000000 ) ) ;
#7890=CARTESIAN_POINT ( 'NONE',  ( 16.99996037728000076, -1.352915776343000118E-09, 314.9999801883000146 ) ) ;
#7892=CARTESIAN_POINT ( 'NONE',  ( 9.217250738626690421, 7.977707550455783725, -315.0000000000000568 ) ) ;
#7893=CARTESIAN_POINT ( 'NONE',  ( 19.56039901294001737, -0.5262506252542004104, 189.9229057364800042 ) ) ;
#7894=CARTESIAN_POINT ( 'NONE',  ( 12.89405919075535500, 6.798013128617255596, 314.4999472004062682 ) ) ;
#7896=CARTESIAN_POINT ( 'NONE',  ( 16.14934711101999909, -6.043101335943000585, -317.5000000000000000 ) ) ;
#7900=CARTESIAN_POINT ( 'NONE',  ( 13.89435758465052828, -5.448822883216570823, 315.0000000000000568 ) ) ;
#7901=CARTESIAN_POINT ( 'NONE',  ( -8.620760283086999820, 8.357092890497000326, -314.8616023057000461 ) ) ;
#7903=CARTESIAN_POINT ( 'NONE',  ( 6.386114867952997542, 11.42839325896998481, 320.0770942683900557 ) ) ;
#7907=CARTESIAN_POINT ( 'NONE',  ( -20.06704520635998179, -0.4211730678688000440, -317.0792622552969533 ) ) ;
#7912=CARTESIAN_POINT ( 'NONE',  ( -17.38327407059815854, 1.141731131567298885, -314.5066153449287754 ) ) ;
#7913=EDGE_LOOP ( 'NONE', ( #736, #3799, #9964, #3596 ) ) ;
#7914=CARTESIAN_POINT ( 'NONE',  ( -13.46369163363000077, 8.092480683229998917, 190.0000000000000000 ) ) ;
#7919=CARTESIAN_POINT ( 'NONE',  ( -9.142607798242581296, -7.997258514545670494, 315.0000000000000000 ) ) ;
#7920=CARTESIAN_POINT ( 'NONE',  ( -17.77274276690001287, -5.888218767436999457, -302.9207377450070453 ) ) ;
#7927=CARTESIAN_POINT ( 'NONE',  ( 16.55370135034999990, 6.459991253353003948, -302.4229045757450081 ) ) ;
#7929=CARTESIAN_POINT ( 'NONE',  ( -4.927840600415999361, -12.12262669806999149, 318.8802828394900644 ) ) ;
#7932=CARTESIAN_POINT ( 'NONE',  ( 12.28828818102000042, -7.249309191407999897, -314.4150829855000211 ) ) ;
#7936=CARTESIAN_POINT ( 'NONE',  ( 7.675832365144997560, -11.11882312068000189, 189.9229057364800042 ) ) ;
#7937=CARTESIAN_POINT ( 'NONE',  ( -2.571935587102001985, 12.40832180828999398, 318.8802828394900644 ) ) ;
#7942=CARTESIAN_POINT ( 'NONE',  ( 3.971626792229000280, -9.186906450543000702, 315.0848619657999734 ) ) ;
#7945=CARTESIAN_POINT ( 'NONE',  ( -12.62060098491999938, -8.441142645117002630, 319.9928079742500131 ) ) ;
#7946=CARTESIAN_POINT ( 'NONE',  ( -15.43598538069024784, -3.955158390306821925, -314.9999999999999432 ) ) ;
#7951=CARTESIAN_POINT ( 'NONE',  ( -4.714169693051696974, 9.123832451407691835, -314.9999999999999432 ) ) ;
#7952=CARTESIAN_POINT ( 'NONE',  ( -19.85617711436999144, 1.942822351932998792, 190.4207385301700128 ) ) ;
#7953=CARTESIAN_POINT ( 'NONE',  ( 17.05557420670857383, 2.295407582498449006, 314.4999494796126669 ) ) ;
#7959=CARTESIAN_POINT ( 'NONE',  ( -17.50000000000000000, 0.7437989020623000380, -315.0000000000000000 ) ) ;
#7960=CARTESIAN_POINT ( 'NONE',  ( -6.537559671572000575, 9.400791339334000796, -314.4150829855000211 ) ) ;
#7962=CARTESIAN_POINT ( 'NONE',  ( 10.04423725781999543, 10.37030404916000315, 320.0770942683900557 ) ) ;
#7967=CARTESIAN_POINT ( 'NONE',  ( -11.79032227421999757, 10.19419839316000065, -317.0792622552969533 ) ) ;
#7968=CARTESIAN_POINT ( 'NONE',  ( -17.71107981743001503, -5.830323931021004213, -316.3802825947000201 ) ) ;
#7978=CARTESIAN_POINT ( 'NONE',  ( 19.78167965760190583, -1.922413304792618405, 319.0000000000003979 ) ) ;
#7981=CARTESIAN_POINT ( 'NONE',  ( 19.30579288353658640, 3.388955136080751274, -316.5000000000004547 ) ) ;
#7983=CARTESIAN_POINT ( 'NONE',  ( -11.80673610560780240, -6.814824988023822527, 315.0000000000000000 ) ) ;
#7984=CARTESIAN_POINT ( 'NONE',  ( -14.97282077145999679, -8.399840787735001868, -302.9207377450070453 ) ) ;
#7985=EDGE_CURVE ( 'NONE', #6759, #3758, #8782, .T. ) ;
#7987=( BOUNDED_SURFACE ( )  B_SPLINE_SURFACE ( 3, 1, ( 
 ( #10429, #1099 ),
 ( #1860, #4331 ),
 ( #299, #9575 ),
 ( #6236, #6039 ),
 ( #6291, #3069 ),
 ( #3577, #6342 ),
 ( #7604, #9523 ) ),
 .UNSPECIFIED., .F., .F., .F. ) 
 B_SPLINE_SURFACE_WITH_KNOTS ( ( 4, 3, 4 ),
 ( 2, 2 ),
 ( 0.000000000000000000, 0.5000000000000000000, 0.9933926304564668630 ),
 ( 0.000000000000000000, 1.000000000000000000 ),
 .UNSPECIFIED. ) 
 GEOMETRIC_REPRESENTATION_ITEM ( )  RATIONAL_B_SPLINE_SURFACE ( (
 ( 1.000000000000000000, 1.000000000000000000),
 ( 0.8025111867385940068, 0.8025111867385940068),
 ( 0.8025111867385940068, 0.8025111867385940068),
 ( 1.000000000000000000, 1.000000000000000000),
 ( 0.8051209498784578367, 0.8051209498784578367),
 ( 0.8025456740775663844, 0.8025456740775663844),
 ( 0.9922741725973256433, 0.9922741725973256433) ) ) 
 REPRESENTATION_ITEM ( '' )  SURFACE ( )  );
#7990=CARTESIAN_POINT ( 'NONE',  ( -6.445113046380004818, 11.41524423681998712, -302.4229045757450081 ) ) ;
#7992=EDGE_LOOP ( 'NONE', ( #7360, #133, #4990, #7385 ) ) ;
#7993=CARTESIAN_POINT ( 'NONE',  ( -6.370857846455999507, -9.209451711050000711, -314.6383426456000052 ) ) ;
#7994=CARTESIAN_POINT ( 'NONE',  ( -17.56954514911999965, -0.4333932196220999788, 314.4150829855000211 ) ) ;
#7996=CARTESIAN_POINT ( 'NONE',  ( 14.59598702685000760, -8.048254220853003460, 189.9229057364800042 ) ) ;
#7997=CARTESIAN_POINT ( 'NONE',  ( -6.404755722164566123, 11.85477825286778497, 190.9999999999996589 ) ) ;
#7999=MECHANICAL_DESIGN_GEOMETRIC_PRESENTATION_REPRESENTATION('',(#2000),#4223);
#8000=CARTESIAN_POINT ( 'NONE',  ( -17.56330558013000243, -0.6698376231023999150, 314.4150829855000211 ) ) ;
#8001=CARTESIAN_POINT ( 'NONE',  ( 1.295798468764000066, 11.49282963429000048, 320.0000000000000000 ) ) ;
#8002=CARTESIAN_POINT ( 'NONE',  ( -3.092734256763002065, -11.24153629139000188, 319.9928079742500131 ) ) ;
#8003=CARTESIAN_POINT ( 'NONE',  ( 10.00000000000000000, -2.500000000000000000, -317.5000000000000000 ) ) ;
#8005=CARTESIAN_POINT ( 'NONE',  ( 13.57573464316000056, 3.225916527208000151, 315.0000000000000000 ) ) ;
#8008=CARTESIAN_POINT ( 'NONE',  ( -13.77732760571000092, 8.580179748050001720, 189.9229057364800042 ) ) ;
#8009=CARTESIAN_POINT ( 'NONE',  ( -17.50000000000000000, 0.000000000000000000, -302.5000000000000000 ) ) ;
#8011=CARTESIAN_POINT ( 'NONE',  ( 11.78107618649762500, 6.828710352419061103, 315.0000000000000000 ) ) ;
#8013=CARTESIAN_POINT ( 'NONE',  ( 3.427628718044569922, -12.33061748745338626, -303.4999999999996589 ) ) ;
#8014=CARTESIAN_POINT ( 'NONE',  ( 15.56325459994999960, 4.731967449628999844, -314.4150829855000211 ) ) ;
#8016=CARTESIAN_POINT ( 'NONE',  ( -18.87264390915002110, -0.3453755595577998605, 319.9928079742500131 ) ) ;
#8019=CARTESIAN_POINT ( 'NONE',  ( -8.115185848843001537, 11.51636271397001465, -317.0792622552969533 ) ) ;
#8020=CARTESIAN_POINT ( 'NONE',  ( 12.86351645698000645, -9.576920946250998767, -316.3802825947000201 ) ) ;
#8022=CARTESIAN_POINT ( 'NONE',  ( -9.820740202793000861, -9.834836518498999425, 320.0000000000000000 ) ) ;
#8026=CARTESIAN_POINT ( 'NONE',  ( 2.572515036489481766, -12.41549478438273191, 319.0000000000003979 ) ) ;
#8029=CARTESIAN_POINT ( 'NONE',  ( 3.357323174585254755, 12.33819210890098894, -316.5000000000004547 ) ) ;
#8031=CARTESIAN_POINT ( 'NONE',  ( -8.717521301463110106, -8.144085127293724469, 314.9999999999999432 ) ) ;
#8032=CARTESIAN_POINT ( 'NONE',  ( 19.56988197685000230, 0.3940236285954000772, -302.4229045757450081 ) ) ;
#8035=CARTESIAN_POINT ( 'NONE',  ( 8.052748353536003378, 11.53355103076000532, -302.9207377450070453 ) ) ;
#8036=CARTESIAN_POINT ( 'NONE',  ( 7.493827757249003518, -11.59400354817999457, 318.8802828394900644 ) ) ;
#8038=CARTESIAN_POINT ( 'NONE',  ( -8.587332113753999963, -8.603326289371000968, -314.6383426456000052 ) ) ;
#8039=LINE ( 'NONE', #6486, #938 ) ;
#8041=CARTESIAN_POINT ( 'NONE',  ( 17.30294281340998452, -5.653404495199006341, 189.9229057364800042 ) ) ;
#8042=CARTESIAN_POINT ( 'NONE',  ( -18.18198898035900157, 5.227591177500496400, 190.9999999999996589 ) ) ;
#8045=CARTESIAN_POINT ( 'NONE',  ( -1.266716818501000041, -9.650794245151999462, 314.8616023057000461 ) ) ;
#8054=CARTESIAN_POINT ( 'NONE',  ( 15.00000000000000000, 0.000000000000000000, -285.0000000000000000 ) ) ;
#8057=CARTESIAN_POINT ( 'NONE',  ( -19.37206517509000037, 1.821913627144001735, 189.9229057364800042 ) ) ;
#8059=ADVANCED_FACE ( 'NONE', ( #4356 ), #10179, .F. ) ;
#8060=CARTESIAN_POINT ( 'NONE',  ( 18.99999673287999968, -1.191366938436000035E-07, 191.0000000000000000 ) ) ;
#8064=CARTESIAN_POINT ( 'NONE',  ( 15.96459840556376086, -7.551217265629140307, -303.4999999999996589 ) ) ;
#8065=( BOUNDED_SURFACE ( )  B_SPLINE_SURFACE ( 3, 3, ( 
 ( #6028, #6084, #6134, #6796, #1141, #445, #4421, #10116, #7646, #5976, #7747, #9320, #3565, #9373, #8446, #9269, #1086, #391, #3720, #2756, #1900, #1954, #7697, #340, #5173, #4373, #2007, #3619, #8501, #10168, #2811, #5272, #8547, #1189, #4468, #3664, #6955, #10229, #3882, #10539, #9627, #9681, #9736, #499, #2268, #4745, #5375, #5429, #8016, #659 ),
 ( #8816, #3182, #10325, #2323, #1350, #3934, #10430, #1298, #548, #3767, #7060, #4632, #3018, #2216, #6402, #6237, #1464, #8655, #7962, #4579, #6456, #7903, #7854, #2967, #7214, #10482, #5534, #4797, #8068, #3825, #7159, #3124, #7266, #609, #9524, #5591, #2163, #6344, #3986, #5484, #8708, #7109, #8874, #1516, #10378, #712, #6292, #3070, #9577, #8763 ),
 ( #1404, #4688, #6828, #4247, #9792, #5898, #9197, #10099, #6880, #7625, #6006, #2379, #3496, #4352, #5642, #1122, #7679, #1879, #10049, #2691, #5959, #271, #217, #5150, #323, #163, #6774, #3548, #8927, #1830, #2739, #5095, #7518, #1772, #4404, #8426, #3437, #8326, #9250, #2430, #1571, #5699, #1066, #9301, #5043, #4848, #960, #8376, #1012, #1932 ),
 ( #4300, #3234, #5203, #8478, #6717, #9993, #10592, #3597, #8124, #760, #4044, #7572, #7321, #6510, #8986, #2635, #5254, #3746, #9499, #10147, #10204, #2138, #5404, #1378, #9449, #2942, #7937, #4450, #3801, #6112, #8683, #4553, #6061, #5302, #8528, #1172, #9400, #7774, #6984, #528, #371, #6215, #3859, #2086, #9351, #579, #2035, #2790, #7729, #1325 ) ),
 .UNSPECIFIED., .F., .F., .F. ) 
 B_SPLINE_SURFACE_WITH_KNOTS ( ( 4, 4 ),
 ( 4, 1, 1, 1, 1, 1, 1, 1, 1, 1, 1, 1, 1, 1, 1, 1, 1, 1, 1, 1, 1, 1, 1, 1, 1, 1, 1, 1, 1, 1, 1, 1, 1, 1, 1, 1, 1, 1, 1, 1, 1, 1, 1, 1, 1, 1, 1, 4 ),
 ( 0.000000000000000000, 1.000000000000000000 ),
 ( -0.007735220065637999493, 0.000000000000000000, 0.01939640243318000237, 0.03761844488146999510, 0.05508578791268000513, 0.07214070117811000049, 0.08907871635319999926, 0.1060760411204000053, 0.1230053663521000068, 0.1398981196264000026, 0.1572430803250000064, 0.1753705638249999921, 0.1940981471027000138, 0.2133035938373999962, 0.2331689712455000119, 0.2537734685920000066, 0.2748467046084999699, 0.2963931466709999740, 0.3191313647827999644, 0.3438702858816999886, 0.3714013923646999893, 0.4021771076120999600, 0.4362733060512000161, 0.4736682024355999832, 0.5129970981982000522, 0.5517690204782000896, 0.5879381184936999238, 0.6208232858471999238, 0.6499923806306000529, 0.6755908196375000063, 0.6986884684476999396, 0.7204440523525998952, 0.7419552906557000949, 0.7633235764464999518, 0.7839199576433999450, 0.8036968760389999744, 0.8229339175995999955, 0.8415832447269999683, 0.8594503467308000078, 0.8767353019176999940, 0.8938012255453000598, 0.9107811110342000083, 0.9277285813575999462, 0.9448366096839999617, 0.9623662406040000006, 0.9806256863350999442, 1.000000000000000000, 1.008468161259999940 ),
 .UNSPECIFIED. ) 
 GEOMETRIC_REPRESENTATION_ITEM ( )  RATIONAL_B_SPLINE_SURFACE ( (
 ( 1.236576751392000073, 1.236576751392000073, 1.236576751392000073, 1.236576751392000073, 1.236576751392000073, 1.236576751392000073, 1.236576751392000073, 1.236576751392000073, 1.236576751392000073, 1.236576751392000073, 1.236576751392000073, 1.236576751392000073, 1.236576751392000073, 1.236576751392000073, 1.236576751392000073, 1.236576751392000073, 1.236576751392000073, 1.236576751392000073, 1.236576751392000073, 1.236576751392000073, 1.236576751392000073, 1.236576751392000073, 1.236576751392000073, 1.236576751392000073, 1.236576751392000073, 1.236576751392000073, 1.236576751392000073, 1.236576751392000073, 1.236576751392000073, 1.236576751392000073, 1.236576751392000073, 1.236576751392000073, 1.236576751392000073, 1.236576751392000073, 1.236576751392000073, 1.236576751392000073, 1.236576751392000073, 1.236576751392000073, 1.236576751392000073, 1.236576751392000073, 1.236576751392000073, 1.236576751392000073, 1.236576751392000073, 1.236576751392000073, 1.236576751392000073, 1.236576751392000073, 1.236576751392000073, 1.236576751392000073, 1.236576751392000073, 1.236576751392000073),
 ( 0.9211410828692999653, 0.9211410828692999653, 0.9211410828692999653, 0.9211410828692999653, 0.9211410828692999653, 0.9211410828692999653, 0.9211410828692999653, 0.9211410828692999653, 0.9211410828692999653, 0.9211410828692999653, 0.9211410828692999653, 0.9211410828692999653, 0.9211410828692999653, 0.9211410828692999653, 0.9211410828692999653, 0.9211410828692999653, 0.9211410828692999653, 0.9211410828692999653, 0.9211410828692999653, 0.9211410828692999653, 0.9211410828692999653, 0.9211410828692999653, 0.9211410828692999653, 0.9211410828692999653, 0.9211410828692999653, 0.9211410828692999653, 0.9211410828692999653, 0.9211410828692999653, 0.9211410828692999653, 0.9211410828692999653, 0.9211410828692999653, 0.9211410828692999653, 0.9211410828692999653, 0.9211410828692999653, 0.9211410828692999653, 0.9211410828692999653, 0.9211410828692999653, 0.9211410828692999653, 0.9211410828692999653, 0.9211410828692999653, 0.9211410828692999653, 0.9211410828692999653, 0.9211410828692999653, 0.9211410828692999653, 0.9211410828692999653, 0.9211410828692999653, 0.9211410828692999653, 0.9211410828692999653, 0.9211410828692999653, 0.9211410828692999653),
 ( 0.9211410828692999653, 0.9211410828692999653, 0.9211410828692999653, 0.9211410828692999653, 0.9211410828692999653, 0.9211410828692999653, 0.9211410828692999653, 0.9211410828692999653, 0.9211410828692999653, 0.9211410828692999653, 0.9211410828692999653, 0.9211410828692999653, 0.9211410828692999653, 0.9211410828692999653, 0.9211410828692999653, 0.9211410828692999653, 0.9211410828692999653, 0.9211410828692999653, 0.9211410828692999653, 0.9211410828692999653, 0.9211410828692999653, 0.9211410828692999653, 0.9211410828692999653, 0.9211410828692999653, 0.9211410828692999653, 0.9211410828692999653, 0.9211410828692999653, 0.9211410828692999653, 0.9211410828692999653, 0.9211410828692999653, 0.9211410828692999653, 0.9211410828692999653, 0.9211410828692999653, 0.9211410828692999653, 0.9211410828692999653, 0.9211410828692999653, 0.9211410828692999653, 0.9211410828692999653, 0.9211410828692999653, 0.9211410828692999653, 0.9211410828692999653, 0.9211410828692999653, 0.9211410828692999653, 0.9211410828692999653, 0.9211410828692999653, 0.9211410828692999653, 0.9211410828692999653, 0.9211410828692999653, 0.9211410828692999653, 0.9211410828692999653),
 ( 1.236576751392000073, 1.236576751392000073, 1.236576751392000073, 1.236576751392000073, 1.236576751392000073, 1.236576751392000073, 1.236576751392000073, 1.236576751392000073, 1.236576751392000073, 1.236576751392000073, 1.236576751392000073, 1.236576751392000073, 1.236576751392000073, 1.236576751392000073, 1.236576751392000073, 1.236576751392000073, 1.236576751392000073, 1.236576751392000073, 1.236576751392000073, 1.236576751392000073, 1.236576751392000073, 1.236576751392000073, 1.236576751392000073, 1.236576751392000073, 1.236576751392000073, 1.236576751392000073, 1.236576751392000073, 1.236576751392000073, 1.236576751392000073, 1.236576751392000073, 1.236576751392000073, 1.236576751392000073, 1.236576751392000073, 1.236576751392000073, 1.236576751392000073, 1.236576751392000073, 1.236576751392000073, 1.236576751392000073, 1.236576751392000073, 1.236576751392000073, 1.236576751392000073, 1.236576751392000073, 1.236576751392000073, 1.236576751392000073, 1.236576751392000073, 1.236576751392000073, 1.236576751392000073, 1.236576751392000073, 1.236576751392000073, 1.236576751392000073) ) ) 
 REPRESENTATION_ITEM ( '' )  SURFACE ( )  );
#8066=CARTESIAN_POINT ( 'NONE',  ( -16.13341719193999779, -6.058597787994999706, -302.5000000000000000 ) ) ;
#8067=CARTESIAN_POINT ( 'NONE',  ( 1.279515965483999906E-07, 10.00000000755999885, 190.0000000000000000 ) ) ;
#8068=CARTESIAN_POINT ( 'NONE',  ( -5.958765323235996725, 11.51784730653000643, 320.0770942683900557 ) ) ;
#8072=CARTESIAN_POINT ( 'NONE',  ( -10.44399617086000021, 10.22112142899999476, -317.5770954168139610 ) ) ;
#8076=CARTESIAN_POINT ( 'NONE',  ( -17.81405818021000087, -3.987619665940000502, 320.0000000000000000 ) ) ;
#8079=CARTESIAN_POINT ( 'NONE',  ( 16.68824139745838409, -1.819223930145251966, -315.0000000000000000 ) ) ;
#8081=CARTESIAN_POINT ( 'NONE',  ( 18.18176685080253563, -5.227975112149438885, 319.0000000000003979 ) ) ;
#8083=CARTESIAN_POINT ( 'NONE',  ( 10.46398288055045711, 10.66551579990979803, -316.5000000000004547 ) ) ;
#8085=CARTESIAN_POINT ( 'NONE',  ( -15.48936016237493973, -3.890032586757016908, 315.0000000000000000 ) ) ;
#8086=CARTESIAN_POINT ( 'NONE',  ( -19.46046181435998079, -1.651614223715000884, -302.4229045757450081 ) ) ;
#8088=EDGE_CURVE ( 'NONE', #1010, #4592, #6894, .T. ) ;
#8089=SURFACE_SIDE_STYLE ('',( #1536 ) ) ;
#8090=CARTESIAN_POINT ( 'NONE',  ( -19.60208457603997090, 0.3236162399036999759, -302.4229045757450081 ) ) ;
#8091=CARTESIAN_POINT ( 'NONE',  ( 12.95981497614000588, -9.523197563374992569, 318.8802828394900644 ) ) ;
#8093=CARTESIAN_POINT ( 'NONE',  ( 1.388768300183999882, -9.421618921053999784, -315.0848619657999734 ) ) ;
#8097=CARTESIAN_POINT ( 'NONE',  ( 12.90475631688000746, -9.082603241465001531, 189.9229057364800042 ) ) ;
#8098=CARTESIAN_POINT ( 'NONE',  ( 4.467179684046221233, 12.20122392890712959, 190.9999999999996589 ) ) ;
#8099=DIRECTION ( 'NONE',  ( 0.000000000000000000, -1.000000000000000000, 0.000000000000000000 ) ) ;
#8101=CARTESIAN_POINT ( 'NONE',  ( -17.34089965840999881, -0.6440164457022999889, 314.6383426456000052 ) ) ;
#8102=CARTESIAN_POINT ( 'NONE',  ( -17.80730577449000052, 3.998365122558999563, 320.0000000000000000 ) ) ;
#8105=CARTESIAN_POINT ( 'NONE',  ( 11.22905947253953762, 10.35317575229729137, 319.0000000000005116 ) ) ;
#8106=CARTESIAN_POINT ( 'NONE',  ( 10.23467949614886763, -10.00000000050611781, 190.0000000000003979 ) ) ;
#8107=CARTESIAN_POINT ( 'NONE',  ( 0.000000000000000000, 7.937240849781000307, 315.0000000000000000 ) ) ;
#8110=VERTEX_POINT ( 'NONE', #3808 ) ;
#8112=AXIS2_PLACEMENT_3D ( 'NONE', #7861, #6855, #2015 ) ;
#8115=CARTESIAN_POINT ( 'NONE',  ( -17.33327037445098284, -2.718756893828222469E-08, -314.6666037066913191 ) ) ;
#8117=CARTESIAN_POINT ( 'NONE',  ( -18.54125634398931766, -4.746072667744948070, -303.4999999999996589 ) ) ;
#8118=CARTESIAN_POINT ( 'NONE',  ( 17.14610219660000112, 0.04370646908745000336, -314.8616023057000461 ) ) ;
#8119=ADVANCED_FACE ( 'NONE', ( #1226 ), #10247, .T. ) ;
#8120=B_SPLINE_CURVE_WITH_KNOTS ( 'NONE', 3,
 ( #7124, #4812, #5928, #3298, #5122, #23, #3248, #8348, #9862, #829, #1742, #4273, #3410, #9219, #7335, #8239, #190, #4964, #7440, #6579, #4915, #7493, #1797, #9159, #4108, #10606, #8192, #5012, #5067, #6526, #79, #986, #3359, #9054, #2500, #1852, #6685, #876, #5766 ),
 .UNSPECIFIED., .F., .F.,
 ( 4, 1, 1, 1, 1, 1, 1, 1, 1, 1, 1, 1, 1, 1, 1, 1, 1, 1, 1, 1, 1, 1, 1, 1, 1, 1, 1, 1, 1, 1, 1, 1, 1, 1, 1, 1, 4 ),
 ( 0.000000000000000000, 0.02777777777778000015, 0.05555555555556000030, 0.08333333333333001192, 0.1111111111111000027, 0.1388888888888999973, 0.1666666666667000196, 0.1944444444444000109, 0.2222222222222000054, 0.2500000000000000000, 0.2777777777777999946, 0.3055555555555999891, 0.3333333333333000081, 0.3611111111111000027, 0.3888888888888999973, 0.4166666666666999919, 0.4444444444444000109, 0.4722222222222000054, 0.5000000000000000000, 0.5277777777777999946, 0.5555555555555999891, 0.5833333333333000637, 0.6111111111111000582, 0.6388888888888999418, 0.6666666666667000474, 0.6944444444444000109, 0.7222222222222000054, 0.7500000000000000000, 0.7777777777777999946, 0.8055555555555999891, 0.8333333333333000637, 0.8611111111111000582, 0.8888888888888999418, 0.9166666666667000474, 0.9444444444444000109, 0.9722222222222000054, 1.000000000000000000 ),
 .UNSPECIFIED. ) ;
#8124=CARTESIAN_POINT ( 'NONE',  ( 18.20466326549998470, 5.184475519960003886, 318.8802828394900644 ) ) ;
#8125=LINE ( 'NONE', #761, #7405 ) ;
#8127=VERTEX_POINT ( 'NONE', #2040 ) ;
#8128=CARTESIAN_POINT ( 'NONE',  ( 10.46141074968000062, 10.65879569097000079, -316.3802825947000201 ) ) ;
#8129=CARTESIAN_POINT ( 'NONE',  ( 14.96823785528000528, -8.299997444912003530, -316.3802825947000201 ) ) ;
#8137=CARTESIAN_POINT ( 'NONE',  ( -4.928966968695707607, -12.12973353869087845, 319.0000000000003979 ) ) ;
#8142=CARTESIAN_POINT ( 'NONE',  ( 19.98289592923002544, 0.4160572288964003440, -303.6197174156509391 ) ) ;
#8143=CLOSED_SHELL ( 'NONE', ( #6068, #7470, #197, #5023, #8119, #8256, #10022, #6485, #2533, #627, #1148, #5679, #3900, #1080, #9649, #2128, #5325, #5612, #8584, #361, #8896, #6750, #8059, #1470, #5152, #4036 ) ) ;
#8148=CARTESIAN_POINT ( 'NONE',  ( 9.338997116452000924, 11.14661793222000519, -302.9207377450070453 ) ) ;
#8149=CARTESIAN_POINT ( 'NONE',  ( 19.99999035944999903, -7.277437094418000096E-10, -303.5000000000000000 ) ) ;
#8151=CARTESIAN_POINT ( 'NONE',  ( -6.273744347102000241, -8.772995918477999311, -315.0848619657999734 ) ) ;
#8152=CARTESIAN_POINT ( 'NONE',  ( -17.12432750374000179, -0.4000877216259000058, 314.8616023057000461 ) ) ;
#8154=CARTESIAN_POINT ( 'NONE',  ( -14.16528011596000169, -7.496216825914998161, 190.0071920248299477 ) ) ;
#8155=CARTESIAN_POINT ( 'NONE',  ( 6.109815047729934001, 11.91693857169685167, 190.9999999999996589 ) ) ;
#8156=CARTESIAN_POINT ( 'NONE',  ( 7.529234060647197246, 8.513083068079142279, -315.0000000000000000 ) ) ;
#8159=CARTESIAN_POINT ( 'NONE',  ( -1.276003512426000075, -9.874146089817999794, 314.6383426456000052 ) ) ;
#8163=CARTESIAN_POINT ( 'NONE',  ( 17.04674817168136158, 6.551802883975647696, 319.0000000000005116 ) ) ;
#8164=CARTESIAN_POINT ( 'NONE',  ( -17.50000000000000711, 8.653861160270983887E-10, -302.4999999999999432 ) ) ;
#8165=CARTESIAN_POINT ( 'NONE',  ( -7.006889269069000115, 6.844138725329000472, 315.0000000000000000 ) ) ;
#8167=CARTESIAN_POINT ( 'NONE',  ( 17.49999998541728985, 5.867334130787307700, 190.0000000000002274 ) ) ;
#8168=( GEOMETRIC_REPRESENTATION_CONTEXT ( 3 ) GLOBAL_UNCERTAINTY_ASSIGNED_CONTEXT ( ( #8830 ) ) GLOBAL_UNIT_ASSIGNED_CONTEXT ( ( #10504, #4009, #5018 ) ) REPRESENTATION_CONTEXT ( 'NONE', 'WORKASPACE' ) );
#8173=CARTESIAN_POINT ( 'NONE',  ( 16.37177374402162400, 2.538919766875962658, 314.9999999999999432 ) ) ;
#8174=CARTESIAN_POINT ( 'NONE',  ( -8.037373804805000077, 9.179324345868998591, -315.0000000000000000 ) ) ;
#8181=CARTESIAN_POINT ( 'NONE',  ( -0.2369326581469002602, 12.59441454048000608, -317.0792622552969533 ) ) ;
#8184=CARTESIAN_POINT ( 'NONE',  ( -6.294482982547999761, -10.85527983184999989, 320.0000000000000000 ) ) ;
#8188=CARTESIAN_POINT ( 'NONE',  ( 15.24002748250033967, -4.193218933356376965, -315.0000000000001137 ) ) ;
#8190=CARTESIAN_POINT ( 'NONE',  ( 17.38327407059815854, -1.141731131567285340, -314.5066153449286048 ) ) ;
#8192=CARTESIAN_POINT ( 'NONE',  ( 10.11497662670000075, 9.727801543432001097, -317.5000000000000000 ) ) ;
#8194=CARTESIAN_POINT ( 'NONE',  ( -11.70175841024000185, -10.14170047206000014, -303.6197174156509391 ) ) ;
#8196=CARTESIAN_POINT ( 'NONE',  ( -7.006889269069000115, -6.844138725329000472, 315.0000000000000000 ) ) ;
#8198=CARTESIAN_POINT ( 'NONE',  ( 1.279516016521960085E-07, 10.00000000000000000, 314.4997059534069308 ) ) ;
#8200=CARTESIAN_POINT ( 'NONE',  ( -17.59334121105999671, -0.04733121045982999903, -314.4150829855000211 ) ) ;
#8203=CARTESIAN_POINT ( 'NONE',  ( 20.04238130943000940, -0.9501178419093005978, 190.4207385301700128 ) ) ;
#8205=CARTESIAN_POINT ( 'NONE',  ( -12.16184652991773163, 9.933083713569276441, 190.9999999999996589 ) ) ;
#8206=CARTESIAN_POINT ( 'NONE',  ( 16.99910511164432947, 0.8673928700097557343, -314.9999999999999432 ) ) ;
#8208=CARTESIAN_POINT ( 'NONE',  ( 6.438474686349000997, -8.964777275824999947, 314.8616023057000461 ) ) ;
#8210=CARTESIAN_POINT ( 'NONE',  ( -10.04423725781999543, -10.37030404916000315, 320.0770942683900557 ) ) ;
#8212=CARTESIAN_POINT ( 'NONE',  ( -18.56827417761491716, 4.704550062028093116, -303.5000000000000000 ) ) ;
#8213=CARTESIAN_POINT ( 'NONE',  ( 13.18712987686000027, 5.898505050745000311, 315.0848619657999734 ) ) ;
#8215=CARTESIAN_POINT ( 'NONE',  ( -20.00000000435073133, 7.322330466772325686, -316.5000000000000000 ) ) ;
#8218=CARTESIAN_POINT ( 'NONE',  ( 14.00164231856462926, 5.362560482542400919, 315.0000000000000000 ) ) ;
#8221=CIRCLE ( 'NONE', #4451, 1.000000000000021982 ) ;
#8228=CARTESIAN_POINT ( 'NONE',  ( -13.93264803488000858, 8.974986968055002734, -316.3802825947000201 ) ) ;
#8231=CARTESIAN_POINT ( 'NONE',  ( 16.26474538691000049, -5.919460245093000061, 320.0000000000000000 ) ) ;
#8234=CARTESIAN_POINT ( 'NONE',  ( 14.02804746531204394, -5.341076607092832162, -315.0000000000000000 ) ) ;
#8237=CARTESIAN_POINT ( 'NONE',  ( 17.04726327197864322, -2.225800558269675378, -314.5277276635413841 ) ) ;
#8239=CARTESIAN_POINT ( 'NONE',  ( -6.537962633339999385, 10.80030782989000038, -317.5000000000000000 ) ) ;
#8241=CARTESIAN_POINT ( 'NONE',  ( -19.98381222165001248, 0.4032365313531999784, -303.6197174156509391 ) ) ;
#8243=CARTESIAN_POINT ( 'NONE',  ( 18.87178158963000030, 0.3573130366704001526, -317.4928077629770087 ) ) ;
#8244=CARTESIAN_POINT ( 'NONE',  ( 0.000000000000000000, -7.937240849781000307, 315.0000000000000000 ) ) ;
#8246=CARTESIAN_POINT ( 'NONE',  ( 16.84215363705000712, 6.757103037815999969, -303.6197174156509391 ) ) ;
#8249=CARTESIAN_POINT ( 'NONE',  ( -17.35477687787999912, 0.3068793820639000303, -314.6383426456000052 ) ) ;
#8253=CARTESIAN_POINT ( 'NONE',  ( 20.00511239988002998, -0.1020359997562000631, 191.1197171614399792 ) ) ;
#8256=ADVANCED_FACE ( 'NONE', ( #587 ), #7721, .T. ) ;
#8258=CARTESIAN_POINT ( 'NONE',  ( -11.16929996816999804, 10.37059603288001419, 191.1197171614399792 ) ) ;
#8260=CARTESIAN_POINT ( 'NONE',  ( 12.28828818102000042, -7.249309191407999897, 314.4150829855000211 ) ) ;
#8262=CARTESIAN_POINT ( 'NONE',  ( 19.59086175841999378, -0.09594170647769000027, 320.0770942683900557 ) ) ;
#8264=CARTESIAN_POINT ( 'NONE',  ( -13.93992802816217136, 8.979094264391768832, -303.4999999999990905 ) ) ;
#8265=CARTESIAN_POINT ( 'NONE',  ( 8.587332113753999963, 8.603326289371000968, 314.6383426456000052 ) ) ;
#8269=EDGE_CURVE ( 'NONE', #8127, #10485, #5616, .T. ) ;
#8272=CARTESIAN_POINT ( 'NONE',  ( -8.377603294184089222, 8.255708763986199017, 315.0000000000000000 ) ) ;
#8276=CARTESIAN_POINT ( 'NONE',  ( 3.370560865743999823, -11.33032003377000052, -302.5000000000000000 ) ) ;
#8282=CARTESIAN_POINT ( 'NONE',  ( 4.976995723842001951, 12.11314212604000318, -316.3802825947000201 ) ) ;
#8283=CARTESIAN_POINT ( 'NONE',  ( 18.95675155274000190, -0.9190877154199000865, 320.0000000000000000 ) ) ;
#8286=CARTESIAN_POINT ( 'NONE',  ( 13.97602275805729555, -5.383336353019481990, -315.0000000000001137 ) ) ;
#8288=CARTESIAN_POINT ( 'NONE',  ( 0.000000000000000000, 10.54711710274999881, -315.0000000000001137 ) ) ;
#8292=CARTESIAN_POINT ( 'NONE',  ( -12.81291305286001858, -9.603378439332990624, -303.6197174156509391 ) ) ;
#8294=CARTESIAN_POINT ( 'NONE',  ( -6.235150775465998052, -10.74512744517000407, -317.4928077629770087 ) ) ;
#8296=FILL_AREA_STYLE_COLOUR ( '', #6633 ) ;
#8298=CARTESIAN_POINT ( 'NONE',  ( -19.39478698591998551, 3.379789856048000196, -302.9207377450070453 ) ) ;
#8301=VERTEX_POINT ( 'NONE', #10566 ) ;
#8302=CARTESIAN_POINT ( 'NONE',  ( -16.90189876424999937, 0.3838616842170000099, -315.0848619657999734 ) ) ;
#8305=VERTEX_POINT ( 'NONE', #3796 ) ;
#8306=CARTESIAN_POINT ( 'NONE',  ( 19.95847042008000827, -0.9399586737018998939, 191.1197171614399792 ) ) ;
#8308=CARTESIAN_POINT ( 'NONE',  ( 11.33749276371198889, 7.060967193034009881, -315.0000000000000000 ) ) ;
#8311=CARTESIAN_POINT ( 'NONE',  ( -3.128426543399003279, 12.35671765842998582, 191.1197171614399792 ) ) ;
#8315=CARTESIAN_POINT ( 'NONE',  ( 17.12243801299000268, -0.5826713957640000663, 314.8616023057000461 ) ) ;
#8319=CARTESIAN_POINT ( 'NONE',  ( -17.33400069613001193, -5.617198899843996784, 320.0770942683900557 ) ) ;
#8321=CARTESIAN_POINT ( 'NONE',  ( 19.99984324442397110, 0.5882482212486084272, -303.5000000000000000 ) ) ;
#8322=CARTESIAN_POINT ( 'NONE',  ( 17.56970546055000071, -0.4338786413876999926, 314.4150829855000211 ) ) ;
#8324=CARTESIAN_POINT ( 'NONE',  ( -12.04241988217490622, -9.990194130379512316, 190.9999999999995737 ) ) ;
#8326=CARTESIAN_POINT ( 'NONE',  ( -15.60880606785999980, 7.925821651060998008, 319.5792614743400009 ) ) ;
#8329=CARTESIAN_POINT ( 'NONE',  ( -10.90962076852776796, 7.272180451173178461, 315.0000000000000000 ) ) ;
#8331=VERTEX_POINT ( 'NONE', #2237 ) ;
#8338=CARTESIAN_POINT ( 'NONE',  ( 20.06802617119998899, -0.4069525832282999134, -317.0792622552969533 ) ) ;
#8342=CARTESIAN_POINT ( 'NONE',  ( 10.00000000000000000, -2.500000000000000000, -315.0000000000000000 ) ) ;
#8343=CARTESIAN_POINT ( 'NONE',  ( 4.252979419060003430, -9.197563690522738256, -315.0000000000000568 ) ) ;
#8345=CARTESIAN_POINT ( 'NONE',  ( 0.9068124364724619024, -10.00021929074745231, -314.4998859403474967 ) ) ;
#8348=CARTESIAN_POINT ( 'NONE',  ( -15.28484891664999878, 6.814525346632999359, -317.5000000000000000 ) ) ;
#8349=ORIENTED_EDGE ( 'NONE', *, *, #9425, .T. ) ;
#8350=CARTESIAN_POINT ( 'NONE',  ( -19.97256092624000701, 0.5562539513971997973, -303.6197174156509391 ) ) ;
#8351=CARTESIAN_POINT ( 'NONE',  ( 11.58474654271000048, -9.740515853135002899, -317.5770954168139610 ) ) ;
#8352=CARTESIAN_POINT ( 'NONE',  ( -16.89986669904000394, 0.5583209492923999484, -315.0848619657999734 ) ) ;
#8354=CARTESIAN_POINT ( 'NONE',  ( 8.030503796230000546, 11.45221762926000153, -303.6197174156509391 ) ) ;
#8356=ORIENTED_EDGE ( 'NONE', *, *, #2143, .F. ) ;
#8357=CARTESIAN_POINT ( 'NONE',  ( -17.13182678275000370, 0.2945984483948000388, -314.8616023057000461 ) ) ;
#8358=CARTESIAN_POINT ( 'NONE',  ( -1.646600138488000020, 11.47371312023999934, -302.5000000000000000 ) ) ;
#8360=CARTESIAN_POINT ( 'NONE',  ( 1.252197968601000744, -12.57265714642999477, 190.4207385301700128 ) ) ;
#8364=CARTESIAN_POINT ( 'NONE',  ( -7.802724030307999215, 11.60041405728999919, 190.4207385301700128 ) ) ;
#8366=CARTESIAN_POINT ( 'NONE',  ( 6.388932193737000276, -8.746770244069999478, 315.0848619657999734 ) ) ;
#8369=CARTESIAN_POINT ( 'NONE',  ( 14.51666864684999680, -8.103202762918000346, 320.0770942683900557 ) ) ;
#8371=CARTESIAN_POINT ( 'NONE',  ( 5.118368704603114087E-10, 10.00000000003099210, 314.4999681336588537 ) ) ;
#8372=CARTESIAN_POINT ( 'NONE',  ( -9.254661647337840691, 11.09380704494734537, -303.4999999999990905 ) ) ;
#8373=CARTESIAN_POINT ( 'NONE',  ( 17.20518503178000103, 1.389427005613000032, 314.6383426456000052 ) ) ;
#8376=CARTESIAN_POINT ( 'NONE',  ( -20.08948270067001829, 0.1023867585008999687, 319.5792614743400009 ) ) ;
#8378=EDGE_CURVE ( 'NONE', #4540, #4067, #10615, .T. ) ;
#8380=CARTESIAN_POINT ( 'NONE',  ( -4.532266548732788003, 9.152838354191798587, 315.0000000000000568 ) ) ;
#8384=CARTESIAN_POINT ( 'NONE',  ( 12.36246450207000080, -8.718211867489999989, -302.5000000000000000 ) ) ;
#8394=CARTESIAN_POINT ( 'NONE',  ( 15.75853520210212366, -3.543431633405212722, -315.0000000000000000 ) ) ;
#8397=CARTESIAN_POINT ( 'NONE',  ( 19.99999036626000048, 4.642009117057000143E-09, -316.5000000000000000 ) ) ;
#8399=LINE ( 'NONE', #7388, #7085 ) ;
#8402=CARTESIAN_POINT ( 'NONE',  ( 17.42196264042997100, -5.530423875593995398, -317.5770954168139610 ) ) ;
#8407=CARTESIAN_POINT ( 'NONE',  ( -19.31742247159998271, 3.345204157467998929, -303.6197174156509391 ) ) ;
#8408=CARTESIAN_POINT ( 'NONE',  ( -11.05317446192489328, -7.762181880391725741, 314.4999466939158879 ) ) ;
#8410=CARTESIAN_POINT ( 'NONE',  ( 16.27944536538999998, -5.903984566639000064, 190.0000000000000000 ) ) ;
#8411=CARTESIAN_POINT ( 'NONE',  ( 3.664414252749999878, 11.29532875361999977, -302.5000000000000000 ) ) ;
#8413=CARTESIAN_POINT ( 'NONE',  ( -14.84250811591998520, -8.483799448551005540, 190.4207385301700128 ) ) ;
#8414=CARTESIAN_POINT ( 'NONE',  ( 17.19853431801041665, -2.231396706186351775, -314.4944826805095772 ) ) ;
#8415=CARTESIAN_POINT ( 'NONE',  ( 10.02545106797884955, 7.672278800222119166, -315.0000000000000000 ) ) ;
#8416=CARTESIAN_POINT ( 'NONE',  ( 14.84250811591998520, 8.483799448551005540, 190.4207385301700128 ) ) ;
#8418=CARTESIAN_POINT ( 'NONE',  ( 10.58688533405000065, -7.844683714540999553, 314.6383426456000052 ) ) ;
#8420=CARTESIAN_POINT ( 'NONE',  ( 18.87264390915002110, 0.3453755595577998605, 319.9928079742500131 ) ) ;
#8422=CARTESIAN_POINT ( 'NONE',  ( 6.687916194383508817, 11.79215677264877016, -303.4999999999990905 ) ) ;
#8423=CARTESIAN_POINT ( 'NONE',  ( 17.16710485141000220, 2.239552065056999997, 314.4150829855000211 ) ) ;
#8426=CARTESIAN_POINT ( 'NONE',  ( -13.92742316895000165, 9.072312068102004190, 319.5792614743400009 ) ) ;
#8428=CARTESIAN_POINT ( 'NONE',  ( -2.737672117484407863, 9.377292971636139285, 315.0000000000000568 ) ) ;
#8431=CARTESIAN_POINT ( 'NONE',  ( -3.664414252749999878, -11.29532875361999977, -302.5000000000000000 ) ) ;
#8433=DIRECTION ( 'NONE',  ( 1.000000000000000000, 0.000000000000000000, 0.000000000000000000 ) ) ;
#8435=CARTESIAN_POINT ( 'NONE',  ( -14.44867893690424410, 4.983401360453108886, -315.0000000000000568 ) ) ;
#8437=CARTESIAN_POINT ( 'NONE',  ( 18.70165185342001735, 1.614428960665998503, 190.0071920248299477 ) ) ;
#8446=CARTESIAN_POINT ( 'NONE',  ( 13.45825946928999706, 7.955479052880997770, 319.9928079742500131 ) ) ;
#8449=DIRECTION ( 'NONE',  ( 1.000000000000000000, 0.000000000000000000, 0.000000000000000000 ) ) ;
#8453=CARTESIAN_POINT ( 'NONE',  ( 13.71837527932998491, -8.620941849619004671, -317.5770954168139610 ) ) ;
#8455=CARTESIAN_POINT ( 'NONE',  ( -16.28527389671999970, 3.844447514156999812, -314.4150829855000211 ) ) ;
#8456=CARTESIAN_POINT ( 'NONE',  ( 16.94482484090574204, 2.428629253473844507, -314.5323066871361561 ) ) ;
#8457=CARTESIAN_POINT ( 'NONE',  ( 10.00000000000000000, -2.500000000000000000, -315.0000000000000000 ) ) ;
#8459=CARTESIAN_POINT ( 'NONE',  ( -16.84157450053000105, -5.300668178571999789, 190.0000000000000000 ) ) ;
#8460=CARTESIAN_POINT ( 'NONE',  ( -16.38421488526942582, -7.181844560322185878, 319.0000000000003979 ) ) ;
#8463=CARTESIAN_POINT ( 'NONE',  ( -17.50000000000125056, -1.338989683019597976E-14, -314.4944826805095204 ) ) ;
#8464=CARTESIAN_POINT ( 'NONE',  ( -18.27982664221999443, -2.925785484622998922, -302.5071922382879279 ) ) ;
#8465=CARTESIAN_POINT ( 'NONE',  ( 20.04745173227997768, 0.9063373766989004654, 190.4207385301700128 ) ) ;
#8471=CARTESIAN_POINT ( 'NONE',  ( 17.04863675780999088, -6.660280422001000566, 319.5792614743400009 ) ) ;
#8472=CARTESIAN_POINT ( 'NONE',  ( 14.43094748301999886, -5.211771040651000497, -314.8616023057000461 ) ) ;
#8473=CARTESIAN_POINT ( 'NONE',  ( -15.92197846796999983, 3.582977715798000062, 314.8616023057000461 ) ) ;
#8476=CARTESIAN_POINT ( 'NONE',  ( 19.78120799650142203, -1.924098540961039605, 190.9999999999995737 ) ) ;
#8478=CARTESIAN_POINT ( 'NONE',  ( 19.96334758606998605, 0.8982332345458986511, 318.8802828394900644 ) ) ;
#8481=DIRECTION ( 'NONE',  ( -1.905029615504999997E-09, 1.123812154447000012E-10, 1.000000000000000000 ) ) ;
#8482=CARTESIAN_POINT ( 'NONE',  ( 8.778709539581399213, 8.123450746681353252, 315.0000000000000000 ) ) ;
#8483=CARTESIAN_POINT ( 'NONE',  ( -11.71572875295034066, -12.49999999989693755, 190.9999999999999432 ) ) ;
#8487=FACE_OUTER_BOUND ( 'NONE', #9141, .T. ) ;
#8488=EDGE_CURVE ( 'NONE', #4386, #1953, #9573, .T. ) ;
#8491=CARTESIAN_POINT ( 'NONE',  ( -18.12330621507001638, 3.185864752952001222, 190.0071920248299477 ) ) ;
#8501=CARTESIAN_POINT ( 'NONE',  ( -5.823281502584001679, 10.83177932830000501, 319.9928079742500131 ) ) ;
#8505=CARTESIAN_POINT ( 'NONE',  ( -0.2281161656705998908, 11.39695712172000164, -317.4928077629770087 ) ) ;
#8506=CARTESIAN_POINT ( 'NONE',  ( 16.01024372474999069, -7.613620273433004293, -317.0792622552969533 ) ) ;
#8508=CARTESIAN_POINT ( 'NONE',  ( -17.34500932694999875, 0.6070218422356999932, -314.6383426456000052 ) ) ;
#8511=CARTESIAN_POINT ( 'NONE',  ( -18.95710617844000012, -0.9155000425601000913, 190.0000000000000000 ) ) ;
#8512=CARTESIAN_POINT ( 'NONE',  ( -18.71196753105320099, -4.439097376277244322, 319.0000000000003979 ) ) ;
#8519=CARTESIAN_POINT ( 'NONE',  ( 19.78498824058000594, 1.878712957033002340, 191.1197171614399792 ) ) ;
#8521=CARTESIAN_POINT ( 'NONE',  ( 18.90059280977999734, 0.3165218993500001909, -302.5071922382879279 ) ) ;
#8522=CARTESIAN_POINT ( 'NONE',  ( 16.36040776911000449, -7.306617842034003552, 319.5792614743400009 ) ) ;
#8524=CARTESIAN_POINT ( 'NONE',  ( -16.80445917461999983, 3.015803745947999825, 314.4150829855000211 ) ) ;
#8525=ORIENTED_EDGE ( 'NONE', *, *, #5731, .T. ) ;
#8526=CARTESIAN_POINT ( 'NONE',  ( 10.73820067419999980, -9.344548074503993718, 190.0071920248299477 ) ) ;
#8528=CARTESIAN_POINT ( 'NONE',  ( -12.95981497614000588, 9.523197563374992569, 318.8802828394900644 ) ) ;
#8529=ADVANCED_FACE ( 'NONE', ( #5722 ), #706, .F. ) ;
#8530=CARTESIAN_POINT ( 'NONE',  ( -16.90887668763000207, 0.2823175147257999673, 315.0848619657999734 ) ) ;
#8532=CARTESIAN_POINT ( 'NONE',  ( -16.33370887135086491, 2.613387004688928261, 315.0000000000000568 ) ) ;
#8533=CARTESIAN_POINT ( 'NONE',  ( -14.79012398733999767, -1.483731117707002278, 315.0000000000001705 ) ) ;
#8537=CARTESIAN_POINT ( 'NONE',  ( -16.40967564559107927, 2.462589562615133065, -315.0000000000000000 ) ) ;
#8540=B_SPLINE_SURFACE_WITH_KNOTS ( 'NONE', 3, 1, ( 
 ( #2647, #9902 ),
 ( #4207, #8929 ),
 ( #4150, #5754 ),
 ( #6566, #1573 ),
 ( #9041, #1676 ),
 ( #763, #6512 ),
 ( #917, #123 ),
 ( #5702, #8988 ),
 ( #3399, #6673 ),
 ( #2593, #9847 ),
 ( #7428, #6788 ),
 ( #1840, #5459 ),
 ( #10407, #10256 ) ),
 .UNSPECIFIED., .F., .F., .F.,
 ( 4, 1, 1, 1, 1, 1, 1, 1, 1, 1, 4 ),
 ( 2, 2 ),
 ( 0.01923076923076999858, 0.09935897435896999530, 0.1794871794871999993, 0.2596153846154000133, 0.3397435897436000274, 0.5000000000000000000, 0.6602564102564000281, 0.7403846153845999867, 0.8205128205128000562, 0.9006410256410000148, 0.9807692307692000844 ),
 ( 0.000000000000000000, 1.000000000000000000 ),
 .UNSPECIFIED. ) ;
#8543=CARTESIAN_POINT ( 'NONE',  ( 15.42265167804419512, -3.971230633025111700, 315.0000000000000568 ) ) ;
#8544=CARTESIAN_POINT ( 'NONE',  ( 3.932702496464000497, 9.868769537474999964, -314.4150829855000211 ) ) ;
#8547=CARTESIAN_POINT ( 'NONE',  ( -10.54985698513999637, 9.422913819601998142, 319.9928079742500131 ) ) ;
#8548=CARTESIAN_POINT ( 'NONE',  ( 8.094664229193856642, -11.44201740537352840, -316.5000000000004547 ) ) ;
#8552=CARTESIAN_POINT ( 'NONE',  ( 2.060812052271002059, -12.52766984582000021, -317.0792622552969533 ) ) ;
#8556=CARTESIAN_POINT ( 'NONE',  ( -8.548650239411999863, -10.26553531915999962, 190.0000000000000000 ) ) ;
#8558=CARTESIAN_POINT ( 'NONE',  ( -14.04520818109275382, -8.909665382566954506, 319.0000000000003979 ) ) ;
#8560=CARTESIAN_POINT ( 'NONE',  ( -0.7125182177439003395, -12.50545814267000644, 191.1197171614399792 ) ) ;
#8564=CARTESIAN_POINT ( 'NONE',  ( 4.466162596268001828, 12.19410025049000446, 191.1197171614399792 ) ) ;
#8567=EDGE_CURVE ( 'NONE', #8110, #8301, #452, .T. ) ;
#8568=CARTESIAN_POINT ( 'NONE',  ( -7.636686903722000430, 10.40663048292000070, -302.5071922382879279 ) ) ;
#8569=CARTESIAN_POINT ( 'NONE',  ( -16.37943014210002346, -7.176468652514003566, 318.8802828394900644 ) ) ;
#8570=CARTESIAN_POINT ( 'NONE',  ( 16.76545246634000108, -2.037063237379999947, -314.8616023057000461 ) ) ;
#8572=CARTESIAN_POINT ( 'NONE',  ( -1.419551022038999966, 10.09154694854999867, 314.4150829855000211 ) ) ;
#8574=CARTESIAN_POINT ( 'NONE',  ( 18.69235161570000159, -1.652152683404002342, 190.0071920248299477 ) ) ;
#8580=CARTESIAN_POINT ( 'NONE',  ( -10.25126250535807770, -10.00000007971003235, 314.9999999999999432 ) ) ;
#8581=CARTESIAN_POINT ( 'NONE',  ( -4.603216684274966219, -9.141664750100051862, -315.0000000000000568 ) ) ;
#8584=ADVANCED_FACE ( 'NONE', ( #547 ), #2719, .F. ) ;
#8586=CARTESIAN_POINT ( 'NONE',  ( -9.619051408962835836, 7.822710805390641120, -315.0000000000000568 ) ) ;
#8587=CARTESIAN_POINT ( 'NONE',  ( 15.60615175339998473, 6.374933892835006333, 190.0071920248299477 ) ) ;
#8589=CARTESIAN_POINT ( 'NONE',  ( 3.698987565691999713, -11.29118203779999874, -317.5000000000000000 ) ) ;
#8592=CARTESIAN_POINT ( 'NONE',  ( 15.43580712988967107, -3.955371400427518669, 315.0000000000000568 ) ) ;
#8593=CARTESIAN_POINT ( 'NONE',  ( 12.21495827233999876, 7.290170534263999969, -314.4150829855000211 ) ) ;
#8597=ADVANCED_FACE ( 'NONE', ( #7108 ), #7987, .F. ) ;
#8600=CARTESIAN_POINT ( 'NONE',  ( 12.29114107644999443, 8.620527874443991934, -317.4928077629770087 ) ) ;
#8601=CARTESIAN_POINT ( 'NONE',  ( -20.06802617119998899, 0.4069525832283997779, -317.0792622552969533 ) ) ;
#8605=CARTESIAN_POINT ( 'NONE',  ( 1.831806507035697473, 9.955740905498860371, -314.5031779949862880 ) ) ;
#8607=CARTESIAN_POINT ( 'NONE',  ( 4.792833739245000224, -11.13811509850999926, 190.0000000000000000 ) ) ;
#8611=CARTESIAN_POINT ( 'NONE',  ( -19.99999036626000048, -4.642009783819999925E-09, -316.5000000000000000 ) ) ;
#8614=CARTESIAN_POINT ( 'NONE',  ( 10.11757849520999031, -9.598459870364994373, -302.5071922382879279 ) ) ;
#8620=CARTESIAN_POINT ( 'NONE',  ( 17.50000000000002487, 1.995060298004523415E-08, 314.4999385900306947 ) ) ;
#8621=CARTESIAN_POINT ( 'NONE',  ( -12.24957049234000728, -9.976523051824997879, 319.5792614743400009 ) ) ;
#8622=CARTESIAN_POINT ( 'NONE',  ( 17.12243801299000268, -0.5826713957640000663, -314.8616023057000461 ) ) ;
#8623=CARTESIAN_POINT ( 'NONE',  ( 1.266716818501000041, 9.650794245151999462, 314.8616023057000461 ) ) ;
#8624=ORIENTED_EDGE ( 'NONE', *, *, #5879, .T. ) ;
#8625=CARTESIAN_POINT ( 'NONE',  ( 18.86316454545999832, 0.4769905026584997931, 190.0071920248299477 ) ) ;
#8628=B_SPLINE_CURVE_WITH_KNOTS ( 'NONE', 3,
 ( #6563, #3181, #4644, #6622, #9845, #6455, #561, #2483, #5440, #4589, #8717, #4948, #9899, #7914, #510, #3783, #1360, #9532, #2172, #3835, #227, #4362, #1130, #2645, #7479, #277, #7580, #5913, #1838, #3556, #1783, #6728, #6672, #6837, #330, #915, #2591, #3607, #10106, #2535, #10058, #1890, #6890, #4998, #2748, #6786, #6016, #5802 ),
 .UNSPECIFIED., .F., .F.,
 ( 4, 1, 1, 1, 1, 1, 1, 1, 1, 1, 1, 1, 1, 1, 1, 1, 1, 1, 1, 1, 1, 1, 1, 1, 1, 1, 1, 1, 1, 1, 1, 1, 1, 1, 1, 1, 1, 1, 1, 1, 1, 1, 1, 1, 1, 4 ),
 ( 0.000000000000000000, 0.02222222222221999915, 0.04444444444443999831, 0.06666666666666999641, 0.08888888888889000250, 0.1111111111111000027, 0.1333333333332999970, 0.1555555555555999947, 0.1777777777777999890, 0.2000000000000000111, 0.2222222222222000054, 0.2444444444443999997, 0.2666666666666999697, 0.2888888888889000195, 0.3111111111111000138, 0.3333333333333000081, 0.3555555555556000336, 0.3777777777777999724, 0.4000000000000000222, 0.4222222222221999610, 0.4444444444444000109, 0.4666666666666999808, 0.4888888888889000306, 0.5111111111110999694, 0.5333333333333000192, 0.5555555555555999891, 0.5777777777778000390, 0.5999999999999999778, 0.6222222222222000276, 0.6444444444443999664, 0.6666666666667000474, 0.6888888888888999862, 0.7111111111111000360, 0.7333333333333000859, 0.7555555555556000558, 0.7777777777777999946, 0.8000000000000000444, 0.8222222222221999832, 0.8444444444443999220, 0.8666666666667000030, 0.8888888888888999418, 0.9111111111110999916, 0.9333333333333000414, 0.9555555555556000114, 0.9777777777778000612, 1.000000000000000000 ),
 .UNSPECIFIED. ) ;
#8634=CARTESIAN_POINT ( 'NONE',  ( 0.000000000000000000, 0.000000000000000000, 0.000000000000000000 ) ) ;
#8635=CARTESIAN_POINT ( 'NONE',  ( -16.82367287970800973, 1.353209159721973309, 315.0000000000000000 ) ) ;
#8636=CARTESIAN_POINT ( 'NONE',  ( -17.50000000000000000, -3.147917160613439321E-08, 315.0000000000000000 ) ) ;
#8637=CARTESIAN_POINT ( 'NONE',  ( -12.16683899257771806, -6.621314373557687816, -315.0000000000000568 ) ) ;
#8642=CARTESIAN_POINT ( 'NONE',  ( -4.648899539349732990, 9.134382686408034857, -315.0000000000000000 ) ) ;
#8643=CARTESIAN_POINT ( 'NONE',  ( -14.19899178590998190, 7.472503199908998361, 190.0071920248299477 ) ) ;
#8652=CARTESIAN_POINT ( 'NONE',  ( 16.35728328174216273, -2.567538628164302228, 315.0000000000000568 ) ) ;
#8653=CARTESIAN_POINT ( 'NONE',  ( 6.419414596134000561, 9.427679607337001499, -314.4150829855000211 ) ) ;
#8654=CARTESIAN_POINT ( 'NONE',  ( -3.206493966914822025, -9.870881096968846080, 314.4999451744449743 ) ) ;
#8655=CARTESIAN_POINT ( 'NONE',  ( 11.06499621481999895, 9.965574156584002807, 320.0770942683900557 ) ) ;
#8660=CARTESIAN_POINT ( 'NONE',  ( -0.2332652941728000917, 12.09631257874000099, -317.5770954168139610 ) ) ;
#8661=CARTESIAN_POINT ( 'NONE',  ( -20.05669107747999291, 0.5612988332226998001, -317.0792622552969533 ) ) ;
#8664=CARTESIAN_POINT ( 'NONE',  ( 14.55942669488976549, 5.453671309400857758, -314.5801547934441942 ) ) ;
#8668=CARTESIAN_POINT ( 'NONE',  ( -17.50000000000000711, 8.653878165429867666E-10, 190.0000000000001137 ) ) ;
#8673=CARTESIAN_POINT ( 'NONE',  ( 14.73495828939998731, -7.957952820716998055, -302.4229045757450081 ) ) ;
#8677=CARTESIAN_POINT ( 'NONE',  ( 16.06615879071999231, 5.957812395457000143, -302.5071922382879279 ) ) ;
#8678=CARTESIAN_POINT ( 'NONE',  ( -3.213253768582002845, -12.43294388789000138, 319.5792614743400009 ) ) ;
#8679=CARTESIAN_POINT ( 'NONE',  ( 13.37260572687999982, -6.041714840053000302, -314.8616023057000461 ) ) ;
#8680=CARTESIAN_POINT ( 'NONE',  ( -15.60185585328000002, 4.689707898928999974, 314.4150829855000211 ) ) ;
#8682=CARTESIAN_POINT ( 'NONE',  ( 18.85089486759000010, -0.8058634873976002755, 190.0071920248299477 ) ) ;
#8683=CARTESIAN_POINT ( 'NONE',  ( -8.771473555299991176, 11.23637119458999223, 318.8802828394900644 ) ) ;
#8688=CARTESIAN_POINT ( 'NONE',  ( 14.79012398734008293, -1.483731117706880154, 315.0000000000001705 ) ) ;
#8689=CARTESIAN_POINT ( 'NONE',  ( -4.461988713456979561, -9.163769885065249809, -314.9999999999999432 ) ) ;
#8693=CARTESIAN_POINT ( 'NONE',  ( 8.636340573252622832, 8.171206817651022192, -315.0000000000000000 ) ) ;
#8694=CARTESIAN_POINT ( 'NONE',  ( 16.73002466287002576, 6.274001814427998980, 189.9229057364800042 ) ) ;
#8695=CARTESIAN_POINT ( 'NONE',  ( 16.56522183954892924, 3.263825208519234078, 314.4999489731222297 ) ) ;
#8699=CARTESIAN_POINT ( 'NONE',  ( 15.28484891664999878, -6.814525346632999359, -317.5000000000000000 ) ) ;
#8702=CARTESIAN_POINT ( 'NONE',  ( 3.970161185191127817, -9.235879793686278205, 315.0000000000000000 ) ) ;
#8703=CARTESIAN_POINT ( 'NONE',  ( 13.44085293541000148, 6.266915263066000108, -314.6383426456000052 ) ) ;
#8708=CARTESIAN_POINT ( 'NONE',  ( -17.29814430729002339, 5.659421966102000212, 320.0770942683900557 ) ) ;
#8711=CARTESIAN_POINT ( 'NONE',  ( 14.69255688194000520, 7.987735679832996816, -317.5770954168139610 ) ) ;
#8712=CARTESIAN_POINT ( 'NONE',  ( -12.61362476840000113, -9.241140244908006451, -317.5770954168139610 ) ) ;
#8715=CARTESIAN_POINT ( 'NONE',  ( -14.57677553938588844, 5.476482737502800013, -314.5817494731896318 ) ) ;
#8717=CARTESIAN_POINT ( 'NONE',  ( -15.66827725153000017, 6.479182156166999995, 190.0000000000000000 ) ) ;
#8720=VERTEX_POINT ( 'NONE', #8067 ) ;
#8721=CARTESIAN_POINT ( 'NONE',  ( 19.99984272814741715, 0.5882336804855479162, -316.5000000000004547 ) ) ;
#8723=CARTESIAN_POINT ( 'NONE',  ( -14.00164231856462926, -5.362560482542400919, 315.0000000000000000 ) ) ;
#8724=CARTESIAN_POINT ( 'NONE',  ( -13.67213454565999875, -8.648884013374997792, -302.4229045757450081 ) ) ;
#8726=( BOUNDED_SURFACE ( )  B_SPLINE_SURFACE ( 3, 1, ( 
 ( #8164, #645 ),
 ( #3166, #2198 ),
 ( #8912, #2252 ),
 ( #1557, #9776 ),
 ( #7198, #8106 ),
 ( #7307, #5467 ),
 ( #2417, #5683 ) ),
 .UNSPECIFIED., .F., .F., .T. ) 
 B_SPLINE_SURFACE_WITH_KNOTS ( ( 4, 3, 4 ),
 ( 2, 2 ),
 ( 0.006576891565977040048, 0.5000000000000000000, 0.9934231084340230389 ),
 ( 0.000000000000000000, 1.000000000000000000 ),
 .UNSPECIFIED. ) 
 GEOMETRIC_REPRESENTATION_ITEM ( )  RATIONAL_B_SPLINE_SURFACE ( (
 ( 0.9922222087809811075, 0.9922222087809811075),
 ( 0.8003084355045908538, 0.8003084355045908538),
 ( 0.8029010325775970403, 0.8029010325775970403),
 ( 1.000000000000000000, 1.000000000000000000),
 ( 0.8029010325775969292, 0.8029010325775969292),
 ( 0.8003084355045906317, 0.8003084355045906317),
 ( 0.9922222087809811075, 0.9922222087809811075) ) ) 
 REPRESENTATION_ITEM ( '' )  SURFACE ( )  );
#8729=CARTESIAN_POINT ( 'NONE',  ( 1.914578617915998704, 11.33709939001001032, -302.5071922382879279 ) ) ;
#8730=CARTESIAN_POINT ( 'NONE',  ( -6.472425350819999146, -11.83301930295000126, 318.8802828394900644 ) ) ;
#8732=CARTESIAN_POINT ( 'NONE',  ( -13.44085293541000148, -6.266915263066000108, -314.6383426456000052 ) ) ;
#8735=CARTESIAN_POINT ( 'NONE',  ( -18.14082875322000277, -3.150077164920001671, 190.0071920248299477 ) ) ;
#8741=CARTESIAN_POINT ( 'NONE',  ( -3.932702496464000497, -9.868769537474999964, 314.4150829855000211 ) ) ;
#8745=CARTESIAN_POINT ( 'NONE',  ( -8.517086849895166623, -8.210518282650744126, -314.9999999999999432 ) ) ;
#8747=ORIENTED_EDGE ( 'NONE', *, *, #2024, .T. ) ;
#8749=CARTESIAN_POINT ( 'NONE',  ( -8.673912564134326431, 8.158689640371338925, -315.0000000000000000 ) ) ;
#8751=CARTESIAN_POINT ( 'NONE',  ( -20.08953225942999765, 0.1031351683529000418, 190.4207385301700128 ) ) ;
#8752=CARTESIAN_POINT ( 'NONE',  ( 17.33327037445099705, 2.718757125457364851E-08, -314.6666037066913759 ) ) ;
#8754=CARTESIAN_POINT ( 'NONE',  ( -12.33668477992999968, -8.731648389349999206, -317.5000000000000000 ) ) ;
#8759=CARTESIAN_POINT ( 'NONE',  ( 7.529172669043764365, -8.513076715957524243, 315.0000000000000000 ) ) ;
#8761=CARTESIAN_POINT ( 'NONE',  ( -6.388932193737000276, 8.746770244069999478, -315.0848619657999734 ) ) ;
#8763=CARTESIAN_POINT ( 'NONE',  ( -19.56036991370999800, -0.5261966905397996719, 320.0770942683900557 ) ) ;
#8767=CARTESIAN_POINT ( 'NONE',  ( 10.31351018857999513, 10.27238149472999851, -317.5770954168139610 ) ) ;
#8770=CARTESIAN_POINT ( 'NONE',  ( 0.000000000000000000, -10.54711710274999881, -315.0000000000000000 ) ) ;
#8771=EDGE_CURVE ( 'NONE', #3758, #8913, #4146, .T. ) ;
#8774=CARTESIAN_POINT ( 'NONE',  ( -16.39561153668570270, -3.420321068896106986, -314.5539561507840176 ) ) ;
#8778=CARTESIAN_POINT ( 'NONE',  ( -12.45718924559404250, -6.445992642206118006, 315.0000000000000568 ) ) ;
#8779=CARTESIAN_POINT ( 'NONE',  ( -18.18877801098002323, -4.514014122889999037, -302.4229045757450081 ) ) ;
#8782=B_SPLINE_CURVE_WITH_KNOTS ( 'NONE', 3,
 ( #1778, #2530, #10053, #6723, #5047, #4254, #9255, #4199, #9140, #5798, #1884, #4944, #61 ),
 .UNSPECIFIED., .F., .F.,
 ( 4, 1, 1, 1, 1, 1, 1, 1, 1, 1, 4 ),
 ( 0.000000000000000000, 0.08333333333333001192, 0.1666666666667000196, 0.2500000000000000000, 0.3333333333333000081, 0.5000000000000000000, 0.6666666666667000474, 0.7500000000000000000, 0.8333333333333000637, 0.9166666666667000474, 1.000000000000000000 ),
 .UNSPECIFIED. ) ;
#8783=CARTESIAN_POINT ( 'NONE',  ( -3.382256884648001893, 11.91212135210998824, -302.4229045757450081 ) ) ;
#8787=CARTESIAN_POINT ( 'NONE',  ( -15.23514566747999943, -4.427644513407000382, -314.8616023057000461 ) ) ;
#8791=CARTESIAN_POINT ( 'NONE',  ( 8.887010007670999912, -10.76703833147000822, 189.9229057364800042 ) ) ;
#8792=CARTESIAN_POINT ( 'NONE',  ( -18.68747751655417133, 4.479206664350980027, 190.9999999999996589 ) ) ;
#8797=CARTESIAN_POINT ( 'NONE',  ( -13.44085293541000148, -6.266915263066000108, 314.6383426456000052 ) ) ;
#8799=CARTESIAN_POINT ( 'NONE',  ( 16.84305512206999822, 5.298470530761999697, 320.0000000000000000 ) ) ;
#8800=CARTESIAN_POINT ( 'NONE',  ( -4.753602499919002078, -11.02326831536999840, 319.9928079742500131 ) ) ;
#8801=CARTESIAN_POINT ( 'NONE',  ( 19.99996733365995283, 0.3063832366037737009, 319.0000000000005116 ) ) ;
#8806=CARTESIAN_POINT ( 'NONE',  ( 13.71790339694999439, 8.616951602761004025, 189.9229057364800042 ) ) ;
#8807=CARTESIAN_POINT ( 'NONE',  ( 17.50000000000000711, -8.653864165198663120E-10, 189.9999999999999432 ) ) ;
#8810=CARTESIAN_POINT ( 'NONE',  ( 11.93437769929943926, 6.745090416342686801, 315.0000000000000568 ) ) ;
#8815=CARTESIAN_POINT ( 'NONE',  ( 17.20518503178000103, 1.389427005613000032, -314.6383426456000052 ) ) ;
#8816=CARTESIAN_POINT ( 'NONE',  ( 19.56036306585002293, -0.5267516669946002983, 320.0770942683900557 ) ) ;
#8822=CARTESIAN_POINT ( 'NONE',  ( 16.55682536756000545, 6.456981081556999236, -317.5770954168139610 ) ) ;
#8823=ORIENTED_CLOSED_SHELL ( 'NONE', *, #83, .F. );
#8824=CARTESIAN_POINT ( 'NONE',  ( 19.98286815278001427, 0.4166756924005995955, -316.3802825947000201 ) ) ;
#8830=UNCERTAINTY_MEASURE_WITH_UNIT (LENGTH_MEASURE( 1.000000000000000082E-05 ), #10504, 'distance_accuracy_value', 'NONE');
#8832=CARTESIAN_POINT ( 'NONE',  ( -13.85286411329785849, 6.044949306166729208, -314.5816605312646175 ) ) ;
#8835=CARTESIAN_POINT ( 'NONE',  ( -7.251913689787720330, -9.130298775770061326, -314.5336966332658335 ) ) ;
#8836=ORIENTED_EDGE ( 'NONE', *, *, #7709, .T. ) ;
#8839=CARTESIAN_POINT ( 'NONE',  ( -11.78107618649762500, -6.828710352419061103, 315.0000000000000000 ) ) ;
#8840=CARTESIAN_POINT ( 'NONE',  ( 18.86312040460998674, 0.4763280864498002920, -302.5071922382879279 ) ) ;
#8845=CARTESIAN_POINT ( 'NONE',  ( 0.1642067852079997503, 12.59486910148998895, -302.9207377450070453 ) ) ;
#8846=CARTESIAN_POINT ( 'NONE',  ( -3.204766135845001696, -12.34903855201999079, 318.8802828394900644 ) ) ;
#8847=ORIENTED_EDGE ( 'NONE', *, *, #8771, .T. ) ;
#8848=CARTESIAN_POINT ( 'NONE',  ( 11.96281778373999849, -6.662668310474999522, -315.0848619657999734 ) ) ;
#8852=CARTESIAN_POINT ( 'NONE',  ( -15.60615175339998473, -6.374933892835006333, 190.0071920248299477 ) ) ;
#8853=CARTESIAN_POINT ( 'NONE',  ( 17.64879272652970599, 5.897502810282468921, 190.9999999999996589 ) ) ;
#8856=CARTESIAN_POINT ( 'NONE',  ( -16.54291557298000370, -1.991497705781999805, 315.0848619657999734 ) ) ;
#8857=CARTESIAN_POINT ( 'NONE',  ( 10.79636471171000167, 9.449795599854001082, 320.0000000000000000 ) ) ;
#8858=CARTESIAN_POINT ( 'NONE',  ( 9.539154743984001428, -9.809959732869000248, 319.9928079742500131 ) ) ;
#8859=CARTESIAN_POINT ( 'NONE',  ( -19.49702808861183101, 2.833672667318400507, 319.0000000000005116 ) ) ;
#8865=CARTESIAN_POINT ( 'NONE',  ( -17.68025656702000603, 5.978840677964003092, 190.4207385301700128 ) ) ;
#8867=B_SPLINE_CURVE_WITH_KNOTS ( 'NONE', 3,
 ( #8371, #9244, #5145, #212, #4347, #7620, #9988, #955, #106, #1007, #3543, #7463, #4295, #4242, #10094, #6822, #3490, #2734, #3383, #2630, #6658, #156 ),
 .UNSPECIFIED., .F., .F.,
 ( 4, 2, 2, 2, 2, 2, 2, 2, 2, 2, 4 ),
 ( 0.4999983561373720353, 0.5624985616202005101, 0.5937486643616147752, 0.6249987671030289293, 0.6562488698444431945, 0.6874989725858574596, 0.7499991780686858789, 0.8124993835515144092, 0.8749995890343429394, 0.9374997945171714697, 1.000000000000000000 ),
 .UNSPECIFIED. ) ;
#8869=CARTESIAN_POINT ( 'NONE',  ( 11.71572875766478639, -12.49999999885353041, -303.4999999999999432 ) ) ;
#8870=CARTESIAN_POINT ( 'NONE',  ( 15.47214269673303200, 3.911151857093433382, 315.0000000000000568 ) ) ;
#8872=CARTESIAN_POINT ( 'NONE',  ( 17.13182678275000370, -0.2945984483948000388, -314.8616023057000461 ) ) ;
#8874=CARTESIAN_POINT ( 'NONE',  ( -18.32873049326003212, 4.258249849688001909, 320.0770942683900557 ) ) ;
#8878=CARTESIAN_POINT ( 'NONE',  ( 18.87261805073000787, -0.3452380817474001162, -317.4928077629770087 ) ) ;
#8879=CARTESIAN_POINT ( 'NONE',  ( 8.092749801746995431, -11.43508185634000007, -316.3802825947000201 ) ) ;
#8882=ORIENTED_EDGE ( 'NONE', *, *, #5029, .T. ) ;
#8886=CARTESIAN_POINT ( 'NONE',  ( -8.988119689606875795, 8.550792887852695756, -314.5455502384737656 ) ) ;
#8888=CARTESIAN_POINT ( 'NONE',  ( -3.205490369836121900, -12.35619803902316782, 319.0000000000003979 ) ) ;
#8892=CARTESIAN_POINT ( 'NONE',  ( -3.023938872602656591, -9.348098599112928397, 315.0000000000000568 ) ) ;
#8893=CARTESIAN_POINT ( 'NONE',  ( 18.93783568409002172, -3.175510411809001177, -302.4229045757450081 ) ) ;
#8896=ADVANCED_FACE ( 'NONE', ( #6015, #8487 ), #3503, .T. ) ;
#8897=CARTESIAN_POINT ( 'NONE',  ( 1.957937398543000418, 12.03510449230999768, -302.4229045757450081 ) ) ;
#8900=CARTESIAN_POINT ( 'NONE',  ( -15.39920013370999996, -4.579805981517999669, -314.6383426456000052 ) ) ;
#8903=CARTESIAN_POINT ( 'NONE',  ( -12.48652197162000554, -8.514177154860004038, 190.0071920248299477 ) ) ;
#8904=CARTESIAN_POINT ( 'NONE',  ( 2.649465170252891522, 12.40913386102118388, 190.9999999999996589 ) ) ;
#8907=CARTESIAN_POINT ( 'NONE',  ( -17.59334121105999671, -0.04733121045982000008, 314.4150829855000211 ) ) ;
#8910=CARTESIAN_POINT ( 'NONE',  ( 7.221770056846003705, -10.51477558267000667, 319.9928079742500131 ) ) ;
#8911=CARTESIAN_POINT ( 'NONE',  ( 18.21047658595730212, 5.188723016677323940, 319.0000000000005116 ) ) ;
#8912=CARTESIAN_POINT ( 'NONE',  ( -10.23467949917771591, -9.999999999493891067, -302.5000000000002274 ) ) ;
#8913=VERTEX_POINT ( 'NONE', #5966 ) ;
#8916=CARTESIAN_POINT ( 'NONE',  ( -9.011282031845993856, 11.16162715973000097, 191.1197171614399792 ) ) ;
#8923=CARTESIAN_POINT ( 'NONE',  ( 14.97723399828063506, -8.302382553459793257, -303.4999999999996589 ) ) ;
#8924=CARTESIAN_POINT ( 'NONE',  ( -14.32653628403999946, -7.536184728883000616, -302.5000000000000000 ) ) ;
#8927=CARTESIAN_POINT ( 'NONE',  ( -6.055260875802999543, 12.00648505189998971, 319.5792614743400009 ) ) ;
#8929=CARTESIAN_POINT ( 'NONE',  ( 15.00000000000071587, 0.4945770392355663403, 315.0000000000001705 ) ) ;
#8931=CARTESIAN_POINT ( 'NONE',  ( 18.53690224725999514, 4.739426065905003149, -316.3802825947000201 ) ) ;
#8934=EDGE_LOOP ( 'NONE', ( #5365, #7136, #4648, #3863 ) ) ;
#8939=CARTESIAN_POINT ( 'NONE',  ( -9.847343584659236981, 8.231878686604520823, -314.5529121822860361 ) ) ;
#8941=CARTESIAN_POINT ( 'NONE',  ( 8.773569371117815763, -11.24325377545516602, 319.0000000000003979 ) ) ;
#8942=EDGE_LOOP ( 'NONE', ( #5657, #4255, #10442, #5723 ) ) ;
#8945=CARTESIAN_POINT ( 'NONE',  ( -8.666088325696231109, -8.161304309888411268, 315.0000000000000568 ) ) ;
#8946=CARTESIAN_POINT ( 'NONE',  ( 18.56223039349998771, -4.700611568415998143, -303.6197174156509391 ) ) ;
#8951=CARTESIAN_POINT ( 'NONE',  ( -19.46926817186999514, 1.611439533454998241, -302.4229045757450081 ) ) ;
#8954=CARTESIAN_POINT ( 'NONE',  ( 13.50042001888999899, -6.225262767767000049, -314.6383426456000052 ) ) ;
#8955=CARTESIAN_POINT ( 'NONE',  ( 15.26659686508999947, 6.829480052022000258, -302.5000000000000000 ) ) ;
#8958=CARTESIAN_POINT ( 'NONE',  ( 3.087789584922997932, -11.94493704178999671, 189.9229057364800042 ) ) ;
#8960=CARTESIAN_POINT ( 'NONE',  ( 3.970004819630974957, 9.235895690467337715, -315.0000000000000568 ) ) ;
#8964=B_SPLINE_CURVE_WITH_KNOTS ( 'NONE', 3,
 ( #5419, #7843, #9460, #4622, #7953, #8695, #1452, #2155, #4737, #9514, #7894, #490, #2100, #3115, #5475, #7152, #10473, #3816, #7102, #10369, #3010, #6333 ),
 .UNSPECIFIED., .F., .F.,
 ( 4, 2, 2, 2, 2, 2, 2, 2, 2, 2, 4 ),
 ( 0.000000000000000000, 0.06249979451717146278, 0.1249995890343429256, 0.1874993835515144092, 0.2499991780686858511, 0.3124989725858572931, 0.3437488698444430835, 0.3749987671030288738, 0.4062486643616146642, 0.4374985616202004546, 0.4999983561373720353 ),
 .UNSPECIFIED. ) ;
#8965=CARTESIAN_POINT ( 'NONE',  ( -1.285290206351000108, -10.09749793447999977, 314.4150829855000211 ) ) ;
#8967=CARTESIAN_POINT ( 'NONE',  ( 8.770005493155000664, 10.19600538561000036, 320.0000000000000000 ) ) ;
#8969=CARTESIAN_POINT ( 'NONE',  ( -18.70127769336001222, -1.615776359209001312, 319.9928079742500131 ) ) ;
#8970=CARTESIAN_POINT ( 'NONE',  ( -8.773569371117819315, 11.24325377545516780, 319.0000000000005116 ) ) ;
#8974=CARTESIAN_POINT ( 'NONE',  ( 14.79012398733999945, 1.483731117707000058, -285.0000000000000000 ) ) ;
#8982=CARTESIAN_POINT ( 'NONE',  ( -15.92130416703352935, -7.586839038430808202, -303.4999999999996589 ) ) ;
#8983=CARTESIAN_POINT ( 'NONE',  ( 17.42228208267999889, 1.444224815522999972, -314.4150829855000211 ) ) ;
#8986=CARTESIAN_POINT ( 'NONE',  ( 14.04143820182998503, 8.903536631273988533, 318.8802828394900644 ) ) ;
#8988=CARTESIAN_POINT ( 'NONE',  ( -7.006889269069000115, 6.844138725329000472, 315.0000000000001705 ) ) ;
#8990=CARTESIAN_POINT ( 'NONE',  ( -11.75551710966999153, 10.11738730586000123, -316.3802825947000201 ) ) ;
#8996=CARTESIAN_POINT ( 'NONE',  ( 14.21145943247442744, -5.188748475648757186, -315.0000000000000000 ) ) ;
#8997=ORIENTED_EDGE ( 'NONE', *, *, #6986, .F. ) ;
#9003=CARTESIAN_POINT ( 'NONE',  ( 13.97988708520999701, -9.045087908074000538, -302.9207377450070453 ) ) ;
#9011=CARTESIAN_POINT ( 'NONE',  ( -10.25126250535807770, -10.00000007971003058, 314.4997059534069308 ) ) ;
#9013=CARTESIAN_POINT ( 'NONE',  ( -16.98808798087999961, -1.334629195702000004, -314.8616023057000461 ) ) ;
#9016=CARTESIAN_POINT ( 'NONE',  ( -13.05089818882000507, -9.570190452814999915, 190.4207385301700128 ) ) ;
#9018=CARTESIAN_POINT ( 'NONE',  ( 15.26192592288500194, 4.160213195839838285, -315.0000000000000000 ) ) ;
#9020=CARTESIAN_POINT ( 'NONE',  ( 15.92197846796999983, -3.582977715798000062, 314.8616023057000461 ) ) ;
#9022=CARTESIAN_POINT ( 'NONE',  ( 4.804283134583999804, 11.13634285072000019, 320.0000000000000000 ) ) ;
#9023=CARTESIAN_POINT ( 'NONE',  ( 17.27957593929000879, -4.562754682971998932, 319.9928079742500131 ) ) ;
#9024=CARTESIAN_POINT ( 'NONE',  ( -0.6338995735901450379, 12.51432109910910029, 319.0000000000005116 ) ) ;
#9025=SURFACE_STYLE_USAGE ( .BOTH. , #9190 ) ;
#9030=DIRECTION ( 'NONE',  ( 3.267118270366935116E-06, 8.358028861085000358E-13, -0.9999999999946629359 ) ) ;
#9032=CARTESIAN_POINT ( 'NONE',  ( 15.75886148104574325, 3.542954957252464343, 315.0000000000000000 ) ) ;
#9034=CARTESIAN_POINT ( 'NONE',  ( 16.92248268936999978, 0.04189409840125999512, -315.0848619657999734 ) ) ;
#9035=EDGE_CURVE ( 'NONE', #9273, #3853, #9038, .T. ) ;
#9038=B_SPLINE_CURVE_WITH_KNOTS ( 'NONE', 3,
 ( #7890, #7045, #5311, #10364 ),
 .UNSPECIFIED., .F., .F.,
 ( 4, 4 ),
 ( 0.000000000000000000, 1.000000000000000000 ),
 .UNSPECIFIED. ) ;
#9041=CARTESIAN_POINT ( 'NONE',  ( 11.28781796570999951, 4.951468039558000633, -284.9999999999999432 ) ) ;
#9044=CARTESIAN_POINT ( 'NONE',  ( -18.56065892533998962, 4.703159488203003669, -316.3802825947000201 ) ) ;
#9046=CARTESIAN_POINT ( 'NONE',  ( -18.99997784094000153, -0.3131176371119000490, 319.9999999999899956 ) ) ;
#9050=CARTESIAN_POINT ( 'NONE',  ( 8.691431531408321476, -8.152829611300951740, -315.0000000000000000 ) ) ;
#9054=CARTESIAN_POINT ( 'NONE',  ( 16.89340345063000015, 5.253727359668999952, -317.4999999999989768 ) ) ;
#9056=CARTESIAN_POINT ( 'NONE',  ( 17.80660862177001746, -5.847896592537999538, -302.9207377450070453 ) ) ;
#9057=CARTESIAN_POINT ( 'NONE',  ( 6.508337484872001255, -10.68452134396000375, -317.4928077629770087 ) ) ;
#9060=( LENGTH_UNIT ( ) NAMED_UNIT ( * ) SI_UNIT ( .MILLI., .METRE. ) );
#9061=CARTESIAN_POINT ( 'NONE',  ( -20.10149561490999659, 0.3453761138107002138, -302.9207377450070453 ) ) ;
#9064=ORIENTED_EDGE ( 'NONE', *, *, #30, .T. ) ;
#9068=CARTESIAN_POINT ( 'NONE',  ( -19.21810730420998681, -3.675731523933000400, 190.4207385301700128 ) ) ;
#9070=CARTESIAN_POINT ( 'NONE',  ( 8.037373804805000077, -9.179324345868998591, -315.0000000000001137 ) ) ;
#9071=CARTESIAN_POINT ( 'NONE',  ( 15.44329739658677880, 3.946306641738668297, -314.9999999999999432 ) ) ;
#9073=CARTESIAN_POINT ( 'NONE',  ( 17.34693632642999717, 0.4167404706239999923, 314.6383426456000052 ) ) ;
#9076=CARTESIAN_POINT ( 'NONE',  ( 19.10207382662997588, -2.686351016941002534, 320.0770942683900557 ) ) ;
#9077=CARTESIAN_POINT ( 'NONE',  ( -10.97430844189483778, 10.45950866754415820, 319.0000000000005116 ) ) ;
#9078=CARTESIAN_POINT ( 'NONE',  ( 3.693615097834042960, 12.29963531854552450, -303.5000000000000000 ) ) ;
#9079=CARTESIAN_POINT ( 'NONE',  ( 17.56330558013000243, 0.6698376231023999150, 314.4150829855000211 ) ) ;
#9085=( BOUNDED_SURFACE ( )  B_SPLINE_SURFACE ( 3, 1, ( 
 ( #3709, #1230 ),
 ( #4508, #7786 ),
 ( #1337, #431 ),
 ( #4616, #6993 ),
 ( #2096, #749 ),
 ( #8215, #5740 ),
 ( #4030, #1448 ) ),
 .UNSPECIFIED., .F., .F., .T. ) 
 B_SPLINE_SURFACE_WITH_KNOTS ( ( 4, 3, 4 ),
 ( 2, 2 ),
 ( 0.000000000000000000, 0.5000000000000000000, 1.000000000000000000 ),
 ( 0.000000000000000000, 1.000000000000000000 ),
 .UNSPECIFIED. ) 
 GEOMETRIC_REPRESENTATION_ITEM ( )  RATIONAL_B_SPLINE_SURFACE ( (
 ( 1.000000000000000000, 1.000000000000000000),
 ( 0.8047378540805999458, 0.8047378540805999458),
 ( 0.8047378540805999458, 0.8047378540805999458),
 ( 1.000000000000000000, 1.000000000000000000),
 ( 0.8047378540805999458, 0.8047378540805999458),
 ( 0.8047378540805999458, 0.8047378540805999458),
 ( 1.000000000000000000, 1.000000000000000000) ) ) 
 REPRESENTATION_ITEM ( '' )  SURFACE ( )  );
#9086=CARTESIAN_POINT ( 'NONE',  ( 3.023938872602656591, 9.348098599112928397, 315.0000000000000568 ) ) ;
#9097=CARTESIAN_POINT ( 'NONE',  ( -5.321980890543003717, 12.05475797716000486, -316.3802825947000201 ) ) ;
#9103=DIRECTION ( 'NONE',  ( -5.580921738635028310E-06, 2.007400790903078554E-12, 0.9999999999844266796 ) ) ;
#9104=CARTESIAN_POINT ( 'NONE',  ( 15.60727917143683108, -3.742131089528405674, -315.0000000000000000 ) ) ;
#9105=VERTEX_POINT ( 'NONE', #2094 ) ;
#9107=CARTESIAN_POINT ( 'NONE',  ( 3.644504295958670426, -9.783030308347003157, -314.5117835914682018 ) ) ;
#9111=CARTESIAN_POINT ( 'NONE',  ( -19.86714287764001696, -1.744094218545000352, -303.6197174156509391 ) ) ;
#9112=CARTESIAN_POINT ( 'NONE',  ( -7.576881921353003868, -10.42269368856000611, -317.4928077629770087 ) ) ;
#9114=CARTESIAN_POINT ( 'NONE',  ( -10.00000000000000000, -2.500000000000000000, -317.5000000000000000 ) ) ;
#9117=CARTESIAN_POINT ( 'NONE',  ( 19.58578074103492739, -1.999241604668525937E-07, -302.5000071933976642 ) ) ;
#9119=CARTESIAN_POINT ( 'NONE',  ( -16.19514236092000203, -2.730451569713999938, -315.0848619657999734 ) ) ;
#9122=CARTESIAN_POINT ( 'NONE',  ( 17.68025656702000603, -5.978840677964003092, 190.4207385301700128 ) ) ;
#9126=CARTESIAN_POINT ( 'NONE',  ( -14.83086724907998999, 8.388894394345001615, 191.1197171614399792 ) ) ;
#9128=CARTESIAN_POINT ( 'NONE',  ( 14.28417481768999941, -5.042936695466000430, 315.0848619657999734 ) ) ;
#9130=CARTESIAN_POINT ( 'NONE',  ( 16.76867785761999485, -5.202124494729996940, 319.9928079742500131 ) ) ;
#9133=CARTESIAN_POINT ( 'NONE',  ( 1.257430124576000008, 9.427442400486999219, 315.0848619657999734 ) ) ;
#9135=CARTESIAN_POINT ( 'NONE',  ( -8.835721849737739220, -11.22420793802478123, 190.9999999999995737 ) ) ;
#9138=CARTESIAN_POINT ( 'NONE',  ( -8.647614135908284538, 8.167456227882626152, 315.0000000000000568 ) ) ;
#9140=CARTESIAN_POINT ( 'NONE',  ( 11.28781796570999951, -4.951468039558000633, -285.0000000000000000 ) ) ;
#9141=EDGE_LOOP ( 'NONE', ( #6377, #8624 ) ) ;
#9142=CARTESIAN_POINT ( 'NONE',  ( -10.00000000000000000, 2.500000000000000000, -317.5000000000000000 ) ) ;
#9145=CARTESIAN_POINT ( 'NONE',  ( -15.52898264372803006, 3.840979768096379310, -315.0000000000000000 ) ) ;
#9149=CARTESIAN_POINT ( 'NONE',  ( 9.218822326027003911, 11.18653774893999220, -317.0792622552969533 ) ) ;
#9155=CARTESIAN_POINT ( 'NONE',  ( 11.28358823633007901, -7.096269052248556086, -315.0000000000000568 ) ) ;
#9156=ORIENTED_EDGE ( 'NONE', *, *, #9035, .T. ) ;
#9159=CARTESIAN_POINT ( 'NONE',  ( 6.294344443169999970, 10.85463315985999877, -317.5000000000000000 ) ) ;
#9161=CARTESIAN_POINT ( 'NONE',  ( 15.96001947224000794, -7.545661119572996789, -303.6197174156509391 ) ) ;
#9162=EDGE_CURVE ( 'NONE', #4540, #8127, #4834, .T. ) ;
#9163=CARTESIAN_POINT ( 'NONE',  ( 19.56985579239002959, 0.3946094453810997660, -317.5770954168139610 ) ) ;
#9165=CARTESIAN_POINT ( 'NONE',  ( -17.34693632642999717, -0.4167404706239999923, -314.6383426456000052 ) ) ;
#9167=CARTESIAN_POINT ( 'NONE',  ( 20.01660392705000646, 0.3690847706228002623, -303.6197174156520759 ) ) ;
#9168=CARTESIAN_POINT ( 'NONE',  ( -17.50000000000000000, -3.147917160613439321E-08, 315.0000000000000000 ) ) ;
#9171=CARTESIAN_POINT ( 'NONE',  ( -16.07469914181999826, -3.754035329064000059, -314.6383426456000052 ) ) ;
#9173=CARTESIAN_POINT ( 'NONE',  ( -16.90628502044000214, 5.238535436438000126, -302.5000000000009663 ) ) ;
#9174=ORIENTED_EDGE ( 'NONE', *, *, #2398, .T. ) ;
#9175=CARTESIAN_POINT ( 'NONE',  ( 13.14174346518001535, -9.520659322650999457, 190.4207385301700128 ) ) ;
#9176=CARTESIAN_POINT ( 'NONE',  ( 15.67978886374999803, -4.575336738469999887, -314.4944826805095772 ) ) ;
#9181=CARTESIAN_POINT ( 'NONE',  ( 20.05695074155000768, -0.5616361869861998812, 190.4207385301700128 ) ) ;
#9185=CARTESIAN_POINT ( 'NONE',  ( 16.55686070535999832, -1.955716293870999767, 315.0848619657999734 ) ) ;
#9188=CARTESIAN_POINT ( 'NONE',  ( 14.12295497348999440, -7.525186449763000773, 319.9928079742500131 ) ) ;
#9189=CARTESIAN_POINT ( 'NONE',  ( 19.00000000000000000, 0.000000000000000000, -302.5000000001010108 ) ) ;
#9190=SURFACE_SIDE_STYLE ('',( #3384 ) ) ;
#9191=CARTESIAN_POINT ( 'NONE',  ( 15.56325459994999960, 4.731967449628999844, 314.4150829855000211 ) ) ;
#9197=CARTESIAN_POINT ( 'NONE',  ( 19.21835421908001607, 3.675208614194998447, 319.5792614743400009 ) ) ;
#9199=CARTESIAN_POINT ( 'NONE',  ( 10.54280934634114786, 7.451587612377529091, 315.0000000000000000 ) ) ;
#9202=EDGE_LOOP ( 'NONE', ( #9629, #2711, #8349, #10488 ) ) ;
#9203=CARTESIAN_POINT ( 'NONE',  ( 10.14429053679999981, -9.716529139337000132, -302.5000000000000000 ) ) ;
#9214=CARTESIAN_POINT ( 'NONE',  ( 5.850354798305524184, -8.918567588720486938, -315.0000000000000000 ) ) ;
#9215=EDGE_LOOP ( 'NONE', ( #8747, #370 ) ) ;
#9216=CARTESIAN_POINT ( 'NONE',  ( -17.50000000000000000, 0.000000000000000000, -314.4999343908002061 ) ) ;
#9217=CARTESIAN_POINT ( 'NONE',  ( 0.2363647329299927713, -12.51727884664821033, -316.5000000000004547 ) ) ;
#9219=CARTESIAN_POINT ( 'NONE',  ( -9.038557733644999814, 10.11114377999000169, -317.5000000000000000 ) ) ;
#9220=ORIENTED_EDGE ( 'NONE', *, *, #1423, .F. ) ;
#9221=CARTESIAN_POINT ( 'NONE',  ( 16.86005112630999037, 5.110605191077000065, -317.4928077629770087 ) ) ;
#9223=CARTESIAN_POINT ( 'NONE',  ( -18.87261805073000787, 0.3452380817474001162, -317.4928077629770087 ) ) ;
#9224=CARTESIAN_POINT ( 'NONE',  ( -16.99702983282000091, 1.298346578676000007, -314.8616023057000461 ) ) ;
#9227=CARTESIAN_POINT ( 'NONE',  ( 0.1637764853584998959, 12.51053635490000282, -303.6197174156509391 ) ) ;
#9228=CARTESIAN_POINT ( 'NONE',  ( -16.24790194983231117, -3.755744826583856000, 314.4999487198771817 ) ) ;
#9233=CARTESIAN_POINT ( 'NONE',  ( 19.19804233804001115, -3.716674010855997690, 190.4207385301700128 ) ) ;
#9235=CARTESIAN_POINT ( 'NONE',  ( 15.35654050466421694, 4.050078947852131073, -315.0000000000001137 ) ) ;
#9236=CARTESIAN_POINT ( 'NONE',  ( 19.58491037614999897, 2.818636756334000903, 190.4207385301700128 ) ) ;
#9237=AXIS2_PLACEMENT_3D ( 'NONE', #2692, #5960, #272 ) ;
#9239=CARTESIAN_POINT ( 'NONE',  ( 15.74033075358999945, -3.452242816619000010, 315.0848619657999734 ) ) ;
#9242=CARTESIAN_POINT ( 'NONE',  ( 14.87701781886999086, -6.977856518223995330, 319.9928079742500131 ) ) ;
#9244=CARTESIAN_POINT ( 'NONE',  ( -1.604652252758985043, 9.999950698701082885, 314.4999444147077838 ) ) ;
#9245=CARTESIAN_POINT ( 'NONE',  ( -3.427628718044569478, 12.33061748745338981, -303.4999999999990905 ) ) ;
#9246=CARTESIAN_POINT ( 'NONE',  ( 6.322301096779000318, 8.991223814764000011, 314.8616023057000461 ) ) ;
#9247=EDGE_LOOP ( 'NONE', ( #9835, #4581, #2454, #2829 ) ) ;
#9250=CARTESIAN_POINT ( 'NONE',  ( -16.36040776911000449, 7.306617842034003552, 319.5792614743400009 ) ) ;
#9251=EDGE_CURVE ( 'NONE', #8913, #2473, #2870, .T. ) ;
#9254=CARTESIAN_POINT ( 'NONE',  ( 4.713955699089914297, 9.123860163919065513, 315.0000000000000568 ) ) ;
#9255=CARTESIAN_POINT ( 'NONE',  ( 0.000000000000000000, -7.937240849781000307, -285.0000000000000000 ) ) ;
#9260=CARTESIAN_POINT ( 'NONE',  ( 11.54108047910937174, -7.525558156534593479, 314.4999425153565085 ) ) ;
#9261=CARTESIAN_POINT ( 'NONE',  ( -7.497671121046002973, 10.44264915526000514, 190.0071920248299477 ) ) ;
#9269=CARTESIAN_POINT ( 'NONE',  ( 12.62060098491999938, 8.441142645117002630, 319.9928079742500131 ) ) ;
#9273=VERTEX_POINT ( 'NONE', #9725 ) ;
#9276=CARTESIAN_POINT ( 'NONE',  ( 14.32792941690000177, -7.389020440446000926, -317.4928077629770087 ) ) ;
#9277=CARTESIAN_POINT ( 'NONE',  ( -17.12243801299000268, 0.5826713957640000663, -314.8616023057000461 ) ) ;
#9279=LINE ( 'NONE', #508, #6751 ) ;
#9282=CARTESIAN_POINT ( 'NONE',  ( 1.290325097615000027, -11.49300988401000012, 190.0000000000000000 ) ) ;
#9285=CARTESIAN_POINT ( 'NONE',  ( -8.833609186824004311, -11.21733050393000575, 191.1197171614399792 ) ) ;
#9288=CARTESIAN_POINT ( 'NONE',  ( -4.867894159875999271, 12.21747625305000007, 190.4207385301700128 ) ) ;
#9295=CARTESIAN_POINT ( 'NONE',  ( 15.60880606785999980, -7.925821651060998008, 319.5792614743400009 ) ) ;
#9297=CARTESIAN_POINT ( 'NONE',  ( 15.10708484062000068, -4.236041382665999500, -315.0848619657999734 ) ) ;
#9298=CARTESIAN_POINT ( 'NONE',  ( 17.14610219660000112, 0.04370646908745000336, 314.8616023057000461 ) ) ;
#9301=CARTESIAN_POINT ( 'NONE',  ( -19.19790409518002861, 3.716965664678998582, 319.5792614743400009 ) ) ;
#9304=CARTESIAN_POINT ( 'NONE',  ( 8.691248314156576171, 8.152891913651146183, 315.0000000000001137 ) ) ;
#9305=CARTESIAN_POINT ( 'NONE',  ( 7.006889269069000115, -6.844138725329000472, -284.9999999999999432 ) ) ;
#9313=CARTESIAN_POINT ( 'NONE',  ( 18.87182479219000442, -0.3569112016842001522, 190.0071920248299477 ) ) ;
#9317=DIRECTION ( 'NONE',  ( -3.596898300242126276E-07, -0.9999999999999354960, -1.311545752197542526E-22 ) ) ;
#9320=CARTESIAN_POINT ( 'NONE',  ( 15.63927740852997950, 6.344868560643003974, 319.9928079742500131 ) ) ;
#9325=CARTESIAN_POINT ( 'NONE',  ( -6.380917221297004005, -11.42904134337998734, -317.5770954168139610 ) ) ;
#9327=CARTESIAN_POINT ( 'NONE',  ( -17.35381917807999841, -0.3185724951638000402, -314.6383426456000052 ) ) ;
#9328=CARTESIAN_POINT ( 'NONE',  ( 9.017403168879978281, 8.607149246413721144, -314.5455549245388056 ) ) ;
#9329=B_SPLINE_SURFACE_WITH_KNOTS ( 'NONE', 3, 3, ( 
 ( #7038, #1224, #6218, #5256 ),
 ( #8530, #374, #423, #2038 ),
 ( #9402, #3701, #9451, #8907 ),
 ( #797, #5678, #8101, #8000 ),
 ( #5573, #10409, #3217, #7144 ),
 ( #8856, #4881, #4726, #9660 ),
 ( #6493, #3268, #3864, #5515 ),
 ( #5626, #10515, #7141, #7246 ),
 ( #9607, #7354, #6546, #3965 ),
 ( #2248, #7303, #1608, #3050 ),
 ( #6319, #584, #8797, #1438 ),
 ( #4075, #9825, #10463, #639 ),
 ( #1551, #5462, #3915, #7194 ),
 ( #3103, #6379, #2411, #2301 ),
 ( #3160, #1497, #6436, #4777 ),
 ( #9719, #4022, #4830, #8741 ),
 ( #1383, #8045, #8159, #8965 ),
 ( #695, #743, #2359, #10575 ),
 ( #7942, #4667, #9771, #1057 ),
 ( #8366, #8208, #4131, #2465 ),
 ( #9881, #7406, #4342, #5033 ),
 ( #2625, #3540, #8418, #7616 ),
 ( #1871, #2681, #6707, #8260 ),
 ( #897, #846, #263, #6817 ),
 ( #9128, #9931, #5889, #5836 ),
 ( #5732, #5950, #2569, #207 ),
 ( #9239, #9020, #3428, #4291 ),
 ( #3320, #5142, #7564, #9984 ),
 ( #9185, #3485, #6765, #2518 ),
 ( #6601, #1762, #1656, #10039 ),
 ( #4931, #8315, #4184, #1712 ),
 ( #952, #1820, #45, #5086 ),
 ( #5782, #4239, #6654, #1004 ),
 ( #7511, #153, #9073, #7459 ) ),
 .UNSPECIFIED., .F., .F., .F.,
 ( 4, 1, 1, 1, 1, 1, 1, 1, 1, 1, 1, 1, 1, 1, 1, 1, 1, 1, 1, 1, 1, 1, 1, 1, 1, 1, 1, 1, 1, 1, 1, 4 ),
 ( 4, 4 ),
 ( -0.01574130609828000224, 0.000000000000000000, 0.03448275862069000164, 0.06896551724138000328, 0.1034482758621000087, 0.1379310344828000023, 0.1724137931033999926, 0.2068965517240999863, 0.2413793103448000077, 0.2758620689655000291, 0.3103448275861999672, 0.3448275862069000164, 0.3793103448276000100, 0.4137931034483000037, 0.4482758620689999973, 0.4827586206897000465, 0.5172413793103000090, 0.5517241379310000582, 0.5862068965516999963, 0.6206896551723999345, 0.6551724137930999836, 0.6896551724138000328, 0.7241379310344999709, 0.7586206896552000201, 0.7931034482758999582, 0.8275862068966000074, 0.8620689655171999144, 0.8965517241379000746, 0.9310344827586000127, 0.9655172413793000619, 1.000000000000000000, 1.014026462982999810 ),
 ( -0.1697239316932999953, 1.169834029081999960 ),
 .UNSPECIFIED. ) ;
#9332=CARTESIAN_POINT ( 'NONE',  ( -15.66137281426499861, -7.786477173011506991, 319.0000000000003979 ) ) ;
#9333=ADVANCED_FACE ( 'NONE', ( #3109 ), #4431, .F. ) ;
#9337=CARTESIAN_POINT ( 'NONE',  ( 10.23467949614885164, -10.00000000050611781, -302.4999999999996589 ) ) ;
#9338=CARTESIAN_POINT ( 'NONE',  ( -18.87259549714001139, 0.3457787829170000937, -302.5071922382879279 ) ) ;
#9339=CARTESIAN_POINT ( 'NONE',  ( 6.108404012864005139, 11.90988283206001519, 191.1197171614399792 ) ) ;
#9344=CARTESIAN_POINT ( 'NONE',  ( -20.08924610253000509, -0.07535283344304002928, 319.5792614743400009 ) ) ;
#9345=CARTESIAN_POINT ( 'NONE',  ( 16.55686070535999832, -1.955716293870999767, -315.0848619657999734 ) ) ;
#9346=CARTESIAN_POINT ( 'NONE',  ( -8.551447359560999217, 8.144527334518999240, 315.0848619657999734 ) ) ;
#9351=CARTESIAN_POINT ( 'NONE',  ( -19.49027688392999735, 2.831154404542999714, 318.8802828394900644 ) ) ;
#9353=VECTOR ( 'NONE', #6834, 1000.000000000000000 ) ;
#9356=CARTESIAN_POINT ( 'NONE',  ( -15.00000000000071587, -0.4945770392355663403, 315.0000000000001705 ) ) ;
#9363=CARTESIAN_POINT ( 'NONE',  ( -16.53772850381891857, 2.187491735906824442, -315.0000000000001137 ) ) ;
#9364=CARTESIAN_POINT ( 'NONE',  ( 5.890130794754004029, 10.81842929378999330, 190.0071920248299477 ) ) ;
#9366=CARTESIAN_POINT ( 'NONE',  ( 10.21957842388999893, -9.686567771335999666, -317.5000000000000000 ) ) ;
#9368=EDGE_CURVE ( 'NONE', #1376, #9105, #7610, .T. ) ;
#9370=CARTESIAN_POINT ( 'NONE',  ( 12.75139817577315604, -6.274227700150676768, 315.0000000000000568 ) ) ;
#9371=CARTESIAN_POINT ( 'NONE',  ( 3.903842856253999738, 9.647088721075000706, -314.6383426456000052 ) ) ;
#9372=EDGE_LOOP ( 'NONE', ( #10555, #9064, #1703, #9890, #3299 ) ) ;
#9373=CARTESIAN_POINT ( 'NONE',  ( 14.24138406224000342, 7.443131114976996976, 319.9928079742500131 ) ) ;
#9377=CARTESIAN_POINT ( 'NONE',  ( -16.09890757810000750, 5.925814185855000638, -317.4928077629770087 ) ) ;
#9378=CARTESIAN_POINT ( 'NONE',  ( 6.769722431736004076, -11.85293133419998846, -317.0792622552969533 ) ) ;
#9380=CARTESIAN_POINT ( 'NONE',  ( -17.14577796628000073, 0.02050488658304000164, -314.8616023057000461 ) ) ;
#9383=VERTEX_POINT ( 'NONE', #5564 ) ;
#9384=DIRECTION ( 'NONE',  ( 1.000000000000000000, 0.000000000000000000, 0.000000000000000000 ) ) ;
#9386=CARTESIAN_POINT ( 'NONE',  ( 6.403271823880001712, -11.84773780780999530, 191.1197171614399792 ) ) ;
#9389=CARTESIAN_POINT ( 'NONE',  ( -11.24500836742999610, -9.126642939585995151, -302.5071922382879279 ) ) ;
#9393=CARTESIAN_POINT ( 'NONE',  ( 8.965618380443995505, 10.00899073891999436, -302.5071922382879279 ) ) ;
#9394=CARTESIAN_POINT ( 'NONE',  ( -19.78455541125000750, -1.880268586931002073, 318.8802828394900644 ) ) ;
#9395=CARTESIAN_POINT ( 'NONE',  ( 17.43193685618000188, -1.405086463480999859, -314.4150829855000211 ) ) ;
#9396=CARTESIAN_POINT ( 'NONE',  ( -17.43193685618000188, 1.405086463480999859, 314.4150829855000211 ) ) ;
#9398=CARTESIAN_POINT ( 'NONE',  ( 1.205561540619000116, -11.37600766585000933, 190.0071920248299477 ) ) ;
#9400=CARTESIAN_POINT ( 'NONE',  ( -14.74960734804001916, 8.445183187697006488, 318.8802828394900644 ) ) ;
#9402=CARTESIAN_POINT ( 'NONE',  ( -16.92248268936999978, -0.04189409840125999512, 315.0848619657999734 ) ) ;
#9405=CARTESIAN_POINT ( 'NONE',  ( -20.00000000032979131, -7.322330470066152230, 319.0000000000000568 ) ) ;
#9406=CARTESIAN_POINT ( 'NONE',  ( -15.35654050466420983, -4.050078947852131073, -315.0000000000000568 ) ) ;
#9409=CARTESIAN_POINT ( 'NONE',  ( -17.49999999999999289, 5.867334123212277319, -302.5000000000003411 ) ) ;
#9410=CARTESIAN_POINT ( 'NONE',  ( -13.97602275805729199, 5.383336353019481102, -315.0000000000000568 ) ) ;
#9411=CARTESIAN_POINT ( 'NONE',  ( 11.56561186376999295, 8.976555918559004255, 190.0071920248299477 ) ) ;
#9413=CARTESIAN_POINT ( 'NONE',  ( 2.034678270035999770, -11.44985799554000039, -317.5000000000000000 ) ) ;
#9415=DIRECTION ( 'NONE',  ( 1.000000000000000000, 0.000000000000000000, 0.000000000000000000 ) ) ;
#9417=CARTESIAN_POINT ( 'NONE',  ( 13.82226565756009684, -5.505830577453552088, 315.0000000000000568 ) ) ;
#9418=CARTESIAN_POINT ( 'NONE',  ( 10.58801790939999954, 8.088125079530000150, -314.4150829855000211 ) ) ;
#9424=CARTESIAN_POINT ( 'NONE',  ( -18.99999673287999968, 1.191366929371999993E-07, 191.0000000000000000 ) ) ;
#9425=EDGE_CURVE ( 'NONE', #10392, #563, #8039, .T. ) ;
#9426=CARTESIAN_POINT ( 'NONE',  ( -7.757100520214003758, -11.09835178152000168, -317.5770954168139610 ) ) ;
#9429=CARTESIAN_POINT ( 'NONE',  ( 15.54698342962804958, 4.499693933759708386, -314.5711572504541778 ) ) ;
#9430=VERTEX_POINT ( 'NONE', #3042 ) ;
#9432=CARTESIAN_POINT ( 'NONE',  ( -17.50000000088854435, -5.867334121986939266, 189.9999999999997442 ) ) ;
#9434=CARTESIAN_POINT ( 'NONE',  ( -4.466162596268001828, -12.19410025049000446, 191.1197171614399792 ) ) ;
#9438=EDGE_CURVE ( 'NONE', #2509, #1953, #576, .T. ) ;
#9442=CARTESIAN_POINT ( 'NONE',  ( 10.13603924037000326, 9.590552501249007378, -302.5071922382879279 ) ) ;
#9443=CARTESIAN_POINT ( 'NONE',  ( -19.86662547467000550, -1.900306748470001139, 319.5792614743400009 ) ) ;
#9444=CARTESIAN_POINT ( 'NONE',  ( 17.35381917807999841, 0.3185724951638000402, -314.6383426456000052 ) ) ;
#9445=CARTESIAN_POINT ( 'NONE',  ( -10.40890489166000066, 7.434429060800999522, 315.0848619657999734 ) ) ;
#9446=ORIENTED_EDGE ( 'NONE', *, *, #9035, .F. ) ;
#9447=CARTESIAN_POINT ( 'NONE',  ( -4.308829118669001979, -11.09213725138999962, 190.0071920248299477 ) ) ;
#9449=CARTESIAN_POINT ( 'NONE',  ( 1.327417525529001496, 12.48520226272998990, 318.8802828394900644 ) ) ;
#9451=CARTESIAN_POINT ( 'NONE',  ( -17.36972170382999892, -0.04551883977363000572, 314.6383426456000052 ) ) ;
#9454=CARTESIAN_POINT ( 'NONE',  ( -11.65180110541762382, -6.897852064324583310, -314.9999999999999432 ) ) ;
#9455=CARTESIAN_POINT ( 'NONE',  ( 20.00000000000000355, 25.00000000015544543, 319.0000000000000000 ) ) ;
#9457=CARTESIAN_POINT ( 'NONE',  ( 17.50000000000000711, -8.653813013134384923E-10, -302.5000000000000568 ) ) ;
#9458=CARTESIAN_POINT ( 'NONE',  ( -4.252979419060009647, 9.197563690522738256, -315.0000000000001137 ) ) ;
#9459=CARTESIAN_POINT ( 'NONE',  ( -18.89081873304001036, 0.08752760549136004431, 190.0071920248299477 ) ) ;
#9460=CARTESIAN_POINT ( 'NONE',  ( 17.44863594430761111, 0.8973220660537315485, 314.4999502393481521 ) ) ;
#9462=CARTESIAN_POINT ( 'NONE',  ( -10.11497662670000075, -9.727801543432001097, -317.5000000000000000 ) ) ;
#9464=CARTESIAN_POINT ( 'NONE',  ( 15.26162423979700300, -4.160529437000930031, 314.9999999999999432 ) ) ;
#9465=CARTESIAN_POINT ( 'NONE',  ( 8.519003879469000395, 8.390442916014999142, -314.8616023057000461 ) ) ;
#9468=FACE_OUTER_BOUND ( 'NONE', #7021, .T. ) ;
#9472=CARTESIAN_POINT ( 'NONE',  ( 19.46050885281001896, 1.651188223417001444, -317.5770954168139610 ) ) ;
#9473=CARTESIAN_POINT ( 'NONE',  ( -1.606003227921999343, -12.55439432250999587, -317.0792622552969533 ) ) ;
#9480=CARTESIAN_POINT ( 'NONE',  ( -9.616122863433998802, -9.909251266138999981, 190.0000000000000000 ) ) ;
#9481=CARTESIAN_POINT ( 'NONE',  ( -12.21612826667444374, -9.907025583609534891, 319.0000000000003979 ) ) ;
#9487=CARTESIAN_POINT ( 'NONE',  ( 20.00478054794001537, 0.07382975964161003768, 191.1197171614399792 ) ) ;
#9492=CARTESIAN_POINT ( 'NONE',  ( 19.60176101890002442, 0.3495461351719001408, -302.4229045757450081 ) ) ;
#9493=CARTESIAN_POINT ( 'NONE',  ( -6.490016473005998598, -11.91548699335000272, 319.5792614743400009 ) ) ;
#9494=CARTESIAN_POINT ( 'NONE',  ( 13.24479143485999977, -5.858166912337999577, -315.0848619657999734 ) ) ;
#9495=CARTESIAN_POINT ( 'NONE',  ( -8.620760283086999820, 8.357092890497000326, 314.8616023057000461 ) ) ;
#9496=EDGE_CURVE ( 'NONE', #4386, #8331, #1981, .T. ) ;
#9498=CARTESIAN_POINT ( 'NONE',  ( -19.51240441859933838, -2.792009854621256171, 190.9999999999995737 ) ) ;
#9499=CARTESIAN_POINT ( 'NONE',  ( 10.18759338605000409, 10.75836373329000217, 318.8802828394900644 ) ) ;
#9506=CARTESIAN_POINT ( 'NONE',  ( 19.99999999999999289, -7.322330470418032533, 319.0000000000000568 ) ) ;
#9507=CARTESIAN_POINT ( 'NONE',  ( -16.25556775813545585, -2.760696635281385092, -315.0000000000000000 ) ) ;
#9512=CARTESIAN_POINT ( 'NONE',  ( 0.3940538687071376001, 9.499927474253876625, -315.0000000000000568 ) ) ;
#9513=CARTESIAN_POINT ( 'NONE',  ( 7.457264729102998757, 11.17642278912000720, 189.9229057364800042 ) ) ;
#9514=CARTESIAN_POINT ( 'NONE',  ( 13.64771696944629475, 6.290639922060250910, 314.4999474536516004 ) ) ;
#9516=CARTESIAN_POINT ( 'NONE',  ( -3.336936413097000287, -11.33398029193999967, -317.5000000000000000 ) ) ;
#9521=CARTESIAN_POINT ( 'NONE',  ( 15.40286302630929427, -3.995001727760178145, 315.0000000000000568 ) ) ;
#9522=CARTESIAN_POINT ( 'NONE',  ( 8.655660348039997842, 8.816209662726999241, -314.4150829855000211 ) ) ;
#9523=CARTESIAN_POINT ( 'NONE',  ( 2.881524480432390771E-09, -9.999999999999998224, 314.4999507458384755 ) ) ;
#9524=CARTESIAN_POINT ( 'NONE',  ( -12.76583521038999613, 9.157751700393998107, 320.0770942683900557 ) ) ;
#9527=CARTESIAN_POINT ( 'NONE',  ( 11.49606901914998858, 9.781307837508002478, -317.5770954168139610 ) ) ;
#9528=CARTESIAN_POINT ( 'NONE',  ( -11.49606901914998858, -9.781307837508002478, -317.5770954168139610 ) ) ;
#9529=CARTESIAN_POINT ( 'NONE',  ( -17.50000000000000000, -0.7437989020623000380, -315.0000000000000000 ) ) ;
#9530=CARTESIAN_POINT ( 'NONE',  ( -15.54345086749721716, 4.503564883714276768, -314.5712070352258820 ) ) ;
#9531=VERTEX_POINT ( 'NONE', #10030 ) ;
#9532=CARTESIAN_POINT ( 'NONE',  ( -9.801682940292002044, 9.841837802148999614, 190.0000000000000000 ) ) ;
#9534=CARTESIAN_POINT ( 'NONE',  ( -6.473926368715491542, -11.84005611832666283, 319.0000000000003979 ) ) ;
#9536=CARTESIAN_POINT ( 'NONE',  ( 6.468659092862918847, 11.84071280232868695, -316.5000000000004547 ) ) ;
#9539=CARTESIAN_POINT ( 'NONE',  ( 9.124390749379998056, -10.69353917616999539, -302.4229045757450081 ) ) ;
#9540=CARTESIAN_POINT ( 'NONE',  ( 13.01115177740000384, 9.495820311550003723, 191.1197171614399792 ) ) ;
#9543=CARTESIAN_POINT ( 'NONE',  ( 3.563286991701002382, 11.18699815210999660, -302.5071922382879279 ) ) ;
#9545=CARTESIAN_POINT ( 'NONE',  ( 6.537559671572000575, -9.400791339334000796, -314.4150829855000211 ) ) ;
#9546=CARTESIAN_POINT ( 'NONE',  ( -16.99702983282000091, 1.298346578676000007, 314.8616023057000461 ) ) ;
#9548=FACE_OUTER_BOUND ( 'NONE', #5123, .T. ) ;
#9550=FACE_OUTER_BOUND ( 'NONE', #9215, .T. ) ;
#9554=ORIENTED_EDGE ( 'NONE', *, *, #810, .T. ) ;
#9556=CARTESIAN_POINT ( 'NONE',  ( -15.44313366109816599, 3.946504251847836819, 315.0000000000000568 ) ) ;
#9558=CARTESIAN_POINT ( 'NONE',  ( -4.532042191365901473, -9.152867265080528725, -315.0000000000000568 ) ) ;
#9562=CARTESIAN_POINT ( 'NONE',  ( 1.669371716897545488, 9.454742746653563401, -315.0000000000000000 ) ) ;
#9564=CARTESIAN_POINT ( 'NONE',  ( 14.56080423438999993, 8.072998568875000558, 189.9229057364800042 ) ) ;
#9568=CARTESIAN_POINT ( 'NONE',  ( 18.99984327789000105, -0.5550485914519999175, -317.4999999998989892 ) ) ;
#9571=CARTESIAN_POINT ( 'NONE',  ( 8.636532331090950976, -8.171139803988637595, 315.0000000000000568 ) ) ;
#9573=( BOUNDED_CURVE ( )  B_SPLINE_CURVE ( 3, ( #9813, #9117, #4226, #8149 ),
 .UNSPECIFIED., .F., .F. ) 
 B_SPLINE_CURVE_WITH_KNOTS ( ( 4, 4 ),
 ( 0.000000000000000000, 1.000000000000000000 ),
 .UNSPECIFIED. ) 
 CURVE ( )  GEOMETRIC_REPRESENTATION_ITEM ( )  RATIONAL_B_SPLINE_CURVE ( ( 1.171566417337515764, 0.9428088753385223120, 0.9428111942444009630, 1.171573374055151495 ) ) 
 REPRESENTATION_ITEM ( '' )  );
#9574=CARTESIAN_POINT ( 'NONE',  ( 14.23799507159000122, 5.083276007328000112, -315.0848619657999734 ) ) ;
#9575=CARTESIAN_POINT ( 'NONE',  ( 17.59656075795390606, 5.807225057570236437, 314.4999507458385324 ) ) ;
#9577=CARTESIAN_POINT ( 'NONE',  ( -19.57081977481000834, -0.3814303831828999014, 320.0770942683900557 ) ) ;
#9581=CARTESIAN_POINT ( 'NONE',  ( 18.28030995243001655, 2.924502517761999876, -317.4928077629770087 ) ) ;
#9582=CARTESIAN_POINT ( 'NONE',  ( -14.92964316144998627, -8.327009966606000901, -316.3802825947000201 ) ) ;
#9586=CARTESIAN_POINT ( 'NONE',  ( -17.03769437857130598, -2.221013643562866680, -314.5274634404338485 ) ) ;
#9588=CARTESIAN_POINT ( 'NONE',  ( -9.374494192145073512, 11.05367988180384842, -316.5000000000004547 ) ) ;
#9590=CARTESIAN_POINT ( 'NONE',  ( -15.46063250253144972, -3.925225575964395919, 315.0000000000000568 ) ) ;
#9591=CARTESIAN_POINT ( 'NONE',  ( -18.91993355959997558, -3.215835268190998075, -302.4229045757450081 ) ) ;
#9595=CARTESIAN_POINT ( 'NONE',  ( 3.702588368219998927, 12.37624192652999966, -302.9207377450070453 ) ) ;
#9598=CARTESIAN_POINT ( 'NONE',  ( -1.257430124576000008, -9.427442400486999219, -315.0848619657999734 ) ) ;
#9601=CARTESIAN_POINT ( 'NONE',  ( -18.89053622393001675, -0.06335528492986002014, 190.0071920248299477 ) ) ;
#9602=CARTESIAN_POINT ( 'NONE',  ( 16.34828874915077535, 7.214440038016817880, 190.9999999999996589 ) ) ;
#9604=AXIS2_PLACEMENT_3D ( 'NONE', #8457, #2965, #1297 ) ;
#9607=CARTESIAN_POINT ( 'NONE',  ( -15.07109120124999890, -4.275483045295999318, 315.0848619657999734 ) ) ;
#9609=CARTESIAN_POINT ( 'NONE',  ( -15.63367387165999922, 6.510275065263000371, 320.0000000000000000 ) ) ;
#9610=CARTESIAN_POINT ( 'NONE',  ( -9.801936311039993299, -9.714404437230999889, 319.9928079742500131 ) ) ;
#9612=CARTESIAN_POINT ( 'NONE',  ( -15.44329739658678058, -3.946306641738667409, -314.9999999999999432 ) ) ;
#9613=CARTESIAN_POINT ( 'NONE',  ( -10.00000000000000000, -2.500000000000000000, -315.0000000000000000 ) ) ;
#9617=CARTESIAN_POINT ( 'NONE',  ( -16.39637408479998726, 7.274214857915000998, 190.4207385301700128 ) ) ;
#9618=CARTESIAN_POINT ( 'NONE',  ( 1.514429654104534930E-09, 10.00000000000000000, 189.9999999999998863 ) ) ;
#9627=CARTESIAN_POINT ( 'NONE',  ( -16.76867785761999485, 5.202124494729996940, 319.9928079742500131 ) ) ;
#9629=ORIENTED_EDGE ( 'NONE', *, *, #3001, .F. ) ;
#9630=CARTESIAN_POINT ( 'NONE',  ( -20.05670149355997722, -0.5623089763428000820, -317.0792622552969533 ) ) ;
#9636=EDGE_CURVE ( 'NONE', #135, #9105, #6977, .T. ) ;
#9640=CARTESIAN_POINT ( 'NONE',  ( -17.50000000000000000, 0.000000000000000000, -314.4999343908002061 ) ) ;
#9642=CARTESIAN_POINT ( 'NONE',  ( 19.99999036626000048, 4.642009117057000143E-09, -316.5000000000000000 ) ) ;
#9643=ORIENTED_EDGE ( 'NONE', *, *, #9251, .T. ) ;
#9644=CARTESIAN_POINT ( 'NONE',  ( -15.45559681510979466, -3.931366100772827998, 315.0000000000000000 ) ) ;
#9645=CARTESIAN_POINT ( 'NONE',  ( -5.268482393219001025, -12.14948647186998976, -302.9207377450070453 ) ) ;
#9648=CARTESIAN_POINT ( 'NONE',  ( 6.704579698891996564, 11.86746000475999452, -302.9207377450070453 ) ) ;
#9649=ADVANCED_FACE ( 'NONE', ( #10240, #1102 ), #7662, .T. ) ;
#9651=DIRECTION ( 'NONE',  ( 0.000000000000000000, 1.000000000000000000, 0.000000000000000000 ) ) ;
#9653=CARTESIAN_POINT ( 'NONE',  ( 12.17979804859000126, -7.053762231097000068, -314.6383426456000052 ) ) ;
#9657=CARTESIAN_POINT ( 'NONE',  ( -15.34534221234999585, -7.499749350177997265, 189.9229057364800042 ) ) ;
#9658=CARTESIAN_POINT ( 'NONE',  ( 7.561138155138405814, 11.58431960382585579, 190.9999999999996589 ) ) ;
#9660=CARTESIAN_POINT ( 'NONE',  ( -17.16710485141000220, -2.239552065056999997, 314.4150829855000211 ) ) ;
#9662=CARTESIAN_POINT ( 'NONE',  ( -18.53283357168000123, 2.549981878952999992, 320.0000000000000000 ) ) ;
#9663=CARTESIAN_POINT ( 'NONE',  ( 8.447271450478007537, -10.17170359172999738, 319.9928079742500131 ) ) ;
#9664=CARTESIAN_POINT ( 'NONE',  ( 6.473926368715493318, 11.84005611832666460, 319.0000000000005116 ) ) ;
#9670=CARTESIAN_POINT ( 'NONE',  ( -17.30294281340998452, 5.653404495199006341, 189.9229057364800042 ) ) ;
#9671=CARTESIAN_POINT ( 'NONE',  ( 10.23467949917770525, 9.999999999493887515, 190.0000000000002842 ) ) ;
#9674=CARTESIAN_POINT ( 'NONE',  ( 16.53777229716873265, 2.187293290751350483, 315.0000000000000000 ) ) ;
#9677=CARTESIAN_POINT ( 'NONE',  ( 5.046018101664359712, -12.10925368423180259, -303.4999999999996589 ) ) ;
#9680=B_SPLINE_CURVE_WITH_KNOTS ( 'NONE', 3,
 ( #183, #6739, #2653, #1845, #4090, #3980, #2263, #8174, #4684, #5638, #6507, #7959, #3280 ),
 .UNSPECIFIED., .F., .F.,
 ( 4, 1, 1, 1, 1, 1, 1, 1, 1, 1, 4 ),
 ( 0.000000000000000000, 0.08333333333333001192, 0.1666666666667000196, 0.2500000000000000000, 0.3333333333333000081, 0.5000000000000000000, 0.6666666666667000474, 0.7500000000000000000, 0.8333333333333000637, 0.9166666666667000474, 1.000000000000000000 ),
 .UNSPECIFIED. ) ;
#9681=CARTESIAN_POINT ( 'NONE',  ( -17.27957593929000879, 4.562754682971998932, 319.9928079742500131 ) ) ;
#9682=CIRCLE ( 'NONE', #414, 1.000000000000008882 ) ;
#9686=CARTESIAN_POINT ( 'NONE',  ( 19.57077664853002119, -0.3812814288523002082, -317.5770954168139610 ) ) ;
#9691=CARTESIAN_POINT ( 'NONE',  ( 0.000000000000000000, 0.000000000000000000, -317.5000000000000000 ) ) ;
#9695=( GEOMETRIC_REPRESENTATION_CONTEXT ( 3 ) GLOBAL_UNCERTAINTY_ASSIGNED_CONTEXT ( ( #1634 ) ) GLOBAL_UNIT_ASSIGNED_CONTEXT ( ( #4296, #5787, #903 ) ) REPRESENTATION_CONTEXT ( 'NONE', 'WORKASPACE' ) );
#9699=CARTESIAN_POINT ( 'NONE',  ( 9.195128512800469167, 11.11313767369120953, -316.5000000000004547 ) ) ;
#9700=ORIENTED_EDGE ( 'NONE', *, *, #833, .F. ) ;
#9701=CARTESIAN_POINT ( 'NONE',  ( -8.021995032228604217, -8.375907102466543463, 315.0000000000000568 ) ) ;
#9702=CARTESIAN_POINT ( 'NONE',  ( -1.988818824435997890, -12.53224469152999099, -302.9207377450070453 ) ) ;
#9708=CARTESIAN_POINT ( 'NONE',  ( 13.92883798546999508, 9.075834183867002025, -302.9207377450070453 ) ) ;
#9709=CARTESIAN_POINT ( 'NONE',  ( 19.77468550638000266, -1.920668048511998904, 318.8802828394900644 ) ) ;
#9711=CARTESIAN_POINT ( 'NONE',  ( -11.99990625867999938, -6.898016740823000426, -314.8616023057000461 ) ) ;
#9713=ORIENTED_EDGE ( 'NONE', *, *, #2673, .T. ) ;
#9714=CARTESIAN_POINT ( 'NONE',  ( -18.45932313982999062, -2.405278989253002209, 190.0071920248299477 ) ) ;
#9715=CARTESIAN_POINT ( 'NONE',  ( -4.856005603318366504, 12.14126555804866570, 190.9999999999996589 ) ) ;
#9719=CARTESIAN_POINT ( 'NONE',  ( -3.846123575835999731, -9.203727088275000412, 315.0848619657999734 ) ) ;
#9722=CARTESIAN_POINT ( 'NONE',  ( -18.14104367554000774, -3.149620910056999623, 319.9928079742500131 ) ) ;
#9725=CARTESIAN_POINT ( 'NONE',  ( 16.99996037728000076, -1.352915776343000118E-09, 314.9999801883000146 ) ) ;
#9727=CARTESIAN_POINT ( 'NONE',  ( 0.000000000000000000, 7.937240849781000307, -285.0000000000000000 ) ) ;
#9728=CARTESIAN_POINT ( 'NONE',  ( 17.32898823752001860, 5.623515075799002894, 189.9229057364800042 ) ) ;
#9731=CARTESIAN_POINT ( 'NONE',  ( 13.97618761079829142, 5.383201530108604693, 314.9999999999999432 ) ) ;
#9732=CARTESIAN_POINT ( 'NONE',  ( 19.86889125890001040, -1.746333262808030584, -303.5000000000005684 ) ) ;
#9733=CARTESIAN_POINT ( 'NONE',  ( 17.35477687787999912, -0.3068793820639000303, -314.6383426456000052 ) ) ;
#9736=CARTESIAN_POINT ( 'NONE',  ( -17.73249602794001234, 3.891729847315997581, 319.9928079742500131 ) ) ;
#9739=ORIENTED_EDGE ( 'NONE', *, *, #2673, .F. ) ;
#9740=CARTESIAN_POINT ( 'NONE',  ( 17.71107981743001503, 5.830323931021004213, -316.3802825947000201 ) ) ;
#9744=CARTESIAN_POINT ( 'NONE',  ( 14.17215049938999982, -7.636433089049000422, 320.0000000000000000 ) ) ;
#9748=CARTESIAN_POINT ( 'NONE',  ( -17.50000000000000000, 0.000000000000000000, -314.4999343908002061 ) ) ;
#9750=CARTESIAN_POINT ( 'NONE',  ( -17.27223423031420069, -1.573973318776765717, -314.5135302205611083 ) ) ;
#9752=CARTESIAN_POINT ( 'NONE',  ( -10.59678593799237944, 10.61334907845371411, -316.5000000000004547 ) ) ;
#9754=CARTESIAN_POINT ( 'NONE',  ( 0.3943348293965602824, -9.499921225251823031, 315.0000000000000000 ) ) ;
#9755=CARTESIAN_POINT ( 'NONE',  ( -12.62193639354000396, -9.236300292413996971, -302.4229045757450081 ) ) ;
#9759=( NAMED_UNIT ( * ) PLANE_ANGLE_UNIT ( ) SI_UNIT ( $, .RADIAN. ) );
#9760=CARTESIAN_POINT ( 'NONE',  ( 18.60584266697000544, 4.788593885995998889, -302.9207377450070453 ) ) ;
#9761=CARTESIAN_POINT ( 'NONE',  ( 19.12221666159999600, -3.679580603257996962, 318.8802828394900644 ) ) ;
#9763=CARTESIAN_POINT ( 'NONE',  ( 1.419551022038999966, -10.09154694854999867, -314.4150829855000211 ) ) ;
#9764=EDGE_CURVE ( 'NONE', #9430, #4467, #7018, .T. ) ;
#9767=CARTESIAN_POINT ( 'NONE',  ( 19.59090808375999515, -0.09664295149309998223, 189.9229057364800042 ) ) ;
#9768=CARTESIAN_POINT ( 'NONE',  ( 19.96251415050937439, 0.9422375983257499366, 190.9999999999996589 ) ) ;
#9769=CARTESIAN_POINT ( 'NONE',  ( -0.7884827272773663465, 9.499887003984509803, -315.0000000000000568 ) ) ;
#9771=CARTESIAN_POINT ( 'NONE',  ( 4.031301020048999817, -9.630010295875997883, 314.6383426456000052 ) ) ;
#9773=CARTESIAN_POINT ( 'NONE',  ( -7.333949653644999955, 10.60950709473999964, 320.0000000000000000 ) ) ;
#9775=CARTESIAN_POINT ( 'NONE',  ( 15.66137281426500572, 7.786477173011509656, 319.0000000000005116 ) ) ;
#9776=CARTESIAN_POINT ( 'NONE',  ( -1.514431797236434930E-09, -10.00000000000000000, 190.0000000000000000 ) ) ;
#9778=ORIENTED_EDGE ( 'NONE', *, *, #9983, .T. ) ;
#9784=CARTESIAN_POINT ( 'NONE',  ( 20.00000000435078107, -7.322330466941333604, -316.5000000000000000 ) ) ;
#9786=CARTESIAN_POINT ( 'NONE',  ( 16.99953299605537183, 0.4334412736564768331, 315.0000000000000568 ) ) ;
#9788=CARTESIAN_POINT ( 'NONE',  ( 19.32402384659099326, -3.348155292981250586, -303.4999999999996589 ) ) ;
#9789=CARTESIAN_POINT ( 'NONE',  ( -13.34617449956999913, -8.168334506422000985, -302.5000000000000000 ) ) ;
#9792=CARTESIAN_POINT ( 'NONE',  ( 19.86662547467000550, 1.900306748470001139, 319.5792614743400009 ) ) ;
#9796=CARTESIAN_POINT ( 'NONE',  ( -6.751314262718001835, 11.77064546103999731, -316.3802825947000201 ) ) ;
#9798=CARTESIAN_POINT ( 'NONE',  ( -11.66516470684000772, -10.15894662545001381, -316.3802825947000201 ) ) ;
#9800=CARTESIAN_POINT ( 'NONE',  ( -16.29068328802999943, -5.892689959824000567, 320.0000000000000000 ) ) ;
#9803=CARTESIAN_POINT ( 'NONE',  ( 8.778856717165009371, -8.123403389731517876, -315.0000000000001137 ) ) ;
#9805=CARTESIAN_POINT ( 'NONE',  ( -15.67978886374999803, 4.575336738469999887, -314.4963898845653603 ) ) ;
#9806=VERTEX_POINT ( 'NONE', #7864 ) ;
#9809=CARTESIAN_POINT ( 'NONE',  ( 17.74191744551998795, -5.793625128177000150, -303.6197174156509391 ) ) ;
#9811=CARTESIAN_POINT ( 'NONE',  ( -13.57573464316000056, -3.225916527208000151, 315.0000000000000000 ) ) ;
#9812=CARTESIAN_POINT ( 'NONE',  ( -19.56988197685000230, -0.3940236285954000772, -302.4229045757450081 ) ) ;
#9813=CARTESIAN_POINT ( 'NONE',  ( 19.00000000000000000, 0.000000000000000000, -302.5000000001010108 ) ) ;
#9815=CARTESIAN_POINT ( 'NONE',  ( -16.89608781496000134, -0.5923740909019999945, -315.0848619657999734 ) ) ;
#9816=CARTESIAN_POINT ( 'NONE',  ( -11.28854116844999922, 9.238965579841000419, -302.5000000000000000 ) ) ;
#9819=CARTESIAN_POINT ( 'NONE',  ( -17.86997157320001151, -4.940892756443005851, 189.9229057364800042 ) ) ;
#9821=CARTESIAN_POINT ( 'NONE',  ( 10.90988923471839023, 7.272053090123300478, -315.0000000000000000 ) ) ;
#9825=CARTESIAN_POINT ( 'NONE',  ( -11.99990625867999938, -6.898016740823000426, 314.8616023057000461 ) ) ;
#9827=CARTESIAN_POINT ( 'NONE',  ( -18.99998145310000197, 0.3132853329045000024, 319.9999999999899956 ) ) ;
#9829=CARTESIAN_POINT ( 'NONE',  ( 17.73249602794001234, -3.891729847315997581, 319.9928079742500131 ) ) ;
#9830=CARTESIAN_POINT ( 'NONE',  ( -19.78167965760190938, 1.922413304792618405, 319.0000000000005116 ) ) ;
#9831=FILL_AREA_STYLE_COLOUR ( '', #3176 ) ;
#9834=CARTESIAN_POINT ( 'NONE',  ( -11.28781796570999951, 4.951468039558000633, -285.0000000000000000 ) ) ;
#9835=ORIENTED_EDGE ( 'NONE', *, *, #8771, .F. ) ;
#9836=EDGE_CURVE ( 'NONE', #6747, #563, #2980, .T. ) ;
#9840=( BOUNDED_CURVE ( )  B_SPLINE_CURVE ( 3, ( #7839, #9409, #538, #1996, #7737, #487, #9457 ),
 .UNSPECIFIED., .F., .T. ) 
 B_SPLINE_CURVE_WITH_KNOTS ( ( 4, 3, 4 ),
 ( 0.006576891535901297804, 0.5000000000000000000, 0.9934231084340220397 ),
 .UNSPECIFIED. ) 
 CURVE ( )  GEOMETRIC_REPRESENTATION_ITEM ( )  RATIONAL_B_SPLINE_CURVE ( ( 0.9922222088160741471, 0.8003084355042745512, 0.8029010325655832059, 1.000000000000000000, 0.8029010325775973733, 0.8003084355045906317, 0.9922222087809797753 ) ) 
 REPRESENTATION_ITEM ( '' )  );
#9842=CARTESIAN_POINT ( 'NONE',  ( 13.93992802816216781, -8.979094264391768832, -303.4999999999996589 ) ) ;
#9843=CARTESIAN_POINT ( 'NONE',  ( 15.89383674730000173, 3.622219875512000087, -314.8616023057000461 ) ) ;
#9845=CARTESIAN_POINT ( 'NONE',  ( -18.53285823922000120, 2.549737172213000225, 190.0000000000000000 ) ) ;
#9847=CARTESIAN_POINT ( 'NONE',  ( -13.57573464316000056, 3.225916527208000151, 315.0000000000001705 ) ) ;
#9849=CARTESIAN_POINT ( 'NONE',  ( 18.60752753902997725, 4.785892219302998463, -317.0792622552969533 ) ) ;
#9853=CARTESIAN_POINT ( 'NONE',  ( -18.95677580539999951, -0.9180370088860999589, 320.0000000000000000 ) ) ;
#9857=CARTESIAN_POINT ( 'NONE',  ( 3.689485142014392149, -9.275849510248951546, -314.9999999999999432 ) ) ;
#9859=CARTESIAN_POINT ( 'NONE',  ( 9.847343584659233429, -8.231878686604515494, -314.5529121822860361 ) ) ;
#9862=CARTESIAN_POINT ( 'NONE',  ( -14.34749558092999777, 7.521529436904000221, -317.5000000000000000 ) ) ;
#9863=EDGE_LOOP ( 'NONE', ( #7439, #4272, #3460, #7862 ) ) ;
#9864=CARTESIAN_POINT ( 'NONE',  ( 9.278531818924999897, -11.16715007748999078, -302.9207377450070453 ) ) ;
#9866=CARTESIAN_POINT ( 'NONE',  ( 3.713744197507001576, -11.87335072286999527, -317.5770954168139610 ) ) ;
#9867=CARTESIAN_POINT ( 'NONE',  ( -14.79012398733999945, -1.483731117707000058, 315.0000000000000000 ) ) ;
#9870=CARTESIAN_POINT ( 'NONE',  ( -19.95943119690998557, 1.720147047185998757, -302.9207377450070453 ) ) ;
#9871=CARTESIAN_POINT ( 'NONE',  ( -17.50000000000000000, 1.896400240175167841E-08, 314.4999014931028682 ) ) ;
#9873=CARTESIAN_POINT ( 'NONE',  ( -17.56970546055000071, 0.4338786413876999926, -314.4150829855000211 ) ) ;
#9876=CARTESIAN_POINT ( 'NONE',  ( -18.27235334878999851, -5.234940180598000481, 190.4207385301700128 ) ) ;
#9877=CARTESIAN_POINT ( 'NONE',  ( -8.037373804805000077, -9.179324345868998591, -314.4944826805095772 ) ) ;
#9878=CARTESIAN_POINT ( 'NONE',  ( 11.54764063961475351, 6.952680983979389495, -315.0000000000000000 ) ) ;
#9881=CARTESIAN_POINT ( 'NONE',  ( 8.551447359560999217, -8.144527334518999240, 315.0848619657999734 ) ) ;
#9882=B_SPLINE_CURVE_WITH_KNOTS ( 'NONE', 3,
 ( #6518, #9046, #9853, #769, #718, #1681, #8076, #1472, #1632, #9800, #3352, #820, #4051, #70, #2437, #6570, #6627, #8022, #4905, #3991, #8184, #3241, #7380, #6409, #4154, #2275, #15, #3289, #1522, #2492, #4955, #7222, #10489, #10548, #3190, #9744, #6462, #5650, #8231, #868, #1579, #4856, #9956, #6792, #10064, #8283, #6735, #7640 ),
 .UNSPECIFIED., .F., .F.,
 ( 4, 1, 1, 1, 1, 1, 1, 1, 1, 1, 1, 1, 1, 1, 1, 1, 1, 1, 1, 1, 1, 1, 1, 1, 1, 1, 1, 1, 1, 1, 1, 1, 1, 1, 1, 1, 1, 1, 1, 1, 1, 1, 1, 1, 1, 4 ),
 ( 0.000000000000000000, 0.02222222222221999915, 0.04444444444443999831, 0.06666666666666999641, 0.08888888888889000250, 0.1111111111111000027, 0.1333333333332999970, 0.1555555555555999947, 0.1777777777777999890, 0.2000000000000000111, 0.2222222222222000054, 0.2444444444443999997, 0.2666666666666999697, 0.2888888888889000195, 0.3111111111111000138, 0.3333333333333000081, 0.3555555555556000336, 0.3777777777777999724, 0.4000000000000000222, 0.4222222222221999610, 0.4444444444444000109, 0.4666666666666999808, 0.4888888888889000306, 0.5111111111110999694, 0.5333333333333000192, 0.5555555555555999891, 0.5777777777778000390, 0.5999999999999999778, 0.6222222222222000276, 0.6444444444443999664, 0.6666666666667000474, 0.6888888888888999862, 0.7111111111111000360, 0.7333333333333000859, 0.7555555555556000558, 0.7777777777777999946, 0.8000000000000000444, 0.8222222222221999832, 0.8444444444443999220, 0.8666666666667000030, 0.8888888888888999418, 0.9111111111110999916, 0.9333333333333000414, 0.9555555555556000114, 0.9777777777778000612, 1.000000000000000000 ),
 .UNSPECIFIED. ) ;
#9884=CARTESIAN_POINT ( 'NONE',  ( 18.75085780967000559, -3.496151560526002289, 320.0770942683900557 ) ) ;
#9885=CARTESIAN_POINT ( 'NONE',  ( -7.495586483745387163, 11.60098025501653929, 319.0000000000005116 ) ) ;
#9886=CARTESIAN_POINT ( 'NONE',  ( 15.89383674730000173, 3.622219875512000087, 314.8616023057000461 ) ) ;
#9888=CARTESIAN_POINT ( 'NONE',  ( 19.49681644515301215, -2.834072041603171499, 190.9999999999995737 ) ) ;
#9890=ORIENTED_EDGE ( 'NONE', *, *, #9368, .F. ) ;
#9891=EDGE_CURVE ( 'NONE', #9921, #4804, #6189, .T. ) ;
#9899=CARTESIAN_POINT ( 'NONE',  ( -14.24871951745999965, 7.583581010724000038, 190.0000000000000000 ) ) ;
#9902=CARTESIAN_POINT ( 'NONE',  ( 15.00000000000325784, -8.632726818195413123E-17, 315.0000000000001705 ) ) ;
#9904=CARTESIAN_POINT ( 'NONE',  ( -12.86351645698000645, 9.576920946250998767, -316.3802825947000201 ) ) ;
#9908=CARTESIAN_POINT ( 'NONE',  ( -0.9838506439437841866, -9.488399989288446079, -315.0000000000000000 ) ) ;
#9910=CARTESIAN_POINT ( 'NONE',  ( 17.48550435259292612, -0.4594173590775665339, -314.5005290240521276 ) ) ;
#9913=EDGE_LOOP ( 'NONE', ( #350, #675, #1637, #10146 ) ) ;
#9914=CARTESIAN_POINT ( 'NONE',  ( 5.058393412147005108, -12.18538300202998315, -302.9207377450070453 ) ) ;
#9915=FACE_OUTER_BOUND ( 'NONE', #3097, .T. ) ;
#9919=CARTESIAN_POINT ( 'NONE',  ( -17.22664556233274880, -1.821222559103062633, 314.4999497328576012 ) ) ;
#9920=( BOUNDED_CURVE ( )  B_SPLINE_CURVE ( 3, ( #1117, #2735, #7674, #1168 ),
 .UNSPECIFIED., .F., .T. ) 
 B_SPLINE_CURVE_WITH_KNOTS ( ( 4, 4 ),
 ( 1.073606735059035064E-09, 1.000000000000000000 ),
 .UNSPECIFIED. ) 
 CURVE ( )  GEOMETRIC_REPRESENTATION_ITEM ( )  RATIONAL_B_SPLINE_CURVE ( ( 0.9922222082322698089, 0.8003084355095323454, 0.8029010327654424461, 1.000000000000000000 ) ) 
 REPRESENTATION_ITEM ( '' )  );
#9921=VERTEX_POINT ( 'NONE', #9216 ) ;
#9922=CARTESIAN_POINT ( 'NONE',  ( -16.54291557298000370, -1.991497705781999805, -315.0848619657999734 ) ) ;
#9925=CARTESIAN_POINT ( 'NONE',  ( -11.06049270995999123, -10.50744457173999713, 190.4207385301700128 ) ) ;
#9930=CARTESIAN_POINT ( 'NONE',  ( -19.49006540358000805, 2.831553480999998929, 191.1197171614399792 ) ) ;
#9931=CARTESIAN_POINT ( 'NONE',  ( 14.43094748301999886, -5.211771040651000497, 314.8616023057000461 ) ) ;
#9933=CARTESIAN_POINT ( 'NONE',  ( -19.38188031595998595, -1.781951755297001450, 320.0770942683900557 ) ) ;
#9935=CARTESIAN_POINT ( 'NONE',  ( -6.533799827619673373, 11.82671337997188132, -303.5000000000000000 ) ) ;
#9936=CARTESIAN_POINT ( 'NONE',  ( 6.370857846455999507, 9.209451711050000711, 314.6383426456000052 ) ) ;
#9940=ADVANCED_FACE ( 'NONE', ( #777 ), #2804, .F. ) ;
#9942=CARTESIAN_POINT ( 'NONE',  ( 2.737043330023148258, 9.374968016864249520, 315.0000000000000568 ) ) ;
#9951=CARTESIAN_POINT ( 'NONE',  ( -16.39029893813008343, 2.501810464458257943, -315.0000000000000568 ) ) ;
#9954=CARTESIAN_POINT ( 'NONE',  ( -19.31691132429000390, 3.346581979927999217, -316.3802825947000201 ) ) ;
#9956=CARTESIAN_POINT ( 'NONE',  ( 18.20355969383999906, -3.293069710501999925, 320.0000000000000000 ) ) ;
#9960=CARTESIAN_POINT ( 'NONE',  ( 8.021995458420214220, -8.375882622524637000, -315.0000000000000000 ) ) ;
#9963=CARTESIAN_POINT ( 'NONE',  ( -17.50000000000126832, 0.7437989020612977287, -315.0000000000001705 ) ) ;
#9964=ORIENTED_EDGE ( 'NONE', *, *, #7521, .F. ) ;
#9967=CARTESIAN_POINT ( 'NONE',  ( 13.93620031452002728, -8.972937827676991773, -303.6197174156509391 ) ) ;
#9968=CARTESIAN_POINT ( 'NONE',  ( -14.29183324405000732, -7.414293696095001884, -317.4928077629770087 ) ) ;
#9972=CARTESIAN_POINT ( 'NONE',  ( -18.63306024686997375, 4.746768565380000027, -302.9207377450070453 ) ) ;
#9973=CARTESIAN_POINT ( 'NONE',  ( 2.381287022736665303E-07, -10.00000000000000000, 315.0000000000000000 ) ) ;
#9976=CARTESIAN_POINT ( 'NONE',  ( -18.32597195921000122, 3.115684853309999891, -302.5000000000129603 ) ) ;
#9978=CARTESIAN_POINT ( 'NONE',  ( -19.56039901294001737, 0.5262506252543003304, 189.9229057364800042 ) ) ;
#9979=CARTESIAN_POINT ( 'NONE',  ( 12.98706127646999953, -6.788989183774999603, -314.4944826805095772 ) ) ;
#9982=CARTESIAN_POINT ( 'NONE',  ( -4.854896540501004054, 12.13415599451999682, 191.1197171614399792 ) ) ;
#9983=EDGE_CURVE ( 'NONE', #9531, #8110, #3136, .T. ) ;
#9984=CARTESIAN_POINT ( 'NONE',  ( 16.80445917461999983, -3.015803745947999825, 314.4150829855000211 ) ) ;
#9986=CARTESIAN_POINT ( 'NONE',  ( -16.74680747859001784, -6.256295688539003308, 320.0770942683900557 ) ) ;
#9988=CARTESIAN_POINT ( 'NONE',  ( -8.203579748838807362, 8.842447418481361510, 314.4999432750971096 ) ) ;
#9989=CARTESIAN_POINT ( 'NONE',  ( -10.52063983335276554, 10.64371280159997823, -303.5000000000000000 ) ) ;
#9990=CARTESIAN_POINT ( 'NONE',  ( 10.41198510038999991, 7.677033091942000453, 314.8616023057000461 ) ) ;
#9993=CARTESIAN_POINT ( 'NONE',  ( 19.50549492440999089, 2.789745814424999359, 318.8802828394900644 ) ) ;
#9997=CARTESIAN_POINT ( 'NONE',  ( 8.900624420096743705, 8.081841135676405941, 314.9999999999999432 ) ) ;
#10014=CARTESIAN_POINT ( 'NONE',  ( 13.12058949809353514, -6.031889286829740904, -315.0000000000000000 ) ) ;
#10016=CARTESIAN_POINT ( 'NONE',  ( 15.84610571802257795, -4.157530358492036449, -314.5664817403809934 ) ) ;
#10017=CARTESIAN_POINT ( 'NONE',  ( 19.32351226214660045, -3.349534253028545905, -316.5000000000004547 ) ) ;
#10021=CARTESIAN_POINT ( 'NONE',  ( 16.93986923087000562, -6.779672025222003739, -302.9207377450070453 ) ) ;
#10022=ADVANCED_FACE ( 'NONE', ( #9468 ), #8065, .T. ) ;
#10023=CARTESIAN_POINT ( 'NONE',  ( -15.21494798568001627, -6.716444321683999519, -317.4928077629770087 ) ) ;
#10024=CARTESIAN_POINT ( 'NONE',  ( -16.92217352393999974, 0.01966449385449000123, -315.0848619657999734 ) ) ;
#10025=CARTESIAN_POINT ( 'NONE',  ( -16.01368207331000093, 7.610776120867003947, -302.9207377450070453 ) ) ;
#10026=CARTESIAN_POINT ( 'NONE',  ( -17.50000003227012613, 5.857864393370423528, 314.4997059534069308 ) ) ;
#10030=CARTESIAN_POINT ( 'NONE',  ( -16.99996037728000076, 1.352916227065999958E-09, 314.9999801883000146 ) ) ;
#10032=CARTESIAN_POINT ( 'NONE',  ( 19.98387668437998954, 0.4031290841193003183, 191.1197171614399792 ) ) ;
#10034=CARTESIAN_POINT ( 'NONE',  ( 15.42284054825286432, 3.971008657351323468, -314.9999999999999432 ) ) ;
#10036=CARTESIAN_POINT ( 'NONE',  ( 6.124940582141004342, 11.99257230354999315, 190.4207385301700128 ) ) ;
#10039=CARTESIAN_POINT ( 'NONE',  ( 17.43193685618000188, -1.405086463480999859, 314.4150829855000211 ) ) ;
#10042=CARTESIAN_POINT ( 'NONE',  ( 17.29814430729002339, -5.659421966102000212, 320.0770942683900557 ) ) ;
#10045=CARTESIAN_POINT ( 'NONE',  ( 15.23514566747999943, 4.427644513407000382, 314.8616023057000461 ) ) ;
#10047=CARTESIAN_POINT ( 'NONE',  ( 18.68747751655416423, -4.479206664350978251, 190.9999999999995737 ) ) ;
#10049=CARTESIAN_POINT ( 'NONE',  ( 10.21681110195000031, 10.83745499882999574, 319.5792614743400009 ) ) ;
#10052=CARTESIAN_POINT ( 'NONE',  ( -8.586872910504615319, 8.187582572610192955, 315.0000000000000568 ) ) ;
#10053=CARTESIAN_POINT ( 'NONE',  ( -14.79012398733999945, -1.483731117707000058, -285.0000000000000000 ) ) ;
#10056=CARTESIAN_POINT ( 'NONE',  ( 1.646600138488000020, -11.47371312023999934, -302.5000000000000000 ) ) ;
#10058=CARTESIAN_POINT ( 'NONE',  ( 17.35547125580999861, 4.661453509011000307, 190.0000000000000000 ) ) ;
#10059=CARTESIAN_POINT ( 'NONE',  ( -15.45543459605808145, 3.931565522428363213, -315.0000000000000568 ) ) ;
#10061=CARTESIAN_POINT ( 'NONE',  ( 16.79769345205001585, 5.168336178625003718, 190.0071920248299477 ) ) ;
#10064=CARTESIAN_POINT ( 'NONE',  ( 18.78787853991000034, -1.761062637770999917, 320.0000000000000000 ) ) ;
#10071=FACE_OUTER_BOUND ( 'NONE', #5829, .T. ) ;
#10075=CARTESIAN_POINT ( 'NONE',  ( 19.56018822079001040, 0.5268747006259002497, -317.5770954168139610 ) ) ;
#10076=CARTESIAN_POINT ( 'NONE',  ( -16.10362618234000109, 3.713712614977999760, -314.6383426456000052 ) ) ;
#10077=CARTESIAN_POINT ( 'NONE',  ( -19.98289592923002544, -0.4160572288964003440, -303.6197174156509391 ) ) ;
#10079=ORIENTED_EDGE ( 'NONE', *, *, #3389, .T. ) ;
#10080=CARTESIAN_POINT ( 'NONE',  ( 18.53285823922000120, -2.549737172213000225, 190.0000000000000000 ) ) ;
#10084=CARTESIAN_POINT ( 'NONE',  ( 10.15702342499999844, -10.85948264422000165, 190.4207385301700128 ) ) ;
#10086=CARTESIAN_POINT ( 'NONE',  ( 18.29625743176001862, -2.888693746018001107, -302.5071922382879279 ) ) ;
#10087=CARTESIAN_POINT ( 'NONE',  ( 2.655864369898997435, 12.48600887025999029, 190.4207385301700128 ) ) ;
#10088=VECTOR ( 'NONE', #2332, 1000.000000000000000 ) ;
#10090=EDGE_CURVE ( 'NONE', #1085, #10392, #10265, .T. ) ;
#10092=CARTESIAN_POINT ( 'NONE',  ( 0.6354225718825003977, -12.59144946217000260, 319.5792614743400009 ) ) ;
#10094=CARTESIAN_POINT ( 'NONE',  ( -15.42213741511416458, 4.758712124319814940, 314.4999411224990240 ) ) ;
#10095=CARTESIAN_POINT ( 'NONE',  ( 17.12432750374000179, 0.4000877216259000058, -314.8616023057000461 ) ) ;
#10096=CARTESIAN_POINT ( 'NONE',  ( 16.54291557298000370, 1.991497705781999805, 315.0848619657999734 ) ) ;
#10098=CARTESIAN_POINT ( 'NONE',  ( -6.109815047729933113, -11.91693857169684989, 190.9999999999995737 ) ) ;
#10099=CARTESIAN_POINT ( 'NONE',  ( 18.77791317464001608, 4.479224074632002228, 319.5792614743400009 ) ) ;
#10101=CARTESIAN_POINT ( 'NONE',  ( -4.603463306792016319, 9.141632142122212201, 315.0000000000000568 ) ) ;
#10104=CARTESIAN_POINT ( 'NONE',  ( -7.774319915545000015, -10.49237824600999858, -302.5000000000000000 ) ) ;
#10106=CARTESIAN_POINT ( 'NONE',  ( 16.27511603407000251, 5.909078865696000271, 190.0000000000000000 ) ) ;
#10107=CARTESIAN_POINT ( 'NONE',  ( 3.206477836452071184, -9.870911208880196241, 314.4999441614608031 ) ) ;
#10108=CARTESIAN_POINT ( 'NONE',  ( 12.48652197162000554, 8.514177154860004038, 190.0071920248299477 ) ) ;
#10114=DIRECTION ( 'NONE',  ( 0.000000000000000000, 0.000000000000000000, 1.000000000000000000 ) ) ;
#10116=CARTESIAN_POINT ( 'NONE',  ( 17.75416867407000154, 3.856294574926997232, 319.9928079742500131 ) ) ;
#10121=CARTESIAN_POINT ( 'NONE',  ( -3.630810623869999976, 11.17897874952999793, -317.4928077629770087 ) ) ;
#10122=CIRCLE ( 'NONE', #6868, 1.000000000000021982 ) ;
#10123=CARTESIAN_POINT ( 'NONE',  ( -19.46050885281001896, -1.651188223417001444, -317.5770954168139610 ) ) ;
#10124=CARTESIAN_POINT ( 'NONE',  ( -15.27200851150000105, 4.387263554753999983, -314.8616023057000461 ) ) ;
#10129=CARTESIAN_POINT ( 'NONE',  ( -15.64479012893000132, -6.500532800106000764, 190.0000000000000000 ) ) ;
#10132=CARTESIAN_POINT ( 'NONE',  ( -19.86884641856056888, 1.746738893747494803, -316.5000000000005116 ) ) ;
#10136=CARTESIAN_POINT ( 'NONE',  ( -12.15874467096999645, 9.926591843472005294, 191.1197171614399792 ) ) ;
#10141=CARTESIAN_POINT ( 'NONE',  ( -20.05691220054001178, 0.5621708077868997622, 319.5792614743400009 ) ) ;
#10143=CARTESIAN_POINT ( 'NONE',  ( -13.24479143485999977, 5.858166912337999577, 315.0848619657999734 ) ) ;
#10145=CARTESIAN_POINT ( 'NONE',  ( -16.34828874915077179, -7.214440038016814327, 190.9999999999995737 ) ) ;
#10146=ORIENTED_EDGE ( 'NONE', *, *, #6263, .T. ) ;
#10147=CARTESIAN_POINT ( 'NONE',  ( 9.073652982438993320, 11.14186456285000126, 318.8802828394900644 ) ) ;
#10152=CARTESIAN_POINT ( 'NONE',  ( -0.3943348293965602824, 9.499921225251823031, 315.0000000000000000 ) ) ;
#10153=CARTESIAN_POINT ( 'NONE',  ( -11.71572875295034066, -12.49999999989693755, 319.0000000000000568 ) ) ;
#10157=CARTESIAN_POINT ( 'NONE',  ( 15.42213744428624267, -4.758712092923055970, 314.4999411224989103 ) ) ;
#10159=CARTESIAN_POINT ( 'NONE',  ( -9.745026809365992193, 9.735374599634990744, 190.0071920248299477 ) ) ;
#10164=CARTESIAN_POINT ( 'NONE',  ( 16.25530297147532721, -2.761162301196854685, 315.0000000000000000 ) ) ;
#10165=CARTESIAN_POINT ( 'NONE',  ( -14.57772014836000096, 5.380605385836000565, -314.6383426456000052 ) ) ;
#10166=AXIS2_PLACEMENT_3D ( 'NONE', #3716, #10224, #9415 ) ;
#10168=CARTESIAN_POINT ( 'NONE',  ( -7.221770056846003705, 10.51477558267000667, 319.9928079742500131 ) ) ;
#10173=CARTESIAN_POINT ( 'NONE',  ( 13.97631948628000309, -9.047145764649998867, -317.0792622552969533 ) ) ;
#10177=( BOUNDED_CURVE ( )  B_SPLINE_CURVE ( 3, ( #10516, #3865, #5409, #6320, #4668, #2360, #1330 ),
 .UNSPECIFIED., .F., .F. ) 
 B_SPLINE_CURVE_WITH_KNOTS ( ( 4, 3, 4 ),
 ( 0.000000000000000000, 0.4966743198807560544, 1.000000000000000000 ),
 .UNSPECIFIED. ) 
 CURVE ( )  GEOMETRIC_REPRESENTATION_ITEM ( )  RATIONAL_B_SPLINE_CURVE ( ( 0.9922741236635395090, 0.8025456745203689568, 0.8051209666325224168, 1.000000000000000000, 0.8025111867385940068, 0.8025111867385940068, 1.000000000000000000 ) ) 
 REPRESENTATION_ITEM ( '' )  );
#10179=B_SPLINE_SURFACE_WITH_KNOTS ( 'NONE', 3, 1, ( 
 ( #2640, #5907 ),
 ( #6832, #9356 ),
 ( #5307, #8533 ),
 ( #10260, #2948 ),
 ( #7834, #7781 ),
 ( #2897, #6221 ),
 ( #4408, #6166 ),
 ( #9305, #1991 ),
 ( #1281, #534 ),
 ( #2091, #7096 ),
 ( #1938, #8688 ),
 ( #5358, #6066 ),
 ( #7683, #5259 ) ),
 .UNSPECIFIED., .F., .F., .F.,
 ( 4, 1, 1, 1, 1, 1, 1, 1, 1, 1, 4 ),
 ( 2, 2 ),
 ( 0.01923076923076999858, 0.09935897435896999530, 0.1794871794871999993, 0.2596153846154000133, 0.3397435897436000274, 0.5000000000000000000, 0.6602564102564000281, 0.7403846153845999867, 0.8205128205128000562, 0.9006410256410000148, 0.9807692307692000844 ),
 ( 0.000000000000000000, 1.000000000000000000 ),
 .UNSPECIFIED. ) ;
#10186=CARTESIAN_POINT ( 'NONE',  ( 4.854896540501004054, -12.13415599451999682, 191.1197171614399792 ) ) ;
#10189=CARTESIAN_POINT ( 'NONE',  ( -13.31171245337000819, -8.049428572247000702, -302.5071922382879279 ) ) ;
#10196=CARTESIAN_POINT ( 'NONE',  ( 12.99935040274999487, -9.597679858163006728, 319.5792614743400009 ) ) ;
#10199=CARTESIAN_POINT ( 'NONE',  ( -16.10362618234000109, 3.713712614977999760, 314.6383426456000052 ) ) ;
#10202=CARTESIAN_POINT ( 'NONE',  ( -18.71194885756699477, -4.439033925638975475, 190.9999999999995737 ) ) ;
#10204=CARTESIAN_POINT ( 'NONE',  ( 7.846787046322997838, 11.50147725199999371, 318.8802828394900644 ) ) ;
#10209=CARTESIAN_POINT ( 'NONE',  ( -15.42265167804419512, 3.971230633025111700, 315.0000000000000568 ) ) ;
#10210=CARTESIAN_POINT ( 'NONE',  ( 19.99999999999999289, -7.322330470418032533, 190.9999999999999432 ) ) ;
#10213=CARTESIAN_POINT ( 'NONE',  ( -15.40306756913855679, -3.994766537461137634, -315.0000000000001137 ) ) ;
#10215=ADVANCED_FACE ( 'NONE', ( #2514 ), #1173, .F. ) ;
#10219=CARTESIAN_POINT ( 'NONE',  ( -14.00145308865742422, 5.362717611231083481, -315.0000000000000568 ) ) ;
#10220=CARTESIAN_POINT ( 'NONE',  ( -18.69235161570000159, 1.652152683404002342, 190.0071920248299477 ) ) ;
#10222=CARTESIAN_POINT ( 'NONE',  ( 14.34749558092999777, -7.521529436904000221, -317.5000000000000000 ) ) ;
#10224=DIRECTION ( 'NONE',  ( 0.000000000000000000, 0.000000000000000000, -1.000000000000000000 ) ) ;
#10225=CARTESIAN_POINT ( 'NONE',  ( 13.37739799451331457, -5.841934623551301442, 315.0000000000000000 ) ) ;
#10226=CARTESIAN_POINT ( 'NONE',  ( -10.40890489166000066, 7.434429060800999522, -315.0848619657999734 ) ) ;
#10229=CARTESIAN_POINT ( 'NONE',  ( -14.87701781886999086, 6.977856518223995330, 319.9928079742500131 ) ) ;
#10230=CARTESIAN_POINT ( 'NONE',  ( 6.752884998590677590, -11.77766676623698494, -316.5000000000004547 ) ) ;
#10233=CARTESIAN_POINT ( 'NONE',  ( 10.06352840551000050, 9.619263554820991047, -317.4928077629770087 ) ) ;
#10235=CARTESIAN_POINT ( 'NONE',  ( -18.60752753902997725, -4.785892219302998463, -317.0792622552969533 ) ) ;
#10237=CARTESIAN_POINT ( 'NONE',  ( 12.32755932899228846, 7.043638358068010419, -314.5741798689287521 ) ) ;
#10239=CARTESIAN_POINT ( 'NONE',  ( -7.347903365571999856, -10.60600056872999986, 190.0000000000000000 ) ) ;
#10240=FACE_BOUND ( 'NONE', #6045, .T. ) ;
#10242=CARTESIAN_POINT ( 'NONE',  ( 3.128426543399003279, -12.35671765842998582, 191.1197171614399792 ) ) ;
#10245=FACE_OUTER_BOUND ( 'NONE', #2458, .T. ) ;
#10247=( BOUNDED_SURFACE ( )  B_SPLINE_SURFACE ( 3, 1, ( 
 ( #7734, #3650 ),
 ( #9506, #10210 ),
 ( #3603, #2848 ),
 ( #6117, #2147 ),
 ( #10153, #8483 ),
 ( #9405, #5411 ),
 ( #10361, #3003 ) ),
 .UNSPECIFIED., .F., .F., .F. ) 
 B_SPLINE_SURFACE_WITH_KNOTS ( ( 4, 3, 4 ),
 ( 2, 2 ),
 ( 0.000000000000000000, 0.5000000000000000000, 1.000000000000000000 ),
 ( 0.000000000000000000, 1.000000000000000000 ),
 .UNSPECIFIED. ) 
 GEOMETRIC_REPRESENTATION_ITEM ( )  RATIONAL_B_SPLINE_SURFACE ( (
 ( 1.000000000000000000, 1.000000000000000000),
 ( 0.8047378541210479241, 0.8047378541210479241),
 ( 0.8047378541210479241, 0.8047378541210479241),
 ( 1.000000000000000000, 1.000000000000000000),
 ( 0.8047378541210479241, 0.8047378541210479241),
 ( 0.8047378541210479241, 0.8047378541210479241),
 ( 1.000000000000000000, 1.000000000000000000) ) ) 
 REPRESENTATION_ITEM ( '' )  SURFACE ( )  );
#10249=CARTESIAN_POINT ( 'NONE',  ( -18.29625743176001862, 2.888693746018001107, -302.5071922382879279 ) ) ;
#10250=CARTESIAN_POINT ( 'NONE',  ( 13.92742316895000165, -9.072312068102004190, 319.5792614743400009 ) ) ;
#10251=CARTESIAN_POINT ( 'NONE',  ( 15.74033075358999945, -3.452242816619000010, -315.0848619657999734 ) ) ;
#10252=CARTESIAN_POINT ( 'NONE',  ( -17.21448334449999962, 1.351716521078000222, 314.6383426456000052 ) ) ;
#10254=CARTESIAN_POINT ( 'NONE',  ( -10.60393767981000757, -9.400660304482000740, 190.0071920248299477 ) ) ;
#10256=CARTESIAN_POINT ( 'NONE',  ( -15.00000000000325961, -7.547804830080786473E-15, 315.0000000000001705 ) ) ;
#10259=CARTESIAN_POINT ( 'NONE',  ( -16.31058353111865955, 2.657800654349994129, 315.0000000000000000 ) ) ;
#10260=CARTESIAN_POINT ( 'NONE',  ( -13.57573464316000056, -3.225916527208000151, -284.9999999999999432 ) ) ;
#10261=CARTESIAN_POINT ( 'NONE',  ( -11.74249363970098514, -6.849480045866886080, -315.0000000000000568 ) ) ;
#10264=DIRECTION ( 'NONE',  ( 0.000000000000000000, 0.000000000000000000, 1.000000000000000000 ) ) ;
#10265=( BOUNDED_CURVE ( )  B_SPLINE_CURVE ( 3, ( #3099, #4721, #4928, #741, #2298, #10513, #8792, #8042, #2357, #1434, #3046, #6542, #6375, #842, #690, #8205, #7138, #3962, #7189, #6432, #7997, #9715, #5567, #7242, #4827, #8904, #8098, #8155, #9658, #4017, #635, #793, #10406, #3910, #10458, #6316, #10622, #9602, #7299, #8853, #10572, #1495, #3214, #6490, #4773, #9768, #3264, #2406 ),
 .UNSPECIFIED., .F., .F. ) 
 B_SPLINE_CURVE_WITH_KNOTS ( ( 4, 1, 1, 1, 1, 1, 1, 1, 1, 1, 1, 1, 1, 1, 1, 1, 1, 1, 1, 1, 1, 1, 1, 1, 1, 1, 1, 1, 1, 1, 1, 1, 1, 1, 1, 1, 1, 1, 1, 1, 1, 1, 1, 1, 1, 4 ),
 ( 0.000000000000000000, 0.01773478386796039155, 0.03606240600880905589, 0.05363178075044054693, 0.07078725724691502241, 0.08782600590454303635, 0.1049244321358658166, 0.1219539535917407574, 0.1389477140559595703, 0.1563980977818864582, 0.1746363666666239378, 0.1934786392176560677, 0.2128025958997292744, 0.2327904454208181428, 0.2535195744865268441, 0.2747166135707194701, 0.2963888843556194419, 0.3192629785013852417, 0.3441555232881245430, 0.3718650194528611563, 0.4028399612510202843, 0.4371448801345994006, 0.4747436484650955357, 0.5142463203427463103, 0.5531490499891782431, 0.5894092591003674553, 0.6223615841373307811, 0.6515869223714267910, 0.6772431252474824248, 0.7004011076752997278, 0.7222184512862190875, 0.7437909259358911340, 0.7652154438741728404, 0.7858628007620030997, 0.8056883297028466506, 0.8249734464625099184, 0.8436696960199339124, 0.8615821821759899191, 0.8789123401951888237, 0.8960241576542978814, 0.9130500659135323271, 0.9300436868742999463, 0.9471989324631474583, 0.9647777872405101096, 0.9830893744542017476, 1.000000000000000000 ),
 .UNSPECIFIED. ) 
 CURVE ( )  GEOMETRIC_REPRESENTATION_ITEM ( )  RATIONAL_B_SPLINE_CURVE ( ( 1.171573003563729509, 1.171573003563729509, 1.171573003563729509, 1.171573003563729509, 1.171573003563729509, 1.171573003563729509, 1.171573003563729509, 1.171573003563729509, 1.171573003563729509, 1.171573003563729509, 1.171573003563729509, 1.171573003563729509, 1.171573003563729509, 1.171573003563729509, 1.171573003563729509, 1.171573003563729509, 1.171573003563729509, 1.171573003563729509, 1.171573003563729509, 1.171573003563729509, 1.171573003563729509, 1.171573003563729509, 1.171573003563729509, 1.171573003563729509, 1.171573003563729509, 1.171573003563729509, 1.171573003563729509, 1.171573003563729509, 1.171573003563729509, 1.171573003563729509, 1.171573003563729509, 1.171573003563729509, 1.171573003563729509, 1.171573003563729509, 1.171573003563729509, 1.171573003563729509, 1.171573003563729509, 1.171573003563729509, 1.171573003563729509, 1.171573003563729509, 1.171573003563729509, 1.171573003563729509, 1.171573003563729509, 1.171573003563729509, 1.171573003563729509, 1.171573003563729509, 1.171573003563729509, 1.171573003563729731 ) ) 
 REPRESENTATION_ITEM ( '' )  );
#10266=CARTESIAN_POINT ( 'NONE',  ( -11.84501012641003825, 6.794057347756047527, -315.0000000000000000 ) ) ;
#10267=CARTESIAN_POINT ( 'NONE',  ( -18.44574565965998758, 2.441956922350000614, 190.0071920248299477 ) ) ;
#10275=CARTESIAN_POINT ( 'NONE',  ( 8.647614135908284538, -8.167456227882626152, 315.0000000000000568 ) ) ;
#10276=CARTESIAN_POINT ( 'NONE',  ( -10.58688533405000065, 7.844683714540999553, -314.6383426456000052 ) ) ;
#10280=ORIENTED_EDGE ( 'NONE', *, *, #3332, .F. ) ;
#10281=CARTESIAN_POINT ( 'NONE',  ( -3.713744197507001576, 11.87335072286999527, -317.5770954168139610 ) ) ;
#10282=CARTESIAN_POINT ( 'NONE',  ( -12.84330733966000437, -9.683159015349998455, -317.0792622552969533 ) ) ;
#10283=CARTESIAN_POINT ( 'NONE',  ( -8.037373804805000077, -9.179324345868998591, -315.0000000000000000 ) ) ;
#10285=CARTESIAN_POINT ( 'NONE',  ( -1.822666172895162529, 9.956379168149535275, -314.5031572587578239 ) ) ;
#10287=CARTESIAN_POINT ( 'NONE',  ( -11.56195786956000049, -9.110631795823000090, 190.0000000000000000 ) ) ;
#10288=CIRCLE ( 'NONE', #3604, 0.9999999999999755751 ) ;
#10291=ORIENTED_EDGE ( 'NONE', *, *, #6882, .T. ) ;
#10292=CARTESIAN_POINT ( 'NONE',  ( -19.50564046359999537, -2.789525877152000621, 191.1197171614399792 ) ) ;
#10293=ORIENTED_EDGE ( 'NONE', *, *, #4443, .F. ) ;
#10294=CARTESIAN_POINT ( 'NONE',  ( -16.24439548573774417, -2.790585206482182556, 315.0000000000000000 ) ) ;
#10295=CARTESIAN_POINT ( 'NONE',  ( 14.33246323392999422, -7.385748264902002092, -302.5071922382879279 ) ) ;
#10297=CARTESIAN_POINT ( 'NONE',  ( 8.833609186824004311, 11.21733050393000575, 191.1197171614399792 ) ) ;
#10300=CARTESIAN_POINT ( 'NONE',  ( -18.90089112233000179, 0.2930644900430999789, -302.5071922382879279 ) ) ;
#10301=CARTESIAN_POINT ( 'NONE',  ( -17.10170768143997932, -6.605950023609995725, 319.5792614743400009 ) ) ;
#10302=CARTESIAN_POINT ( 'NONE',  ( 17.57673583306999632, 0.3313182897943000582, -314.4150829855000211 ) ) ;
#10303=CARTESIAN_POINT ( 'NONE',  ( -17.56758064089999749, 0.6313722887073999201, 314.4150829855000211 ) ) ;
#10305=CARTESIAN_POINT ( 'NONE',  ( 18.12330621507001638, -3.185864752952001222, 190.0071920248299477 ) ) ;
#10311=CARTESIAN_POINT ( 'NONE',  ( -14.25090727152774228, 5.161646102170217354, 315.0000000000000568 ) ) ;
#10312=CARTESIAN_POINT ( 'NONE',  ( -13.89455516181870642, -5.448669939092228631, -314.9999999999999432 ) ) ;
#10315=CARTESIAN_POINT ( 'NONE',  ( 8.616488358140820480, 8.177789738293624211, -315.0000000000000000 ) ) ;
#10316=CARTESIAN_POINT ( 'NONE',  ( 18.86321946521001180, -0.4765678057151002123, 190.0071920248299477 ) ) ;
#10317=CARTESIAN_POINT ( 'NONE',  ( -17.50000000000001776, 8.653894624238266756E-10, -302.5000000000001137 ) ) ;
#10319=CARTESIAN_POINT ( 'NONE',  ( 18.32558628770999931, -3.116746082530000184, -317.4999999999870397 ) ) ;
#10321=CARTESIAN_POINT ( 'NONE',  ( 8.586872910504615319, -8.187582572610192955, 315.0000000000000568 ) ) ;
#10322=CARTESIAN_POINT ( 'NONE',  ( -3.971626792229000280, 9.186906450543000702, -315.0848619657999734 ) ) ;
#10323=CARTESIAN_POINT ( 'NONE',  ( -12.89405912172824920, -6.798013172113485325, 314.4999472004059839 ) ) ;
#10325=CARTESIAN_POINT ( 'NONE',  ( 19.59064078059999758, 0.07061976926606000626, 320.0770942683900557 ) ) ;
#10329=CARTESIAN_POINT ( 'NONE',  ( 7.757100520214003758, 11.09835178152000168, -317.5770954168139610 ) ) ;
#10330=CARTESIAN_POINT ( 'NONE',  ( -10.49155472272000011, -10.73755170802999714, -317.0792622552969533 ) ) ;
#10335=CARTESIAN_POINT ( 'NONE',  ( 17.03769437857128821, 2.221013643562902651, -314.5274634404338485 ) ) ;
#10339=CARTESIAN_POINT ( 'NONE',  ( 16.30951479290585482, -7.248637510199255729, 319.0000000000003979 ) ) ;
#10343=CARTESIAN_POINT ( 'NONE',  ( -16.45391189178886293, -2.370722300009959760, 315.0000000000001705 ) ) ;
#10344=CARTESIAN_POINT ( 'NONE',  ( -9.183684135703998663, -10.67340332910999834, -302.4229045757450081 ) ) ;
#10345=CARTESIAN_POINT ( 'NONE',  ( 14.79481407445002183, 8.414248563823001348, 191.1197171614399792 ) ) ;
#10350=CARTESIAN_POINT ( 'NONE',  ( -16.10169247195999631, 5.923112460043001626, -302.5071922382879279 ) ) ;
#10352=CARTESIAN_POINT ( 'NONE',  ( 10.67587555525000020, -8.049811041411000900, -314.4150829855000211 ) ) ;
#10353=CARTESIAN_POINT ( 'NONE',  ( -16.90798586812000082, -0.2930809059028999797, 315.0848619657999734 ) ) ;
#10360=CARTESIAN_POINT ( 'NONE',  ( -16.99965680672947954, 0.4176726732850534751, 314.9999999999998863 ) ) ;
#10361=CARTESIAN_POINT ( 'NONE',  ( -20.00000000000000000, 3.518725546161979705E-10, 319.0000000000000000 ) ) ;
#10362=CARTESIAN_POINT ( 'NONE',  ( -16.99910511164433302, -0.8673928700097519595, -315.0000000000000000 ) ) ;
#10363=FACE_OUTER_BOUND ( 'NONE', #7992, .T. ) ;
#10364=CARTESIAN_POINT ( 'NONE',  ( 17.50000000000002487, 1.995060298004523415E-08, 314.4999385900306947 ) ) ;
#10367=CARTESIAN_POINT ( 'NONE',  ( -11.80659750965543608, 6.814906413124091955, -314.9999999999999432 ) ) ;
#10368=CARTESIAN_POINT ( 'NONE',  ( -6.317945743273003956, 11.44290306353000730, 189.9229057364800042 ) ) ;
#10369=CARTESIAN_POINT ( 'NONE',  ( 3.206494179919505694, 9.870881073625612956, 314.4999451744448606 ) ) ;
#10370=CARTESIAN_POINT ( 'NONE',  ( -7.617198281494000689, -10.53565010756000042, -317.5000000000000000 ) ) ;
#10375=CARTESIAN_POINT ( 'NONE',  ( 15.63365740121746406, -3.715179591933191361, 315.0000000000000568 ) ) ;
#10376=CARTESIAN_POINT ( 'NONE',  ( 8.450675645183000739, 8.177559542660000957, -315.0848619657999734 ) ) ;
#10377=CARTESIAN_POINT ( 'NONE',  ( -8.203499201192052226, -8.842483654835438855, 314.4999460608030404 ) ) ;
#10378=CARTESIAN_POINT ( 'NONE',  ( -19.10207382662997588, 2.686351016941002534, 320.0770942683900557 ) ) ;
#10382=CARTESIAN_POINT ( 'NONE',  ( -19.39427072114999717, 3.381181012882998882, -317.0792622552969533 ) ) ;
#10383=CARTESIAN_POINT ( 'NONE',  ( -13.88920775975001298, -9.001345760802989204, -316.3802825947000201 ) ) ;
#10386=EDGE_LOOP ( 'NONE', ( #9220, #3378, #6158, #3386, #3584 ) ) ;
#10388=CARTESIAN_POINT ( 'NONE',  ( -17.44177680037102007, -0.9115828329868908009, -314.5029970719331232 ) ) ;
#10391=CARTESIAN_POINT ( 'NONE',  ( -0.2363647329299939648, 12.51727884664820856, -316.5000000000004547 ) ) ;
#10392=VERTEX_POINT ( 'NONE', #6257 ) ;
#10393=CARTESIAN_POINT ( 'NONE',  ( -3.689342025446077589, -9.275861061134104801, 315.0000000000001137 ) ) ;
#10394=CARTESIAN_POINT ( 'NONE',  ( -15.97017057534000450, -7.646575558462997080, -302.9207377450070453 ) ) ;
#10395=CARTESIAN_POINT ( 'NONE',  ( 15.59929043073998578, 7.826471063572999931, 191.1197171614399792 ) ) ;
#10398=CARTESIAN_POINT ( 'NONE',  ( 11.73636226353998779, 10.21860227534999943, -302.9207377450070453 ) ) ;
#10399=CARTESIAN_POINT ( 'NONE',  ( -10.00000000000000000, -2.500000000000000000, -285.0000000000000000 ) ) ;
#10401=CARTESIAN_POINT ( 'NONE',  ( -10.50000150490000017, -7.882579085736000302, -314.6383426456000052 ) ) ;
#10402=B_SPLINE_CURVE_WITH_KNOTS ( 'NONE', 3,
 ( #6396, #9786, #6616, #4842, #9674, #5747, #4892, #7261, #4943, #8173, #10531, #3929, #9032, #7209, #5586, #4740, #8870, #6450, #2424, #4, #806, #5692, #2529, #753, #1512, #8218, #4089, #9731, #858, #3279, #4037, #10475, #8810, #1459, #7316, #8011, #654, #5962, #9199, #5205, #325, #9997, #8482, #3602, #9304, #5797, #6778, #7628, #1834, #6666, #1124, #273, #2693, #9254, #1883, #3551, #6831, #2584, #9086, #9942, #3498, #1724, #4407, #5046, #10152, #2638, #6885, #5905, #5155, #5101, #8428, #116, #1070, #4355, #7682, #8380, #1015, #10101, #2743, #4304, #220, #6011, #8272, #3391, #10052, #7574, #5847, #9138, #1937, #4993, #8329, #1776, #909, #4198, #7473, #967, #4252, #7523, #166, #3443, #6721, #586, #2947, #7833, #4454, #4559, #10311, #6933, #4669, #3866, #1280, #6220, #10209, #4611, #9556, #7733, #375, #5257, #6065, #10259, #8532, #424, #3702, #7143, #482, #3750, #2195, #8635, #2847, #5410, #6276, #10360, #2895 ),
 .UNSPECIFIED., .F., .F.,
 ( 4, 1, 1, 1, 1, 1, 2, 2, 1, 1, 1, 1, 1, 2, 2, 1, 1, 1, 1, 1, 2, 2, 1, 1, 1, 1, 1, 2, 2, 1, 1, 1, 1, 1, 1, 2, 2, 1, 1, 1, 1, 1, 2, 2, 1, 1, 2, 2, 2, 1, 1, 2, 2, 1, 1, 1, 1, 2, 2, 1, 1, 1, 1, 1, 1, 2, 2, 1, 1, 1, 1, 1, 2, 2, 1, 1, 1, 1, 1, 2, 2, 1, 1, 1, 1, 1, 2, 2, 1, 1, 1, 1, 2, 2, 1, 1, 1, 2, 2, 4 ),
 ( 0.000000000000000000, 0.06250000000000791034, 0.09375000000001181000, 0.1093750000000137529, 0.1171875000000147105, 0.1210937500000152794, 0.1230468750000155709, 0.1250000000000158484, 0.1562500000000223432, 0.1718750000000255906, 0.1796875000000270617, 0.1835937500000277833, 0.1855468750000281719, 0.1865234375000283107, 0.1875000000000284217, 0.2187500000000311418, 0.2343750000000323908, 0.2421875000000330014, 0.2460937500000334177, 0.2480468750000336398, 0.2490234375000336953, 0.2500000000000337508, 0.2812500000000370259, 0.2968750000000386358, 0.3046875000000394684, 0.3085937500000398570, 0.3105468750000400235, 0.3115234375000401346, 0.3125000000000403011, 0.3437500000000445199, 0.3593750000000465739, 0.3671875000000476286, 0.3710937500000481282, 0.3730468750000484057, 0.3740234375000484612, 0.3745117187500484612, 0.3750000000000484612, 0.4062500000000490163, 0.4218750000000493494, 0.4296875000000495159, 0.4335937500000495715, 0.4355468750000495715, 0.4365234375000495715, 0.4375000000000495715, 0.4531250000000494604, 0.4609375000000494049, 0.4648437500000494049, 0.4687500000000494049, 0.5000000000000491829, 0.5156250000000491829, 0.5234375000000491829, 0.5273437500000490719, 0.5312500000000490719, 0.5468750000000488498, 0.5546875000000488498, 0.5585937500000488498, 0.5605468750000488498, 0.5615234375000488498, 0.5625000000000488498, 0.5937500000000481837, 0.6093750000000478506, 0.6171875000000476286, 0.6210937500000475175, 0.6230468750000474065, 0.6240234375000474065, 0.6245117187500474065, 0.6250000000000472955, 0.6562500000000430767, 0.6718750000000409672, 0.6796875000000398570, 0.6835937500000393019, 0.6855468750000390799, 0.6865234375000389688, 0.6875000000000388578, 0.7187500000000363043, 0.7343750000000350830, 0.7421875000000345279, 0.7460937500000343059, 0.7480468750000340838, 0.7490234375000340838, 0.7500000000000340838, 0.7812500000000317524, 0.7968750000000304201, 0.8046875000000298650, 0.8085937500000295319, 0.8105468750000293099, 0.8115234375000293099, 0.8125000000000293099, 0.8437500000000242029, 0.8593750000000216493, 0.8671875000000203171, 0.8710937500000196509, 0.8730468750000193179, 0.8750000000000189848, 0.9062500000000143219, 0.9218750000000121014, 0.9296875000000109912, 0.9335937500000103251, 0.9375000000000097700, 1.000000000000000000 ),
 .UNSPECIFIED. ) ;
#10405=CARTESIAN_POINT ( 'NONE',  ( -19.38229133873998222, -1.780473529460998128, 189.9229057364800042 ) ) ;
#10406=CARTESIAN_POINT ( 'NONE',  ( 12.04241988217490622, 9.990194130379512316, 190.9999999999996589 ) ) ;
#10407=CARTESIAN_POINT ( 'NONE',  ( -15.00000000000325961, -7.547804830080786473E-15, -284.9999999999999432 ) ) ;
#10409=CARTESIAN_POINT ( 'NONE',  ( -16.98808798087999961, -1.334629195702000004, 314.8616023057000461 ) ) ;
#10412=CARTESIAN_POINT ( 'NONE',  ( -8.736690731312993563, -10.08117623986000133, 319.9928079742500131 ) ) ;
#10413=CARTESIAN_POINT ( 'NONE',  ( -2.737481088004029228, -9.377302004685557080, -315.0000000000000000 ) ) ;
#10418=CARTESIAN_POINT ( 'NONE',  ( 4.298300662841374020, 9.188610398197571527, -315.0000000000000568 ) ) ;
#10420=CARTESIAN_POINT ( 'NONE',  ( -7.675832365144997560, 11.11882312068000189, 189.9229057364800042 ) ) ;
#10421=CARTESIAN_POINT ( 'NONE',  ( 17.50000000088856567, 5.867334121986925055, -302.4999999999996589 ) ) ;
#10424=CARTESIAN_POINT ( 'NONE',  ( 3.131429216827940247E-09, -12.50000000000000000, -316.5000000000000000 ) ) ;
#10427=CARTESIAN_POINT ( 'NONE',  ( -17.71378747801018960, -5.838323448755803113, -303.5000000000006253 ) ) ;
#10429=CARTESIAN_POINT ( 'NONE',  ( -3.214697847761800006E-15, 10.00000000000000000, 315.0000000000000000 ) ) ;
#10430=CARTESIAN_POINT ( 'NONE',  ( 18.77022956583000735, 3.456581952569002247, 320.0770942683900557 ) ) ;
#10434=CARTESIAN_POINT ( 'NONE',  ( -5.251781279335003383, 11.64703610505998910, -317.5770954168139610 ) ) ;
#10435=CARTESIAN_POINT ( 'NONE',  ( -6.467159262072997628, -11.83367582535999141, -316.3802825947000201 ) ) ;
#10436=EDGE_CURVE ( 'NONE', #9806, #1376, #727, .T. ) ;
#10439=CARTESIAN_POINT ( 'NONE',  ( -17.04726327197863256, 2.225800558269679819, -314.5277276635413273 ) ) ;
#10441=CARTESIAN_POINT ( 'NONE',  ( -15.84843729815538538, -4.154783985720819750, -314.5664249374442534 ) ) ;
#10442=ORIENTED_EDGE ( 'NONE', *, *, #9636, .F. ) ;
#10443=CARTESIAN_POINT ( 'NONE',  ( -14.97237716209997416, 8.305886502593784471, -316.5000000000004547 ) ) ;
#10445=CARTESIAN_POINT ( 'NONE',  ( -11.28384026436728327, -7.096146896414363248, 315.0000000000000000 ) ) ;
#10446=CARTESIAN_POINT ( 'NONE',  ( -7.921361508960999664, -11.05315760980000661, -302.4229045757450081 ) ) ;
#10451=CARTESIAN_POINT ( 'NONE',  ( 14.68756396110000395, 7.991310926523999214, -302.4229045757450081 ) ) ;
#10452=CARTESIAN_POINT ( 'NONE',  ( 19.49027688392999735, -2.831154404542999714, 318.8802828394900644 ) ) ;
#10454=CARTESIAN_POINT ( 'NONE',  ( -3.846123575835999731, -9.203727088275000412, -315.0848619657999734 ) ) ;
#10455=CARTESIAN_POINT ( 'NONE',  ( 13.34617449956999913, 8.168334506422000985, -302.5000000000000000 ) ) ;
#10457=CARTESIAN_POINT ( 'NONE',  ( 15.36042613538998758, -7.487426557894995227, 189.9229057364800042 ) ) ;
#10458=CARTESIAN_POINT ( 'NONE',  ( 13.93599793909949547, 8.976999749472311052, 190.9999999999996589 ) ) ;
#10461=ORIENTED_EDGE ( 'NONE', *, *, #10623, .F. ) ;
#10463=CARTESIAN_POINT ( 'NONE',  ( -12.10743226551000085, -7.094093637544000686, 314.6383426456000052 ) ) ;
#10465=CARTESIAN_POINT ( 'NONE',  ( -13.45825946928999706, -7.955479052880997770, 319.9928079742500131 ) ) ;
#10467=CARTESIAN_POINT ( 'NONE',  ( -11.98824862436842587, 10.01561519341996487, 319.0000000000005116 ) ) ;
#10470=ORIENTED_EDGE ( 'NONE', *, *, #4895, .F. ) ;
#10472=CARTESIAN_POINT ( 'NONE',  ( 18.76999596014998772, 3.457077136807001683, 189.9229057364800042 ) ) ;
#10473=CARTESIAN_POINT ( 'NONE',  ( 7.551285798577536568, 9.031218586147737426, 314.4999459341804595 ) ) ;
#10475=CARTESIAN_POINT ( 'NONE',  ( 12.11102551177084941, 6.646503028198875285, 314.9999999999999432 ) ) ;
#10477=CARTESIAN_POINT ( 'NONE',  ( -14.92864611359687999, -8.336576156742355082, -303.4999999999996589 ) ) ;
#10478=CARTESIAN_POINT ( 'NONE',  ( 17.56330558013000243, 0.6698376231023999150, -314.4150829855000211 ) ) ;
#10482=CARTESIAN_POINT ( 'NONE',  ( -0.6255878334489998194, 12.09339422449000168, 320.0770942683900557 ) ) ;
#10485=VERTEX_POINT ( 'NONE', #307 ) ;
#10486=CARTESIAN_POINT ( 'NONE',  ( 18.90056365643000547, 0.3167749459464000994, -317.4928077629770087 ) ) ;
#10487=CARTESIAN_POINT ( 'NONE',  ( -19.29920617650999404, -3.385971943253997640, -316.3802825947000201 ) ) ;
#10488=ORIENTED_EDGE ( 'NONE', *, *, #9836, .F. ) ;
#10489=CARTESIAN_POINT ( 'NONE',  ( 11.54587391409000041, -9.118162486329000060, 320.0000000000000000 ) ) ;
#10490=FACE_BOUND ( 'NONE', #8942, .T. ) ;
#10493=CARTESIAN_POINT ( 'NONE',  ( 12.96318846091384991, -9.529552999724860030, 319.0000000000003979 ) ) ;
#10494=EDGE_CURVE ( 'NONE', #9531, #9273, #811, .T. ) ;
#10498=CARTESIAN_POINT ( 'NONE',  ( -4.252796533868254514, -9.197585063050969012, 315.0000000000000568 ) ) ;
#10499=CARTESIAN_POINT ( 'NONE',  ( -10.56785312427999735, -10.70734743398999811, -302.9207377450070453 ) ) ;
#10500=B_SPLINE_CURVE_WITH_KNOTS ( 'NONE', 3,
 ( #1997, #4411, #10107, #2749, #6018, #7687, #1132, #6729, #2592, #175, #9260, #5854, #331, #6891, #10157, #5968, #1025, #1839, #4260, #5107, #228, #7530 ),
 .UNSPECIFIED., .F., .F.,
 ( 4, 2, 2, 2, 2, 2, 2, 2, 2, 2, 4 ),
 ( 0.4999983592357296613, 0.5624985643312634398, 0.5937486668790303845, 0.6249987694267972183, 0.6562488719745640520, 0.6874989745223309967, 0.7499991796178647752, 0.8124993847133985536, 0.8749995898089324431, 0.9374997949044662215, 1.000000000000000000 ),
 .UNSPECIFIED. ) ;
#10503=CARTESIAN_POINT ( 'NONE',  ( 0.000000000000000000, -10.00000000000000000, 315.0000000000000000 ) ) ;
#10504=( LENGTH_UNIT ( ) NAMED_UNIT ( * ) SI_UNIT ( .MILLI., .METRE. ) );
#10505=CARTESIAN_POINT ( 'NONE',  ( -9.278531818924999897, 11.16715007748999078, -302.9207377450070453 ) ) ;
#10506=CARTESIAN_POINT ( 'NONE',  ( 18.17597206675998223, -5.223702392620001689, 318.8802828394900644 ) ) ;
#10508=CARTESIAN_POINT ( 'NONE',  ( -3.903842856253999738, -9.647088721075000706, -314.6383426456000052 ) ) ;
#10509=CARTESIAN_POINT ( 'NONE',  ( -17.50000000000000000, 0.000000000000000000, -302.5000000000000000 ) ) ;
#10512=CARTESIAN_POINT ( 'NONE',  ( -18.76999596014998772, -3.457077136807001683, 189.9229057364800042 ) ) ;
#10513=CARTESIAN_POINT ( 'NONE',  ( -19.12881201168725198, 3.682481340332639519, 190.9999999999996589 ) ) ;
#10515=CARTESIAN_POINT ( 'NONE',  ( -15.89383674730000173, -3.622219875512000087, 314.8616023057000461 ) ) ;
#10516=CARTESIAN_POINT ( 'NONE',  ( 0.000000000000000000, -10.00000000000000178, 315.0000000000000000 ) ) ;
#10519=CARTESIAN_POINT ( 'NONE',  ( -13.88765719697804712, 9.006220412848993107, 319.0000000000005116 ) ) ;
#10521=CARTESIAN_POINT ( 'NONE',  ( -13.57573464316000056, 3.225916527208000151, 315.0000000000000000 ) ) ;
#10526=CARTESIAN_POINT ( 'NONE',  ( 8.712128322568002403, 10.82186910204999997, 189.9229057364800042 ) ) ;
#10531=CARTESIAN_POINT ( 'NONE',  ( 16.24439548573774417, 2.790585206482182556, 315.0000000000000000 ) ) ;
#10534=CARTESIAN_POINT ( 'NONE',  ( 16.88587703871184331, -6.724495681871323072, -303.4999999999996589 ) ) ;
#10536=CARTESIAN_POINT ( 'NONE',  ( 17.16710485141000220, 2.239552065056999997, -314.4150829855000211 ) ) ;
#10537=CARTESIAN_POINT ( 'NONE',  ( 15.00000000000000000, 0.000000000000000000, -285.0000000000000000 ) ) ;
#10539=CARTESIAN_POINT ( 'NONE',  ( -16.20020866270998638, 5.814836367836996978, 319.9928079742500131 ) ) ;
#10542=CARTESIAN_POINT ( 'NONE',  ( 12.80442074722001067, 9.608322671940996429, -316.3802825947000201 ) ) ;
#10543=CARTESIAN_POINT ( 'NONE',  ( 6.751314262718001835, -11.77064546103999731, -316.3802825947000201 ) ) ;
#10548=CARTESIAN_POINT ( 'NONE',  ( 12.48775874806000097, -8.649334263351001084, 320.0000000000000000 ) ) ;
#10555=ORIENTED_EDGE ( 'NONE', *, *, #3332, .T. ) ;
#10556=CARTESIAN_POINT ( 'NONE',  ( -14.55942669488979391, -5.453671309400836442, -314.5801547934445352 ) ) ;
#10560=CARTESIAN_POINT ( 'NONE',  ( -2.545396798794703042, -9.391972178232515844, 315.0000000000000568 ) ) ;
#10561=CARTESIAN_POINT ( 'NONE',  ( -3.644643686525998572, -11.88155656384000203, -302.4229045757450081 ) ) ;
#10562=FACE_OUTER_BOUND ( 'NONE', #7570, .T. ) ;
#10565=CARTESIAN_POINT ( 'NONE',  ( 12.62193639354000396, 9.236300292413996971, -302.4229045757450081 ) ) ;
#10566=CARTESIAN_POINT ( 'NONE',  ( 9.526067998327799539E-10, -10.00000000005854339, 314.4999528359535361 ) ) ;
#10568=CARTESIAN_POINT ( 'NONE',  ( 12.07130791617000121, -6.858215270785999351, -314.8616023057000461 ) ) ;
#10569=CARTESIAN_POINT ( 'NONE',  ( 19.99999036626000048, 4.642009117057000143E-09, -316.5000000000000000 ) ) ;
#10571=CARTESIAN_POINT ( 'NONE',  ( -18.70165185342001735, -1.614428960665998503, 190.0071920248299477 ) ) ;
#10572=CARTESIAN_POINT ( 'NONE',  ( 18.21004088691051948, 5.189404274100754222, 190.9999999999996589 ) ) ;
#10575=CARTESIAN_POINT ( 'NONE',  ( 1.419551022038999966, -10.09154694854999867, 314.4150829855000211 ) ) ;
#10576=CARTESIAN_POINT ( 'NONE',  ( 7.608551686289999338, 10.53686309807999955, 320.0000000000000000 ) ) ;
#10578=CARTESIAN_POINT ( 'NONE',  ( 16.38421488526942582, 7.181844560322187654, 319.0000000000005116 ) ) ;
#10583=ORIENTED_EDGE ( 'NONE', *, *, #2143, .T. ) ;
#10584=CARTESIAN_POINT ( 'NONE',  ( 19.99999036626000048, 4.642009117057000143E-09, -316.5000000000000000 ) ) ;
#10585=( BOUNDED_CURVE ( )  B_SPLINE_CURVE ( 3, ( #7417, #3335, #3177, #3978 ),
 .UNSPECIFIED., .F., .F. ) 
 B_SPLINE_CURVE_WITH_KNOTS ( ( 4, 4 ),
 ( 0.000000000000000000, 1.000000000000000000 ),
 .UNSPECIFIED. ) 
 CURVE ( )  GEOMETRIC_REPRESENTATION_ITEM ( )  RATIONAL_B_SPLINE_CURVE ( ( 1.171566417337508881, 0.9428088753384672449, 0.9428111942444036275, 1.171573374055317807 ) ) 
 REPRESENTATION_ITEM ( '' )  );
#10588=CARTESIAN_POINT ( 'NONE',  ( 1.674130924758677086, -12.47364919270561856, -303.4999999999996589 ) ) ;
#10589=CARTESIAN_POINT ( 'NONE',  ( 15.39920013370999996, 4.579805981517999669, -314.6383426456000052 ) ) ;
#10592=CARTESIAN_POINT ( 'NONE',  ( 19.14248421182001891, 3.638193899013998145, 318.8802828394900644 ) ) ;
#10596=CARTESIAN_POINT ( 'NONE',  ( 17.77555462084998794, 5.884850558328997394, -317.0792622552969533 ) ) ;
#10597=CARTESIAN_POINT ( 'NONE',  ( 5.321980890543003717, -12.05475797716000486, -316.3802825947000201 ) ) ;
#10601=DIRECTION ( 'NONE',  ( 2.716996281204025196E-06, -0.9999999999963090636, 3.949787424940705384E-23 ) ) ;
#10602=CARTESIAN_POINT ( 'NONE',  ( 4.780493465650555329, -9.113006550021841790, -315.0000000000000568 ) ) ;
#10604=CARTESIAN_POINT ( 'NONE',  ( 17.50000000000125056, 1.338989683019597976E-14, -315.0000000000000568 ) ) ;
#10606=CARTESIAN_POINT ( 'NONE',  ( 8.891587890486999157, 10.15986303230000054, -317.5000000000000000 ) ) ;
#10608=CARTESIAN_POINT ( 'NONE',  ( 20.05676974677001922, 0.5613724988767001545, -302.9207377450070453 ) ) ;
#10614=CARTESIAN_POINT ( 'NONE',  ( -11.54867409098999964, 9.757628671089998207, -302.4229045757450081 ) ) ;
#10615=LINE ( 'NONE', #1699, #1721 ) ;
#10620=ORIENTED_EDGE ( 'NONE', *, *, #8488, .F. ) ;
#10621=CARTESIAN_POINT ( 'NONE',  ( -17.32898823752001860, -5.623515075799002894, 189.9229057364800042 ) ) ;
#10622=CARTESIAN_POINT ( 'NONE',  ( 15.60370682163541289, 7.832153051853420145, 190.9999999999996589 ) ) ;
#10623=EDGE_CURVE ( 'NONE', #4592, #1010, #10177, .T. ) ;
ENDSEC;
END-ISO-10303-21;
